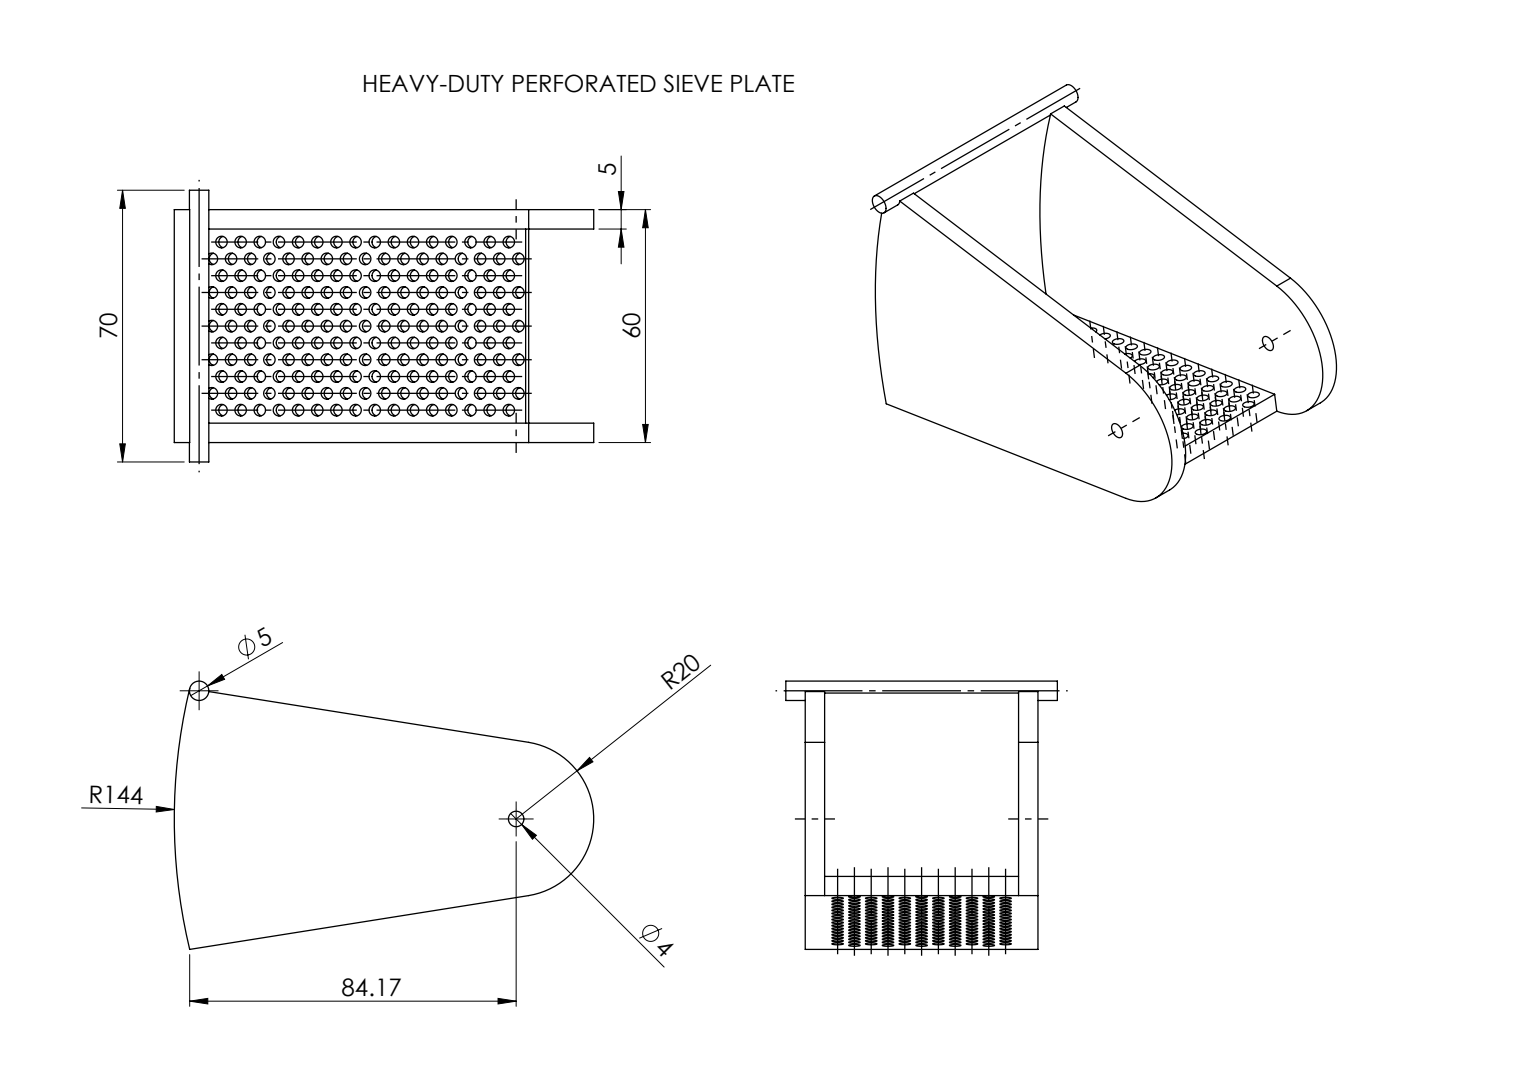
ISO-10303-21;
HEADER;
FILE_DESCRIPTION (('STEP AP214'),
    '1' );
FILE_NAME ('Heavy-Duty Perforated Sieve Plate.step',
    '2026-10-02T13:02:33',
    ( '' ),
    ( '' ),
    'SwSTEP 2.0',
    'SolidWorks 2026',
    '' );
FILE_SCHEMA (( 'AUTOMOTIVE_DESIGN' ));
ENDSEC;

DATA;
#1=DIRECTION ( 'NONE',  ( -0.9876526153536341335, -0.1566598588826327021, 0.000000000000000000 ) ) ;
#2=VERTEX_POINT ( 'NONE', #2570 ) ;
#3=LINE ( 'NONE', #7217, #14699 ) ;
#4=ADVANCED_FACE ( 'NONE', ( #13839 ), #888, .F. ) ;
#5=CARTESIAN_POINT ( 'NONE',  ( -30.20514499443620338, -82.74634522781904877, 4.330127018922213189 ) ) ;
#6=AXIS2_PLACEMENT_3D ( 'NONE', #420, #4760, #13466 ) ;
#7=DIRECTION ( 'NONE',  ( 0.000000000000000000, 0.000000000000000000, 1.000000000000000000 ) ) ;
#8=ORIENTED_EDGE ( 'NONE', *, *, #17949, .T. ) ;
#9=CIRCLE ( 'NONE', #3911, 1.500000000000000888 ) ;
#10=ORIENTED_EDGE ( 'NONE', *, *, #1419, .F. ) ;
#11=CYLINDRICAL_SURFACE ( 'NONE', #12678, 1.500000000000001554 ) ;
#14=VERTEX_POINT ( 'NONE', #10991 ) ;
#15=ORIENTED_EDGE ( 'NONE', *, *, #18047, .F. ) ;
#16=DIRECTION ( 'NONE',  ( -0.1566598588826321192, 0.9876526153536342445, 7.798540720466730171E-17 ) ) ;
#17=FACE_BOUND ( 'NONE', #10882, .T. ) ;
#18=AXIS2_PLACEMENT_3D ( 'NONE', #16860, #4970, #18101 ) ;
#19=EDGE_CURVE ( 'NONE', #12170, #1369, #18158, .T. ) ;
#20=DIRECTION ( 'NONE',  ( -0.9876526153536341335, -0.1566598588826327021, 0.000000000000000000 ) ) ;
#21=ORIENTED_EDGE ( 'NONE', *, *, #15181, .F. ) ;
#22=EDGE_CURVE ( 'NONE', #3591, #12466, #3580, .T. ) ;
#23=EDGE_CURVE ( 'NONE', #2732, #16279, #9785, .T. ) ;
#24=EDGE_CURVE ( 'NONE', #1802, #4978, #17849, .T. ) ;
#25=AXIS2_PLACEMENT_3D ( 'NONE', #11149, #18028, #14009 ) ;
#26=DIRECTION ( 'NONE',  ( -0.1566598588826321192, 0.9876526153536342445, 7.798540720466730171E-17 ) ) ;
#27=CARTESIAN_POINT ( 'NONE',  ( -56.41757431148525370, -29.19865005186066043, 17.32050807568881723 ) ) ;
#28=DIRECTION ( 'NONE',  ( -0.1566598588826321192, 0.9876526153536342445, 7.798540720466730171E-17 ) ) ;
#30=FACE_OUTER_BOUND ( 'NONE', #13183, .T. ) ;
#31=AXIS2_PLACEMENT_3D ( 'NONE', #12240, #913, #6318 ) ;
#32=DIRECTION ( 'NONE',  ( -0.1566598588826321192, 0.9876526153536342445, 7.798540720466730171E-17 ) ) ;
#33=ORIENTED_EDGE ( 'NONE', *, *, #662, .F. ) ;
#34=CIRCLE ( 'NONE', #6695, 1.500000000000000888 ) ;
#35=ORIENTED_EDGE ( 'NONE', *, *, #7081, .F. ) ;
#36=EDGE_LOOP ( 'NONE', ( #5022, #14370, #8560, #13804 ) ) ;
#37=ORIENTED_EDGE ( 'NONE', *, *, #12771, .T. ) ;
#38=ORIENTED_EDGE ( 'NONE', *, *, #14374, .T. ) ;
#41=DIRECTION ( 'NONE',  ( 0.000000000000000000, 0.000000000000000000, 1.000000000000000000 ) ) ;
#42=AXIS2_PLACEMENT_3D ( 'NONE', #5371, #11127, #3921 ) ;
#43=CARTESIAN_POINT ( 'NONE',  ( -67.24211807019732134, -88.62108993591773753, 1.443110928631665584E-14 ) ) ;
#45=AXIS2_PLACEMENT_3D ( 'NONE', #1422, #5499, #1514 ) ;
#46=CARTESIAN_POINT ( 'NONE',  ( -71.02801022084922522, -26.45362499944938506, 12.99038105676661736 ) ) ;
#48=CIRCLE ( 'NONE', #6755, 1.500000000000000000 ) ;
#50=DIRECTION ( 'NONE',  ( 0.000000000000000000, 0.000000000000000000, 1.000000000000000000 ) ) ;
#51=EDGE_CURVE ( 'NONE', #10382, #2699, #15096, .T. ) ;
#52=VECTOR ( 'NONE', #9149, 1000.000000000000000 ) ;
#53=DIRECTION ( 'NONE',  ( -0.9876526153536336894, -0.1566598588826349503, 0.000000000000000000 ) ) ;
#54=ORIENTED_EDGE ( 'NONE', *, *, #7944, .T. ) ;
#57=FACE_OUTER_BOUND ( 'NONE', #3238, .T. ) ;
#58=CARTESIAN_POINT ( 'NONE',  ( -47.32434745236211171, -22.69378838626622397, 1.926565525561698076E-14 ) ) ;
#60=CARTESIAN_POINT ( 'NONE',  ( -84.16561914167408531, -33.59999999999994458, -30.00000000000000000 ) ) ;
#61=CIRCLE ( 'NONE', #8830, 1.500000000000000444 ) ;
#62=VERTEX_POINT ( 'NONE', #27 ) ;
#63=LINE ( 'NONE', #14371, #9733 ) ;
#64=ORIENTED_EDGE ( 'NONE', *, *, #598, .T. ) ;
#66=VECTOR ( 'NONE', #7491, 1000.000000000000000 ) ;
#67=DIRECTION ( 'NONE',  ( -0.1566598588826321192, 0.9876526153536342445, 7.798540720466730171E-17 ) ) ;
#68=CARTESIAN_POINT ( 'NONE',  ( -27.28182215855319015, -24.57718421482303484, -4.330127018922181215 ) ) ;
#69=DIRECTION ( 'NONE',  ( -0.1566598588826321192, 0.9876526153536342445, 7.798540720466731404E-17 ) ) ;
#72=DIRECTION ( 'NONE',  ( -0.9876526153536336894, -0.1566598588826349503, 0.000000000000000000 ) ) ;
#73=DIRECTION ( 'NONE',  ( -0.1566598588826321192, 0.9876526153536342445, 7.798540720466731404E-17 ) ) ;
#74=DIRECTION ( 'NONE',  ( -0.1566598588826321192, 0.9876526153536342445, 7.798540720466730171E-17 ) ) ;
#75=CYLINDRICAL_SURFACE ( 'NONE', #18095, 1.500000000000001554 ) ;
#76=EDGE_LOOP ( 'NONE', ( #16554, #5977 ) ) ;
#77=CARTESIAN_POINT ( 'NONE',  ( -30.53425299135042081, -20.03057078526148516, 8.660254037844417496 ) ) ;
#78=ADVANCED_FACE ( 'NONE', ( #8643 ), #2771, .F. ) ;
#79=CARTESIAN_POINT ( 'NONE',  ( -22.79775037928398618, -81.57139628619931671, 17.32050807568881368 ) ) ;
#81=EDGE_CURVE ( 'NONE', #12067, #4830, #257, .T. ) ;
#82=DIRECTION ( 'NONE',  ( 0.000000000000000000, 0.000000000000000000, 1.000000000000000000 ) ) ;
#83=ORIENTED_EDGE ( 'NONE', *, *, #3528, .F. ) ;
#89=CYLINDRICAL_SURFACE ( 'NONE', #17046, 1.500000000000001554 ) ;
#90=DIRECTION ( 'NONE',  ( -0.1566598588826321192, 0.9876526153536342445, 7.798540720466730171E-17 ) ) ;
#91=CARTESIAN_POINT ( 'NONE',  ( -66.78792677269836986, -30.84357857012828674, 21.65063509461101887 ) ) ;
#92=CARTESIAN_POINT ( 'NONE',  ( -75.18297400320422241, -32.17518737063066681, 21.65063509461101887 ) ) ;
#93=VERTEX_POINT ( 'NONE', #10234 ) ;
#94=DIRECTION ( 'NONE',  ( -0.1566598588826321747, 0.9876526153536343555, 0.000000000000000000 ) ) ;
#95=DIRECTION ( 'NONE',  ( -0.1566598588826321747, 0.9876526153536343555, 0.000000000000000000 ) ) ;
#97=ORIENTED_EDGE ( 'NONE', *, *, #2052, .T. ) ;
#98=VERTEX_POINT ( 'NONE', #12699 ) ;
#100=AXIS2_PLACEMENT_3D ( 'NONE', #10768, #16585, #15534 ) ;
#101=EDGE_CURVE ( 'NONE', #13042, #12109, #10138, .T. ) ;
#103=ORIENTED_EDGE ( 'NONE', *, *, #6276, .F. ) ;
#104=DIRECTION ( 'NONE',  ( -0.9876526153536336894, -0.1566598588826349503, 0.000000000000000000 ) ) ;
#105=FACE_BOUND ( 'NONE', #10139, .T. ) ;
#106=ADVANCED_FACE ( 'NONE', ( #14516 ), #13086, .F. ) ;
#107=ORIENTED_EDGE ( 'NONE', *, *, #8467, .F. ) ;
#108=ORIENTED_EDGE ( 'NONE', *, *, #6919, .T. ) ;
#110=AXIS2_PLACEMENT_3D ( 'NONE', #4893, #11798, #13415 ) ;
#112=ORIENTED_EDGE ( 'NONE', *, *, #1667, .T. ) ;
#114=CARTESIAN_POINT ( 'NONE',  ( -84.16561914167411373, 33.60000000000000142, -30.00000000000000000 ) ) ;
#115=EDGE_LOOP ( 'NONE', ( #1862, #4295 ) ) ;
#117=LINE ( 'NONE', #3375, #307 ) ;
#118=EDGE_CURVE ( 'NONE', #9740, #1864, #12345, .T. ) ;
#119=FACE_OUTER_BOUND ( 'NONE', #18220, .T. ) ;
#120=FACE_BOUND ( 'NONE', #14429, .T. ) ;
#121=DIRECTION ( 'NONE',  ( -0.1566598588826321192, 0.9876526153536342445, 7.798540720466730171E-17 ) ) ;
#123=EDGE_CURVE ( 'NONE', #15608, #18110, #18554, .T. ) ;
#124=ORIENTED_EDGE ( 'NONE', *, *, #13553, .F. ) ;
#128=EDGE_CURVE ( 'NONE', #14364, #5884, #10830, .T. ) ;
#129=ORIENTED_EDGE ( 'NONE', *, *, #2912, .F. ) ;
#131=EDGE_CURVE ( 'NONE', #13266, #3195, #7839, .T. ) ;
#132=CYLINDRICAL_SURFACE ( 'NONE', #16628, 1.500000000000001554 ) ;
#133=EDGE_LOOP ( 'NONE', ( #5269, #5864 ) ) ;
#134=EDGE_CURVE ( 'NONE', #306, #3989, #4730, .T. ) ;
#135=DIRECTION ( 'NONE',  ( -0.9876526153536344665, -0.1566598588826304539, 0.000000000000000000 ) ) ;
#136=CARTESIAN_POINT ( 'NONE',  ( -54.89646037827696290, -86.66284169988483654, -12.99038105676658539 ) ) ;
#137=DIRECTION ( 'NONE',  ( -0.1566598588826321192, 0.9876526153536342445, 7.798540720466731404E-17 ) ) ;
#138=CARTESIAN_POINT ( 'NONE',  ( -48.02252708097939404, -27.86704125135830523, 8.660254037844417496 ) ) ;
#139=VERTEX_POINT ( 'NONE', #14880 ) ;
#140=ORIENTED_EDGE ( 'NONE', *, *, #2716, .F. ) ;
#143=CARTESIAN_POINT ( 'NONE',  ( -35.67686938905902849, -25.90879301532540779, -4.330127018922181215 ) ) ;
#144=CARTESIAN_POINT ( 'NONE',  ( -24.27922930231443743, -81.80638607452327449, 8.660254037844412167 ) ) ;
#145=EDGE_CURVE ( 'NONE', #1457, #13070, #13868, .T. ) ;
#146=ORIENTED_EDGE ( 'NONE', *, *, #12497, .F. ) ;
#147=DIRECTION ( 'NONE',  ( -0.1566598588826321747, 0.9876526153536343555, 0.000000000000000000 ) ) ;
#149=EDGE_CURVE ( 'NONE', #14051, #4382, #6373, .T. ) ;
#151=DIRECTION ( 'NONE',  ( -0.1566598588826321192, 0.9876526153536342445, 7.798540720466730171E-17 ) ) ;
#153=LINE ( 'NONE', #5658, #5168 ) ;
#154=CARTESIAN_POINT ( 'NONE',  ( -70.24471092643608472, -31.39188807621751209, 21.65063509461101887 ) ) ;
#155=SHAPE_REPRESENTATION_RELATIONSHIP ( 'NONE' , 'NONE' ,  #6739, #1868 ) ;
#157=CARTESIAN_POINT ( 'NONE',  ( -33.00338452973448966, -20.42222043246806251, 4.330127018922218518 ) ) ;
#158=DIRECTION ( 'NONE',  ( -0.1566598588826321192, 0.9876526153536342445, 7.798540720466730171E-17 ) ) ;
#159=DIRECTION ( 'NONE',  ( -0.1566598588826321192, 0.9876526153536342445, 7.798540720466730171E-17 ) ) ;
#160=CARTESIAN_POINT ( 'NONE',  ( -18.35331361019266794, -80.86642692122747178, 4.330127018922213189 ) ) ;
#161=ORIENTED_EDGE ( 'NONE', *, *, #2086, .F. ) ;
#163=CARTESIAN_POINT ( 'NONE',  ( -6.047290928450125946, -21.20899724884646531, -21.65063509461098334 ) ) ;
#164=ORIENTED_EDGE ( 'NONE', *, *, #5902, .T. ) ;
#166=CARTESIAN_POINT ( 'NONE',  ( -39.91695283720987675, -21.51883944464648479, -4.330127018922180326 ) ) ;
#167=EDGE_LOOP ( 'NONE', ( #17757, #5769 ) ) ;
#168=CARTESIAN_POINT ( 'NONE',  ( -16.91146969734005268, -22.93225569655540141, -8.660254037844380193 ) ) ;
#169=EDGE_CURVE ( 'NONE', #4575, #3501, #2377, .T. ) ;
#170=DIRECTION ( 'NONE',  ( -0.9876526153536336894, -0.1566598588826349503, 0.000000000000000000 ) ) ;
#172=DIRECTION ( 'NONE',  ( -0.1566598588826321192, 0.9876526153536342445, 7.798540720466730171E-17 ) ) ;
#173=CARTESIAN_POINT ( 'NONE',  ( -58.88670584986932255, -29.59029969906724133, 12.99038105676661736 ) ) ;
#174=EDGE_CURVE ( 'NONE', #9818, #7902, #192, .T. ) ;
#175=LINE ( 'NONE', #6157, #13878 ) ;
#176=AXIS2_PLACEMENT_3D ( 'NONE', #2016, #3423, #9416 ) ;
#177=ORIENTED_EDGE ( 'NONE', *, *, #17607, .F. ) ;
#178=CARTESIAN_POINT ( 'NONE',  ( -22.79775037928398618, -81.57139628619930249, -17.32050807568878525 ) ) ;
#179=CARTESIAN_POINT ( 'NONE',  ( -34.19539046602857724, -25.67380322700145356, 12.99038105676661736 ) ) ;
#182=CARTESIAN_POINT ( 'NONE',  ( -60.36818477289978091, -29.82528948739120267, -12.99038105676658006 ) ) ;
#183=CIRCLE ( 'NONE', #2605, 1.500000000000000888 ) ;
#184=ORIENTED_EDGE ( 'NONE', *, *, #555, .T. ) ;
#185=ORIENTED_EDGE ( 'NONE', *, *, #890, .F. ) ;
#186=CARTESIAN_POINT ( 'NONE',  ( -68.55887868246516348, -26.06197535224280770, 17.32050807568882078 ) ) ;
#187=CARTESIAN_POINT ( 'NONE',  ( -37.94164760650264867, -21.20551972688121012, -21.65063509461098334 ) ) ;
#188=EDGE_LOOP ( 'NONE', ( #13607, #15627 ) ) ;
#189=CARTESIAN_POINT ( 'NONE',  ( -49.01017969633304006, -28.02370111024093191, -12.99038105676658006 ) ) ;
#191=EDGE_CURVE ( 'NONE', #13070, #8810, #6083, .T. ) ;
#192=LINE ( 'NONE', #17673, #12969 ) ;
#193=EDGE_LOOP ( 'NONE', ( #12370, #7151, #5297, #6845 ) ) ;
#195=ORIENTED_EDGE ( 'NONE', *, *, #18603, .T. ) ;
#197=AXIS2_PLACEMENT_3D ( 'NONE', #13789, #13899, #10956 ) ;
#200=DIRECTION ( 'NONE',  ( -0.1566598588826321192, 0.9876526153536342445, 7.798540720466731404E-17 ) ) ;
#201=ADVANCED_FACE ( 'NONE', ( #1648 ), #132, .F. ) ;
#202=VERTEX_POINT ( 'NONE', #5909 ) ;
#203=ORIENTED_EDGE ( 'NONE', *, *, #2611, .T. ) ;
#204=ORIENTED_EDGE ( 'NONE', *, *, #16861, .F. ) ;
#205=ORIENTED_EDGE ( 'NONE', *, *, #601, .T. ) ;
#206=DIRECTION ( 'NONE',  ( -0.1566598588826321192, 0.9876526153536342445, 7.798540720466731404E-17 ) ) ;
#207=AXIS2_PLACEMENT_3D ( 'NONE', #17977, #18347, #1736 ) ;
#208=ORIENTED_EDGE ( 'NONE', *, *, #14608, .T. ) ;
#209=FACE_BOUND ( 'NONE', #76, .T. ) ;
#210=CARTESIAN_POINT ( 'NONE',  ( 10.28861223506262412, -76.32329101363113466, 8.660254037844406838 ) ) ;
#211=VERTEX_POINT ( 'NONE', #5994 ) ;
#213=EDGE_LOOP ( 'NONE', ( #813, #9222, #12211, #16308 ) ) ;
#214=CIRCLE ( 'NONE', #11085, 1.500000000000000888 ) ;
#216=CIRCLE ( 'NONE', #4738, 1.500000000000000444 ) ;
#217=DIRECTION ( 'NONE',  ( -0.9876526153536344665, -0.1566598588826304539, 0.000000000000000000 ) ) ;
#218=CIRCLE ( 'NONE', #4461, 1.499999999999999556 ) ;
#219=EDGE_CURVE ( 'NONE', #16637, #6756, #7426, .T. ) ;
#221=CARTESIAN_POINT ( 'NONE',  ( -18.39294862037050393, -23.16724548487935564, 1.869203119972154228E-14 ) ) ;
#222=CARTESIAN_POINT ( 'NONE',  ( -10.98555400521827607, -21.99229654325962002, 12.99038105676661381 ) ) ;
#223=DIRECTION ( 'NONE',  ( -0.000000000000000000, -0.000000000000000000, -1.000000000000000000 ) ) ;
#224=EDGE_CURVE ( 'NONE', #15083, #7553, #10560, .T. ) ;
#226=ORIENTED_EDGE ( 'NONE', *, *, #15016, .F. ) ;
#227=VERTEX_POINT ( 'NONE', #8930 ) ;
#228=CARTESIAN_POINT ( 'NONE',  ( -19.34096622554629263, -81.02308678011010556, 1.424741226644455312E-14 ) ) ;
#231=LINE ( 'NONE', #17611, #15362 ) ;
#232=ORIENTED_EDGE ( 'NONE', *, *, #13411, .F. ) ;
#234=ORIENTED_EDGE ( 'NONE', *, *, #16412, .F. ) ;
#235=CARTESIAN_POINT ( 'NONE',  ( -9.299721761247353058, -16.66238381928489787, -17.32050807568878170 ) ) ;
#236=FACE_BOUND ( 'NONE', #6125, .T. ) ;
#238=CARTESIAN_POINT ( 'NONE',  ( -64.77298653181324539, -88.22944028871116018, 21.65063509461101532 ) ) ;
#239=EDGE_CURVE ( 'NONE', #10470, #12526, #9677, .T. ) ;
#240=CIRCLE ( 'NONE', #6612, 1.500000000000000444 ) ;
#242=EDGE_CURVE ( 'NONE', #4960, #1643, #5109, .T. ) ;
#243=DIRECTION ( 'NONE',  ( -0.9876526153536336894, -0.1566598588826349503, 0.000000000000000000 ) ) ;
#244=CARTESIAN_POINT ( 'NONE',  ( -14.40270314877813895, -80.23978748569693664, -17.32050807568878525 ) ) ;
#247=EDGE_LOOP ( 'NONE', ( #10607, #2910 ) ) ;
#248=EDGE_LOOP ( 'NONE', ( #11901, #15407, #18357, #803 ) ) ;
#249=CARTESIAN_POINT ( 'NONE',  ( -41.39843176024032800, -21.75382923297043192, 4.330127018922218518 ) ) ;
#250=CIRCLE ( 'NONE', #2017, 1.500000000000000444 ) ;
#251=AXIS2_PLACEMENT_3D ( 'NONE', #14278, #17128, #4490 ) ;
#252=ORIENTED_EDGE ( 'NONE', *, *, #3818, .T. ) ;
#253=VECTOR ( 'NONE', #1467, 1000.000000000000000 ) ;
#254=EDGE_LOOP ( 'NONE', ( #5319, #8500, #14701, #2198 ) ) ;
#255=ORIENTED_EDGE ( 'NONE', *, *, #6970, .T. ) ;
#257=CIRCLE ( 'NONE', #7250, 1.499999999999999556 ) ;
#260=AXIS2_PLACEMENT_3D ( 'NONE', #1453, #14527, #297 ) ;
#261=CARTESIAN_POINT ( 'NONE',  ( -36.62488699423482785, -83.76463431055616127, -21.65063509461098690 ) ) ;
#262=CARTESIAN_POINT ( 'NONE',  ( -41.39843176024032800, -21.75382923297042836, -4.330127018922180326 ) ) ;
#264=DIRECTION ( 'NONE',  ( -0.9876526153536336894, -0.1566598588826349503, 0.000000000000000000 ) ) ;
#265=CARTESIAN_POINT ( 'NONE',  ( -26.78799585087635649, -24.49885428538171794, -8.660254037844380193 ) ) ;
#267=ORIENTED_EDGE ( 'NONE', *, *, #13623, .F. ) ;
#268=DIRECTION ( 'NONE',  ( -0.9876526153536336894, -0.1566598588826349503, 0.000000000000000000 ) ) ;
#269=EDGE_LOOP ( 'NONE', ( #9815, #12862, #15948, #5626 ) ) ;
#270=EDGE_CURVE ( 'NONE', #17286, #16790, #6357, .T. ) ;
#271=AXIS2_PLACEMENT_3D ( 'NONE', #15102, #6588, #11007 ) ;
#272=VERTEX_POINT ( 'NONE', #11653 ) ;
#274=CARTESIAN_POINT ( 'NONE',  ( -6.047290928450125946, -21.20899724884646531, 21.65063509461101177 ) ) ;
#275=VECTOR ( 'NONE', #8347, 1000.000000000000000 ) ;
#277=ORIENTED_EDGE ( 'NONE', *, *, #10855, .F. ) ;
#278=FACE_OUTER_BOUND ( 'NONE', #17914, .T. ) ;
#279=CIRCLE ( 'NONE', #11460, 1.500000000000000444 ) ;
#280=EDGE_CURVE ( 'NONE', #14450, #6414, #16167, .T. ) ;
#281=VECTOR ( 'NONE', #15110, 1000.000000000000000 ) ;
#282=CIRCLE ( 'NONE', #10852, 1.500000000000000000 ) ;
#283=DIRECTION ( 'NONE',  ( -0.9876526153536341335, -0.1566598588826327021, 0.000000000000000000 ) ) ;
#285=CARTESIAN_POINT ( 'NONE',  ( -13.25033222266188560, -17.28902325481542235, 4.330127018922214965 ) ) ;
#287=AXIS2_PLACEMENT_3D ( 'NONE', #9251, #13887, #9450 ) ;
#291=FACE_BOUND ( 'NONE', #9868, .T. ) ;
#292=AXIS2_PLACEMENT_3D ( 'NONE', #3529, #12534, #16843 ) ;
#295=DIRECTION ( 'NONE',  ( -0.9876526153536341335, -0.1566598588826327021, 0.000000000000000000 ) ) ;
#296=VECTOR ( 'NONE', #9069, 1000.000000000000000 ) ;
#297=DIRECTION ( 'NONE',  ( 0.000000000000000000, 0.000000000000000000, 1.000000000000000000 ) ) ;
#298=ORIENTED_EDGE ( 'NONE', *, *, #1505, .F. ) ;
#299=VERTEX_POINT ( 'NONE', #6020 ) ;
#300=ORIENTED_EDGE ( 'NONE', *, *, #13362, .F. ) ;
#301=AXIS2_PLACEMENT_3D ( 'NONE', #1034, #11223, #5560 ) ;
#302=ORIENTED_EDGE ( 'NONE', *, *, #6850, .F. ) ;
#303=DIRECTION ( 'NONE',  ( -0.9876526153536336894, -0.1566598588826349503, 0.000000000000000000 ) ) ;
#306=VERTEX_POINT ( 'NONE', #6126 ) ;
#307=VECTOR ( 'NONE', #16481, 1000.000000000000000 ) ;
#308=FACE_BOUND ( 'NONE', #13049, .T. ) ;
#309=DIRECTION ( 'NONE',  ( -0.9876526153536336894, -0.1566598588826349503, 0.000000000000000000 ) ) ;
#310=VECTOR ( 'NONE', #14810, 1000.000000000000000 ) ;
#311=VERTEX_POINT ( 'NONE', #14829 ) ;
#312=CARTESIAN_POINT ( 'NONE',  ( -23.33121169713865584, -23.95054477929251036, -8.660254037844380193 ) ) ;
#313=VECTOR ( 'NONE', #867, 1000.000000000000000 ) ;
#314=EDGE_LOOP ( 'NONE', ( #6630, #11469 ) ) ;
#315=EDGE_CURVE ( 'NONE', #5884, #5893, #1848, .T. ) ;
#316=EDGE_CURVE ( 'NONE', #12986, #12973, #2391, .T. ) ;
#317=EDGE_LOOP ( 'NONE', ( #16039, #7700, #562, #13733 ) ) ;
#318=AXIS2_PLACEMENT_3D ( 'NONE', #5866, #8616, #8694 ) ;
#319=DIRECTION ( 'NONE',  ( 0.000000000000000000, 0.000000000000000000, 1.000000000000000000 ) ) ;
#320=DIRECTION ( 'NONE',  ( -0.1566598588826321192, 0.9876526153536342445, 7.798540720466730171E-17 ) ) ;
#321=AXIS2_PLACEMENT_3D ( 'NONE', #1598, #12854, #13040 ) ;
#322=CARTESIAN_POINT ( 'NONE',  ( -13.45468554360235203, -22.38394619046619383, 1.869203119972154228E-14 ) ) ;
#323=DIRECTION ( 'NONE',  ( -0.1566598588826321192, 0.9876526153536342445, 7.798540720466731404E-17 ) ) ;
#324=CARTESIAN_POINT ( 'NONE',  ( -6.995308533625909320, -79.06483854407721878, 21.65063509461100821 ) ) ;
#325=LINE ( 'NONE', #9139, #5689 ) ;
#327=ORIENTED_EDGE ( 'NONE', *, *, #12450, .F. ) ;
#328=LINE ( 'NONE', #4668, #9322 ) ;
#329=AXIS2_PLACEMENT_3D ( 'NONE', #4692, #16469, #16269 ) ;
#330=DIRECTION ( 'NONE',  ( -0.1566598588826321192, 0.9876526153536342445, 7.798540720466730171E-17 ) ) ;
#331=DIRECTION ( 'NONE',  ( -0.1566598588826321192, 0.9876526153536342445, 7.798540720466730171E-17 ) ) ;
#332=CIRCLE ( 'NONE', #3341, 1.500000000000000888 ) ;
#333=ADVANCED_FACE ( 'NONE', ( #10729 ), #15383, .F. ) ;
#334=VERTEX_POINT ( 'NONE', #16930 ) ;
#335=CARTESIAN_POINT ( 'NONE',  ( -75.18297400320422241, -32.17518737063066681, 21.65063509461101887 ) ) ;
#336=CIRCLE ( 'NONE', #16374, 1.500000000000000888 ) ;
#337=AXIS2_PLACEMENT_3D ( 'NONE', #9442, #15216, #13774 ) ;
#338=FACE_BOUND ( 'NONE', #5848, .T. ) ;
#339=EDGE_CURVE ( 'NONE', #7418, #9571, #3618, .T. ) ;
#340=DIRECTION ( 'NONE',  ( 0.000000000000000000, 0.000000000000000000, 1.000000000000000000 ) ) ;
#341=CIRCLE ( 'NONE', #12123, 1.500000000000001332 ) ;
#342=DIRECTION ( 'NONE',  ( -0.1566598588826321192, 0.9876526153536342445, 7.798540720466731404E-17 ) ) ;
#343=DIRECTION ( 'NONE',  ( -0.1566598588826321192, 0.9876526153536342445, 7.798540720466730171E-17 ) ) ;
#344=VERTEX_POINT ( 'NONE', #5255 ) ;
#345=DIRECTION ( 'NONE',  ( -0.1566598588826321747, 0.9876526153536343555, 0.000000000000000000 ) ) ;
#346=CARTESIAN_POINT ( 'NONE',  ( -45.34904222165486942, -22.38046866850094929, -17.32050807568878170 ) ) ;
#349=FACE_OUTER_BOUND ( 'NONE', #8068, .T. ) ;
#350=LINE ( 'NONE', #15811, #2031 ) ;
#351=EDGE_LOOP ( 'NONE', ( #7291, #2729, #13644, #16148 ) ) ;
#352=CARTESIAN_POINT ( 'NONE',  ( -45.01993422474065198, -85.09624311105852712, 4.330127018922213189 ) ) ;
#353=EDGE_CURVE ( 'NONE', #8550, #12053, #18503, .T. ) ;
#356=VERTEX_POINT ( 'NONE', #16529 ) ;
#357=EDGE_CURVE ( 'NONE', #4379, #18393, #1509, .T. ) ;
#358=EDGE_CURVE ( 'NONE', #1477, #15259, #8155, .T. ) ;
#360=EDGE_LOOP ( 'NONE', ( #2874, #17765 ) ) ;
#362=EDGE_CURVE ( 'NONE', #1820, #10566, #9051, .T. ) ;
#363=AXIS2_PLACEMENT_3D ( 'NONE', #14211, #2358, #12673 ) ;
#365=DIRECTION ( 'NONE',  ( -0.1566598588826321192, 0.9876526153536342445, 7.798540720466730171E-17 ) ) ;
#366=ORIENTED_EDGE ( 'NONE', *, *, #8931, .T. ) ;
#367=CARTESIAN_POINT ( 'NONE',  ( -48.80582637539254875, -22.92877817459017464, 17.32050807568882078 ) ) ;
#368=CARTESIAN_POINT ( 'NONE',  ( -66.25446545484369665, -88.46443007703511796, -12.99038105676658539 ) ) ;
#369=DIRECTION ( 'NONE',  ( -0.9876526153536336894, -0.1566598588826349503, 0.000000000000000000 ) ) ;
#370=VERTEX_POINT ( 'NONE', #11385 ) ;
#371=AXIS2_PLACEMENT_3D ( 'NONE', #10848, #743, #7570 ) ;
#372=CARTESIAN_POINT ( 'NONE',  ( -46.50141314777110324, -85.33123289938248490, 4.330127018922213189 ) ) ;
#375=AXIS2_PLACEMENT_3D ( 'NONE', #5395, #11058, #12194 ) ;
#376=DIRECTION ( 'NONE',  ( -0.9876526153536341335, -0.1566598588826327021, 0.000000000000000000 ) ) ;
#377=EDGE_LOOP ( 'NONE', ( #5700, #15642 ) ) ;
#378=DIRECTION ( 'NONE',  ( -0.9876526153536341335, -0.1566598588826327021, 0.000000000000000000 ) ) ;
#382=DIRECTION ( 'NONE',  ( 0.000000000000000000, 0.000000000000000000, 1.000000000000000000 ) ) ;
#383=ORIENTED_EDGE ( 'NONE', *, *, #18100, .F. ) ;
#384=VERTEX_POINT ( 'NONE', #4086 ) ;
#385=EDGE_LOOP ( 'NONE', ( #16397, #10275 ) ) ;
#386=DIRECTION ( 'NONE',  ( -0.9876526153536341335, -0.1566598588826327021, 0.000000000000000000 ) ) ;
#389=ORIENTED_EDGE ( 'NONE', *, *, #13835, .T. ) ;
#390=CARTESIAN_POINT ( 'NONE',  ( -48.97054468615517919, -85.72288254658904805, 8.660254037844412167 ) ) ;
#391=ORIENTED_EDGE ( 'NONE', *, *, #358, .T. ) ;
#392=CYLINDRICAL_SURFACE ( 'NONE', #15221, 1.500000000000001554 ) ;
#393=ORIENTED_EDGE ( 'NONE', *, *, #4749, .F. ) ;
#394=EDGE_CURVE ( 'NONE', #17063, #537, #14514, .T. ) ;
#396=ORIENTED_EDGE ( 'NONE', *, *, #516, .F. ) ;
#397=ORIENTED_EDGE ( 'NONE', *, *, #14939, .F. ) ;
#398=AXIS2_PLACEMENT_3D ( 'NONE', #6831, #12574, #2548 ) ;
#399=DIRECTION ( 'NONE',  ( -0.9876526153536336894, -0.1566598588826350336, 0.000000000000000000 ) ) ;
#400=FACE_OUTER_BOUND ( 'NONE', #2830, .T. ) ;
#401=ORIENTED_EDGE ( 'NONE', *, *, #13050, .T. ) ;
#402=ORIENTED_EDGE ( 'NONE', *, *, #11892, .F. ) ;
#403=VERTEX_POINT ( 'NONE', #17028 ) ;
#404=ORIENTED_EDGE ( 'NONE', *, *, #8014, .T. ) ;
#405=VERTEX_POINT ( 'NONE', #2589 ) ;
#406=ORIENTED_EDGE ( 'NONE', *, *, #492, .F. ) ;
#407=CARTESIAN_POINT ( 'NONE',  ( -21.81009776393036503, -81.41473642731666871, -21.65063509461098690 ) ) ;
#408=ORIENTED_EDGE ( 'NONE', *, *, #6164, .F. ) ;
#409=ORIENTED_EDGE ( 'NONE', *, *, #15155, .F. ) ;
#410=FACE_BOUND ( 'NONE', #1885, .T. ) ;
#412=CARTESIAN_POINT ( 'NONE',  ( -44.03228160938703439, -84.93958325217590755, 8.660254037844412167 ) ) ;
#413=ORIENTED_EDGE ( 'NONE', *, *, #12861, .T. ) ;
#414=ADVANCED_FACE ( 'NONE', ( #17211 ), #2684, .T. ) ;
#415=ORIENTED_EDGE ( 'NONE', *, *, #13647, .F. ) ;
#416=FACE_BOUND ( 'NONE', #8311, .T. ) ;
#418=ADVANCED_FACE ( 'NONE', ( #10070 ), #1375, .F. ) ;
#419=CARTESIAN_POINT ( 'NONE',  ( -46.50141314777111745, -85.33123289938247069, -21.65063509461098690 ) ) ;
#420=CARTESIAN_POINT ( 'NONE',  ( -75.18297400320422241, -32.17518737063066681, 4.330127018922217630 ) ) ;
#422=DIRECTION ( 'NONE',  ( -0.1566598588826321192, 0.9876526153536342445, 7.798540720466731404E-17 ) ) ;
#423=DIRECTION ( 'NONE',  ( -0.9876526153536336894, -0.1566598588826349503, 0.000000000000000000 ) ) ;
#424=ORIENTED_EDGE ( 'NONE', *, *, #224, .F. ) ;
#425=EDGE_LOOP ( 'NONE', ( #6614, #11556 ) ) ;
#427=CARTESIAN_POINT ( 'NONE',  ( -51.97313754239394257, -28.49368068688882971, -21.65063509461098334 ) ) ;
#428=DIRECTION ( 'NONE',  ( -0.1566598588826321192, 0.9876526153536342445, 7.798540720466730171E-17 ) ) ;
#431=DIRECTION ( 'NONE',  ( -0.1566598588826321192, 0.9876526153536342445, 7.798540720466730171E-17 ) ) ;
#432=DIRECTION ( 'NONE',  ( -0.1566598588826321192, 0.9876526153536342445, 7.798540720466731404E-17 ) ) ;
#433=FACE_OUTER_BOUND ( 'NONE', #8720, .T. ) ;
#434=EDGE_CURVE ( 'NONE', #14223, #211, #7251, .T. ) ;
#435=CARTESIAN_POINT ( 'NONE',  ( -1.109027851681966492, -20.42569795443330349, 12.99038105676661026 ) ) ;
#436=FACE_OUTER_BOUND ( 'NONE', #14679, .T. ) ;
#437=CARTESIAN_POINT ( 'NONE',  ( -38.10636591726525069, -83.99962409888011905, 21.65063509461101532 ) ) ;
#439=ORIENTED_EDGE ( 'NONE', *, *, #9830, .F. ) ;
#441=DIRECTION ( 'NONE',  ( -0.1566598588826321192, 0.9876526153536342445, 7.798540720466730171E-17 ) ) ;
#442=VERTEX_POINT ( 'NONE', #9802 ) ;
#443=ORIENTED_EDGE ( 'NONE', *, *, #4057, .T. ) ;
#444=EDGE_CURVE ( 'NONE', #18320, #13724, #15774, .T. ) ;
#445=ORIENTED_EDGE ( 'NONE', *, *, #17707, .F. ) ;
#446=CIRCLE ( 'NONE', #10419, 1.500000000000000444 ) ;
#448=ORIENTED_EDGE ( 'NONE', *, *, #11230, .F. ) ;
#449=DIRECTION ( 'NONE',  ( -0.1566598588826321192, 0.9876526153536342445, 7.798540720466730171E-17 ) ) ;
#450=VERTEX_POINT ( 'NONE', #8374 ) ;
#451=DIRECTION ( 'NONE',  ( -0.1566598588826321747, 0.9876526153536343555, 0.000000000000000000 ) ) ;
#452=DIRECTION ( 'NONE',  ( -0.1566598588826321747, 0.9876526153536343555, 0.000000000000000000 ) ) ;
#453=DIRECTION ( 'NONE',  ( -0.9876526153536341335, -0.1566598588826327021, 0.000000000000000000 ) ) ;
#455=CARTESIAN_POINT ( 'NONE',  ( -37.61253960958843834, -83.92129416943879505, 1.443110928631665584E-14 ) ) ;
#456=ORIENTED_EDGE ( 'NONE', *, *, #5446, .T. ) ;
#458=FACE_BOUND ( 'NONE', #12232, .T. ) ;
#459=ADVANCED_FACE ( 'NONE', ( #14152 ), #2791, .F. ) ;
#460=DIRECTION ( 'NONE',  ( -0.1566598588826321192, 0.9876526153536342445, 7.798540720466730171E-17 ) ) ;
#461=ORIENTED_EDGE ( 'NONE', *, *, #12663, .T. ) ;
#462=DIRECTION ( 'NONE',  ( -0.1566598588826321192, 0.9876526153536342445, 7.798540720466730171E-17 ) ) ;
#463=EDGE_CURVE ( 'NONE', #931, #3364, #13273, .T. ) ;
#464=VECTOR ( 'NONE', #8302, 1000.000000000000000 ) ;
#465=FACE_OUTER_BOUND ( 'NONE', #17810, .T. ) ;
#466=ORIENTED_EDGE ( 'NONE', *, *, #9742, .F. ) ;
#467=EDGE_CURVE ( 'NONE', #9397, #7759, #14260, .T. ) ;
#469=EDGE_LOOP ( 'NONE', ( #9333, #3211, #5541, #13498 ) ) ;
#470=ORIENTED_EDGE ( 'NONE', *, *, #17168, .T. ) ;
#471=ORIENTED_EDGE ( 'NONE', *, *, #13823, .T. ) ;
#472=CARTESIAN_POINT ( 'NONE',  ( -38.10636591726526490, -83.99962409888010484, -12.99038105676658539 ) ) ;
#473=CYLINDRICAL_SURFACE ( 'NONE', #18582, 1.500000000000001554 ) ;
#474=ORIENTED_EDGE ( 'NONE', *, *, #16472, .T. ) ;
#475=CYLINDRICAL_SURFACE ( 'NONE', #1700, 1.500000000000000888 ) ;
#477=AXIS2_PLACEMENT_3D ( 'NONE', #13662, #13565, #10447 ) ;
#478=DIRECTION ( 'NONE',  ( 0.000000000000000000, 0.000000000000000000, 1.000000000000000000 ) ) ;
#483=FACE_BOUND ( 'NONE', #13486, .T. ) ;
#484=EDGE_CURVE ( 'NONE', #14364, #13704, #1564, .T. ) ;
#485=ORIENTED_EDGE ( 'NONE', *, *, #9618, .T. ) ;
#486=VECTOR ( 'NONE', #9487, 1000.000000000000000 ) ;
#487=DIRECTION ( 'NONE',  ( -0.9876526153536341335, -0.1566598588826327021, 0.000000000000000000 ) ) ;
#488=DIRECTION ( 'NONE',  ( -0.9876526153536341335, -0.1566598588826327021, 0.000000000000000000 ) ) ;
#489=EDGE_CURVE ( 'NONE', #18416, #1139, #6043, .T. ) ;
#491=VERTEX_POINT ( 'NONE', #2863 ) ;
#492=EDGE_CURVE ( 'NONE', #15556, #14764, #2100, .T. ) ;
#493=EDGE_LOOP ( 'NONE', ( #4032, #9284, #18031, #15546 ) ) ;
#494=ORIENTED_EDGE ( 'NONE', *, *, #2458, .T. ) ;
#495=VERTEX_POINT ( 'NONE', #13004 ) ;
#497=EDGE_LOOP ( 'NONE', ( #2948, #10572, #17851, #2071 ) ) ;
#498=FACE_BOUND ( 'NONE', #17308, .T. ) ;
#499=AXIS2_PLACEMENT_3D ( 'NONE', #13270, #3318, #9014 ) ;
#500=CYLINDRICAL_SURFACE ( 'NONE', #18608, 1.500000000000001554 ) ;
#501=ORIENTED_EDGE ( 'NONE', *, *, #11049, .F. ) ;
#502=VECTOR ( 'NONE', #15322, 1000.000000000000000 ) ;
#503=ORIENTED_EDGE ( 'NONE', *, *, #3380, .F. ) ;
#504=DIRECTION ( 'NONE',  ( -0.9876526153536341335, -0.1566598588826327021, 0.000000000000000000 ) ) ;
#505=ORIENTED_EDGE ( 'NONE', *, *, #6048, .T. ) ;
#506=LINE ( 'NONE', #700, #9084 ) ;
#507=CARTESIAN_POINT ( 'NONE',  ( -42.38608437559395270, -21.91048909185306925, 8.660254037844417496 ) ) ;
#509=DIRECTION ( 'NONE',  ( 0.000000000000000000, 0.000000000000000000, 1.000000000000000000 ) ) ;
#510=ORIENTED_EDGE ( 'NONE', *, *, #9686, .F. ) ;
#511=EDGE_LOOP ( 'NONE', ( #3706, #485 ) ) ;
#513=AXIS2_PLACEMENT_3D ( 'NONE', #14412, #1535, #9778 ) ;
#515=DIRECTION ( 'NONE',  ( -0.9876526153536336894, -0.1566598588826349503, 0.000000000000000000 ) ) ;
#516=EDGE_CURVE ( 'NONE', #370, #16376, #2953, .T. ) ;
#517=DIRECTION ( 'NONE',  ( 0.000000000000000000, 0.000000000000000000, 1.000000000000000000 ) ) ;
#519=EDGE_CURVE ( 'NONE', #14468, #5881, #4054, .T. ) ;
#520=VECTOR ( 'NONE', #6791, 1000.000000000000000 ) ;
#521=ORIENTED_EDGE ( 'NONE', *, *, #3170, .T. ) ;
#523=AXIS2_PLACEMENT_3D ( 'NONE', #1578, #2969, #8674 ) ;
#524=DIRECTION ( 'NONE',  ( -0.1566598588826321747, 0.9876526153536343555, 0.000000000000000000 ) ) ;
#525=ORIENTED_EDGE ( 'NONE', *, *, #14996, .F. ) ;
#526=EDGE_CURVE ( 'NONE', #6605, #14798, #15112, .T. ) ;
#527=CIRCLE ( 'NONE', #10191, 1.500000000000000888 ) ;
#529=DIRECTION ( 'NONE',  ( -0.1566598588826321192, 0.9876526153536342445, 7.798540720466731404E-17 ) ) ;
#531=EDGE_LOOP ( 'NONE', ( #10532, #13578 ) ) ;
#532=DIRECTION ( 'NONE',  ( -0.1566598588826321192, 0.9876526153536342445, 7.798540720466731404E-17 ) ) ;
#533=DIRECTION ( 'NONE',  ( -0.9876526153536341335, -0.1566598588826327021, 0.000000000000000000 ) ) ;
#535=VECTOR ( 'NONE', #11000, 1000.000000000000000 ) ;
#537=VERTEX_POINT ( 'NONE', #4535 ) ;
#538=DIRECTION ( 'NONE',  ( -0.1566598588826321192, 0.9876526153536342445, 7.798540720466731404E-17 ) ) ;
#539=ORIENTED_EDGE ( 'NONE', *, *, #13629, .T. ) ;
#540=AXIS2_PLACEMENT_3D ( 'NONE', #14197, #7021, #18420 ) ;
#541=ORIENTED_EDGE ( 'NONE', *, *, #18462, .T. ) ;
#542=ORIENTED_EDGE ( 'NONE', *, *, #10730, .T. ) ;
#543=EDGE_CURVE ( 'NONE', #4382, #4160, #12054, .T. ) ;
#544=DIRECTION ( 'NONE',  ( -0.9876526153536344665, -0.1566598588826304539, 0.000000000000000000 ) ) ;
#545=CARTESIAN_POINT ( 'NONE',  ( -57.20087360589841552, -24.26038697509253694, -8.660254037844380193 ) ) ;
#546=AXIS2_PLACEMENT_3D ( 'NONE', #4997, #10776, #10699 ) ;
#547=DIRECTION ( 'NONE',  ( -0.1566598588826321192, 0.9876526153536342445, 7.798540720466730171E-17 ) ) ;
#548=DIRECTION ( 'NONE',  ( -0.1566598588826321192, 0.9876526153536342445, 7.798540720466731404E-17 ) ) ;
#549=ORIENTED_EDGE ( 'NONE', *, *, #6994, .F. ) ;
#550=CARTESIAN_POINT ( 'NONE',  ( -26.74836084069850983, -82.19803572172985184, 21.65063509461101532 ) ) ;
#553=AXIS2_PLACEMENT_3D ( 'NONE', #8026, #3657, #13790 ) ;
#554=DIRECTION ( 'NONE',  ( -0.1566598588826321192, 0.9876526153536342445, 7.798540720466730171E-17 ) ) ;
#555=EDGE_CURVE ( 'NONE', #8251, #1903, #12013, .T. ) ;
#556=CARTESIAN_POINT ( 'NONE',  ( -16.87183468716221313, -80.63143713290354242, 12.99038105676661203 ) ) ;
#557=AXIS2_PLACEMENT_3D ( 'NONE', #12003, #12293, #13716 ) ;
#560=CARTESIAN_POINT ( 'NONE',  ( -43.86756329862440396, -22.14547888017701283, 8.660254037844417496 ) ) ;
#561=CARTESIAN_POINT ( 'NONE',  ( -42.55080268635658314, -84.70459346385194976, 1.443110928631665584E-14 ) ) ;
#562=ORIENTED_EDGE ( 'NONE', *, *, #1186, .T. ) ;
#565=ORIENTED_EDGE ( 'NONE', *, *, #12861, .F. ) ;
#566=EDGE_LOOP ( 'NONE', ( #4430, #255 ) ) ;
#567=DIRECTION ( 'NONE',  ( -0.1566598588826321747, 0.9876526153536343555, 0.000000000000000000 ) ) ;
#568=ADVANCED_FACE ( 'NONE', ( #7048 ), #12876, .F. ) ;
#570=CARTESIAN_POINT ( 'NONE',  ( -73.70149508017377116, -31.94019758230671258, -4.330127018922181215 ) ) ;
#571=VECTOR ( 'NONE', #10120, 1000.000000000000000 ) ;
#572=EDGE_CURVE ( 'NONE', #12438, #2916, #15328, .T. ) ;
#573=ORIENTED_EDGE ( 'NONE', *, *, #1192, .T. ) ;
#576=ORIENTED_EDGE ( 'NONE', *, *, #17660, .F. ) ;
#577=CARTESIAN_POINT ( 'NONE',  ( -50.49165861936347000, -28.25869089856487903, 21.65063509461101887 ) ) ;
#578=CYLINDRICAL_SURFACE ( 'NONE', #1583, 1.500000000000001554 ) ;
#579=ADVANCED_FACE ( 'NONE', ( #13708 ), #5677, .F. ) ;
#581=DIRECTION ( 'NONE',  ( -0.1566598588826321747, 0.9876526153536343555, 0.000000000000000000 ) ) ;
#583=CARTESIAN_POINT ( 'NONE',  ( -6.830590222863280658, -16.27073417207831696, 4.330127018922214965 ) ) ;
#585=CARTESIAN_POINT ( 'NONE',  ( -52.92115514756972061, -86.34952198211959740, -4.330127018922185655 ) ) ;
#586=ORIENTED_EDGE ( 'NONE', *, *, #12943, .T. ) ;
#587=FACE_OUTER_BOUND ( 'NONE', #13970, .T. ) ;
#588=CIRCLE ( 'NONE', #9042, 1.500000000000000888 ) ;
#589=AXIS2_PLACEMENT_3D ( 'NONE', #10009, #16176, #5934 ) ;
#590=CARTESIAN_POINT ( 'NONE',  ( -49.79347899074619477, -23.08543803347279422, -21.65063509461098334 ) ) ;
#591=CIRCLE ( 'NONE', #11158, 1.500000000000001332 ) ;
#592=VERTEX_POINT ( 'NONE', #4242 ) ;
#593=ORIENTED_EDGE ( 'NONE', *, *, #12961, .T. ) ;
#594=ORIENTED_EDGE ( 'NONE', *, *, #8585, .F. ) ;
#595=CARTESIAN_POINT ( 'NONE',  ( -42.38608437559395270, -21.91048909185306570, 1.926565525561698076E-14 ) ) ;
#596=EDGE_CURVE ( 'NONE', #7360, #1643, #10020, .T. ) ;
#597=FACE_BOUND ( 'NONE', #11849, .T. ) ;
#598=EDGE_CURVE ( 'NONE', #9513, #6519, #16338, .T. ) ;
#599=AXIS2_PLACEMENT_3D ( 'NONE', #9609, #16835, #3523 ) ;
#600=ADVANCED_FACE ( 'NONE', ( #10108 ), #4133, .F. ) ;
#601=EDGE_CURVE ( 'NONE', #8134, #12438, #12857, .T. ) ;
#602=CARTESIAN_POINT ( 'NONE',  ( -20.86208015875458344, -23.55889513208593655, 4.330127018922217630 ) ) ;
#604=ORIENTED_EDGE ( 'NONE', *, *, #11122, .T. ) ;
#605=VECTOR ( 'NONE', #12622, 1000.000000000000000 ) ;
#606=AXIS2_PLACEMENT_3D ( 'NONE', #12503, #16894, #9679 ) ;
#608=ORIENTED_EDGE ( 'NONE', *, *, #18557, .T. ) ;
#609=FACE_BOUND ( 'NONE', #5299, .T. ) ;
#612=ORIENTED_EDGE ( 'NONE', *, *, #8796, .F. ) ;
#613=DIRECTION ( 'NONE',  ( -0.9876526153536336894, -0.1566598588826349503, 0.000000000000000000 ) ) ;
#614=FACE_OUTER_BOUND ( 'NONE', #5842, .T. ) ;
#615=AXIS2_PLACEMENT_3D ( 'NONE', #12181, #13417, #453 ) ;
#616=DIRECTION ( 'NONE',  ( -0.1566598588826321192, 0.9876526153536342445, 7.798540720466730171E-17 ) ) ;
#617=DIRECTION ( 'NONE',  ( -0.9876526153536336894, -0.1566598588826349503, 0.000000000000000000 ) ) ;
#618=ORIENTED_EDGE ( 'NONE', *, *, #8953, .T. ) ;
#620=CARTESIAN_POINT ( 'NONE',  ( -0.5755665338273089349, -78.04654946134009208, -21.65063509461098690 ) ) ;
#621=AXIS2_PLACEMENT_3D ( 'NONE', #894, #5241, #613 ) ;
#622=CARTESIAN_POINT ( 'NONE',  ( 0.000000000000000000, 0.000000000000000000, 24.99999999999999289 ) ) ;
#623=CYLINDRICAL_SURFACE ( 'NONE', #6256, 1.500000000000001554 ) ;
#624=ORIENTED_EDGE ( 'NONE', *, *, #17746, .T. ) ;
#625=FACE_OUTER_BOUND ( 'NONE', #8989, .T. ) ;
#626=VERTEX_POINT ( 'NONE', #5942 ) ;
#627=VECTOR ( 'NONE', #13045, 1000.000000000000000 ) ;
#628=FACE_OUTER_BOUND ( 'NONE', #2003, .T. ) ;
#629=CIRCLE ( 'NONE', #16060, 1.500000000000000888 ) ;
#630=DIRECTION ( 'NONE',  ( -0.9876526153536341335, -0.1566598588826330907, 0.000000000000000000 ) ) ;
#631=EDGE_CURVE ( 'NONE', #4650, #2328, #2045, .T. ) ;
#632=EDGE_LOOP ( 'NONE', ( #12628, #11654, #16155, #8883 ) ) ;
#633=CIRCLE ( 'NONE', #2130, 1.500000000000000000 ) ;
#635=DIRECTION ( 'NONE',  ( 0.000000000000000000, 0.000000000000000000, 1.000000000000000000 ) ) ;
#637=CYLINDRICAL_SURFACE ( 'NONE', #5402, 1.500000000000001554 ) ;
#638=DIRECTION ( 'NONE',  ( 0.000000000000000000, 0.000000000000000000, 1.000000000000000000 ) ) ;
#639=EDGE_LOOP ( 'NONE', ( #12804, #15222 ) ) ;
#640=EDGE_LOOP ( 'NONE', ( #4206, #1912, #17476, #10777 ) ) ;
#641=DIRECTION ( 'NONE',  ( -0.1566598588826321192, 0.9876526153536342445, 7.798540720466730171E-17 ) ) ;
#642=EDGE_LOOP ( 'NONE', ( #576, #3191 ) ) ;
#643=AXIS2_PLACEMENT_3D ( 'NONE', #1751, #7726, #1586 ) ;
#644=CARTESIAN_POINT ( 'NONE',  ( -33.00338452973448966, -20.42222043246806606, 12.99038105676661736 ) ) ;
#645=ORIENTED_EDGE ( 'NONE', *, *, #717, .T. ) ;
#646=DIRECTION ( 'NONE',  ( -0.1566598588826321747, 0.9876526153536343555, 0.000000000000000000 ) ) ;
#647=CARTESIAN_POINT ( 'NONE',  ( 10.28861223506262412, -76.32329101363113466, -8.660254037844389075 ) ) ;
#649=CYLINDRICAL_SURFACE ( 'NONE', #9079, 1.500000000000001554 ) ;
#652=DIRECTION ( 'NONE',  ( -0.1566598588826321747, 0.9876526153536343555, 0.000000000000000000 ) ) ;
#653=EDGE_CURVE ( 'NONE', #16941, #893, #3016, .T. ) ;
#654=AXIS2_PLACEMENT_3D ( 'NONE', #15823, #11614, #7302 ) ;
#655=ADVANCED_FACE ( 'NONE', ( #2425 ), #15585, .F. ) ;
#656=DIRECTION ( 'NONE',  ( -0.1566598588826321747, 0.9876526153536343555, 0.000000000000000000 ) ) ;
#657=DIRECTION ( 'NONE',  ( -0.9876526153536336894, -0.1566598588826349503, 0.000000000000000000 ) ) ;
#658=FACE_BOUND ( 'NONE', #11920, .T. ) ;
#659=CARTESIAN_POINT ( 'NONE',  ( -84.16561914167408531, -33.59999999999994458, -30.00000000000000000 ) ) ;
#661=FACE_OUTER_BOUND ( 'NONE', #1913, .T. ) ;
#662=EDGE_CURVE ( 'NONE', #6476, #14356, #11311, .T. ) ;
#663=CARTESIAN_POINT ( 'NONE',  ( -33.20773785067495254, -25.51714336811882688, -17.32050807568878170 ) ) ;
#664=CARTESIAN_POINT ( 'NONE',  ( -49.79347899074619477, -23.08543803347279777, -12.99038105676658006 ) ) ;
#665=ORIENTED_EDGE ( 'NONE', *, *, #1714, .F. ) ;
#666=AXIS2_PLACEMENT_3D ( 'NONE', #9517, #14150, #12441 ) ;
#667=CARTESIAN_POINT ( 'NONE',  ( -64.77298653181324539, -88.22944028871116018, 4.330127018922213189 ) ) ;
#670=VECTOR ( 'NONE', #1243, 1000.000000000000000 ) ;
#672=ORIENTED_EDGE ( 'NONE', *, *, #2828, .F. ) ;
#673=CIRCLE ( 'NONE', #17636, 1.500000000000001332 ) ;
#674=DIRECTION ( 'NONE',  ( -0.9876526153536341335, -0.1566598588826327021, 0.000000000000000000 ) ) ;
#675=CARTESIAN_POINT ( 'NONE',  ( -70.24471092643608472, -31.39188807621751209, -4.330127018922181215 ) ) ;
#677=CARTESIAN_POINT ( 'NONE',  ( -21.84973277410820458, -23.71555499096855613, 8.660254037844417496 ) ) ;
#680=ORIENTED_EDGE ( 'NONE', *, *, #12590, .F. ) ;
#681=( LENGTH_UNIT ( ) NAMED_UNIT ( * ) SI_UNIT ( .MILLI., .METRE. ) );
#683=EDGE_CURVE ( 'NONE', #5280, #3602, #11594, .T. ) ;
#684=DIRECTION ( 'NONE',  ( -0.1566598588826321192, 0.9876526153536342445, 7.798540720466730171E-17 ) ) ;
#685=CARTESIAN_POINT ( 'NONE',  ( -84.16561914167408531, -33.59999999999994458, 30.00000000000000000 ) ) ;
#686=AXIS2_PLACEMENT_3D ( 'NONE', #16566, #452, #6525 ) ;
#687=ORIENTED_EDGE ( 'NONE', *, *, #7447, .F. ) ;
#688=EDGE_LOOP ( 'NONE', ( #15524, #11717, #9471, #1813 ) ) ;
#689=EDGE_LOOP ( 'NONE', ( #1640, #7060 ) ) ;
#690=EDGE_CURVE ( 'NONE', #16087, #855, #10278, .T. ) ;
#691=ORIENTED_EDGE ( 'NONE', *, *, #6782, .T. ) ;
#692=EDGE_LOOP ( 'NONE', ( #8385, #4021 ) ) ;
#693=DIRECTION ( 'NONE',  ( -1.000000000000000000, 0.000000000000000000, 0.000000000000000000 ) ) ;
#694=FACE_BOUND ( 'NONE', #15508, .T. ) ;
#695=CYLINDRICAL_SURFACE ( 'NONE', #15624, 1.500000000000001554 ) ;
#696=DIRECTION ( 'NONE',  ( 0.000000000000000000, 0.000000000000000000, 1.000000000000000000 ) ) ;
#697=VERTEX_POINT ( 'NONE', #8248 ) ;
#699=DIRECTION ( 'NONE',  ( -0.1566598588826321192, 0.9876526153536342445, 7.798540720466731404E-17 ) ) ;
#700=CARTESIAN_POINT ( 'NONE',  ( -28.22983976372896109, -82.43302551005379541, 12.99038105676661203 ) ) ;
#701=CARTESIAN_POINT ( 'NONE',  ( -79.30363509306917535, 32.43333333333333002, 25.00000000000002132 ) ) ;
#702=CYLINDRICAL_SURFACE ( 'NONE', #4184, 1.500000000000001554 ) ;
#704=EDGE_CURVE ( 'NONE', #8986, #862, #12070, .T. ) ;
#705=EDGE_LOOP ( 'NONE', ( #18497, #13074 ) ) ;
#706=ORIENTED_EDGE ( 'NONE', *, *, #10496, .T. ) ;
#707=DIRECTION ( 'NONE',  ( -0.1566598588826321192, 0.9876526153536342445, 7.798540720466731404E-17 ) ) ;
#708=EDGE_CURVE ( 'NONE', #13151, #10116, #6664, .T. ) ;
#709=DIRECTION ( 'NONE',  ( -0.1566598588826321192, 0.9876526153536342445, 7.798540720466730171E-17 ) ) ;
#710=ORIENTED_EDGE ( 'NONE', *, *, #11771, .F. ) ;
#711=CARTESIAN_POINT ( 'NONE',  ( -48.97054468615517919, -85.72288254658906226, 17.32050807568881368 ) ) ;
#712=EDGE_CURVE ( 'NONE', #4620, #15439, #5093, .T. ) ;
#713=CARTESIAN_POINT ( 'NONE',  ( -4.565812005419673802, -20.97400746052251108, 12.99038105676661026 ) ) ;
#714=ORIENTED_EDGE ( 'NONE', *, *, #10708, .T. ) ;
#717=EDGE_CURVE ( 'NONE', #8478, #7247, #7561, .T. ) ;
#719=VERTEX_POINT ( 'NONE', #12471 ) ;
#720=FACE_BOUND ( 'NONE', #3866, .T. ) ;
#721=CARTESIAN_POINT ( 'NONE',  ( -2.096680467035594297, -20.58235781331593017, -8.660254037844383745 ) ) ;
#722=CARTESIAN_POINT ( 'NONE',  ( -46.50141314777108903, -85.33123289938248490, 21.65063509461101532 ) ) ;
#723=CARTESIAN_POINT ( 'NONE',  ( -30.73860631229088725, -25.12549372091224598, 21.65063509461101887 ) ) ;
#724=CYLINDRICAL_SURFACE ( 'NONE', #1811, 1.500000000000001554 ) ;
#725=CARTESIAN_POINT ( 'NONE',  ( -8.516422466834198346, -21.60064689605303911, -17.32050807568878170 ) ) ;
#726=CARTESIAN_POINT ( 'NONE',  ( -77.65210554158829837, -32.56683701783724416, -8.660254037844380193 ) ) ;
#727=EDGE_CURVE ( 'NONE', #16068, #9239, #3604, .T. ) ;
#728=DIRECTION ( 'NONE',  ( -0.1566598588826321192, 0.9876526153536342445, 7.798540720466731404E-17 ) ) ;
#729=ADVANCED_FACE ( 'NONE', ( #13640 ), #2185, .F. ) ;
#730=VERTEX_POINT ( 'NONE', #6878 ) ;
#731=ORIENTED_EDGE ( 'NONE', *, *, #2510, .T. ) ;
#734=CYLINDRICAL_SURFACE ( 'NONE', #16067, 1.500000000000001554 ) ;
#735=ORIENTED_EDGE ( 'NONE', *, *, #17861, .T. ) ;
#737=ORIENTED_EDGE ( 'NONE', *, *, #9685, .F. ) ;
#738=EDGE_CURVE ( 'NONE', #5480, #5362, #12722, .T. ) ;
#740=DIRECTION ( 'NONE',  ( -0.9876526153536341335, -0.1566598588826327021, 0.000000000000000000 ) ) ;
#741=CARTESIAN_POINT ( 'NONE',  ( -72.71384246482016067, -31.78353772342409300, 8.660254037844417496 ) ) ;
#743=DIRECTION ( 'NONE',  ( -0.1566598588826321192, 0.9876526153536342445, 7.798540720466731404E-17 ) ) ;
#745=DIRECTION ( 'NONE',  ( -0.1566598588826321192, 0.9876526153536342445, 7.798540720466730171E-17 ) ) ;
#747=CARTESIAN_POINT ( 'NONE',  ( -56.91140061916207316, -29.27697998130197732, 21.65063509461101887 ) ) ;
#749=DIRECTION ( 'NONE',  ( 0.000000000000000000, 0.000000000000000000, 1.000000000000000000 ) ) ;
#750=ORIENTED_EDGE ( 'NONE', *, *, #11331, .T. ) ;
#752=VECTOR ( 'NONE', #5936, 1000.000000000000000 ) ;
#754=ADVANCED_FACE ( 'NONE', ( #2793 ), #7079, .F. ) ;
#755=VERTEX_POINT ( 'NONE', #15859 ) ;
#756=ORIENTED_EDGE ( 'NONE', *, *, #631, .F. ) ;
#758=CARTESIAN_POINT ( 'NONE',  ( 6.831828081324923474, -76.87160051972034580, 8.660254037844406838 ) ) ;
#759=ORIENTED_EDGE ( 'NONE', *, *, #8356, .F. ) ;
#760=DIRECTION ( 'NONE',  ( -0.9876526153536336894, -0.1566598588826349503, 0.000000000000000000 ) ) ;
#761=ADVANCED_FACE ( 'NONE', ( #14689 ), #17671, .F. ) ;
#762=DIRECTION ( 'NONE',  ( -0.9876526153536341335, -0.1566598588826327021, 0.000000000000000000 ) ) ;
#763=ORIENTED_EDGE ( 'NONE', *, *, #17578, .T. ) ;
#764=FACE_OUTER_BOUND ( 'NONE', #7194, .T. ) ;
#767=CIRCLE ( 'NONE', #14675, 1.499999999999999556 ) ;
#770=ORIENTED_EDGE ( 'NONE', *, *, #8506, .F. ) ;
#771=DIRECTION ( 'NONE',  ( 0.000000000000000000, 0.000000000000000000, 1.000000000000000000 ) ) ;
#772=CARTESIAN_POINT ( 'NONE',  ( -43.86756329862441817, -22.14547888017700217, -17.32050807568878170 ) ) ;
#773=DIRECTION ( 'NONE',  ( -0.9876526153536341335, -0.1566598588826327021, 0.000000000000000000 ) ) ;
#774=CARTESIAN_POINT ( 'NONE',  ( -40.08167114797250719, -84.31294381664535820, -4.330127018922185655 ) ) ;
#776=EDGE_LOOP ( 'NONE', ( #9787, #14436, #16293, #12999 ) ) ;
#777=VERTEX_POINT ( 'NONE', #10233 ) ;
#778=EDGE_LOOP ( 'NONE', ( #10197, #3952, #17970, #7335 ) ) ;
#779=EDGE_LOOP ( 'NONE', ( #18617, #8741 ) ) ;
#781=AXIS2_PLACEMENT_3D ( 'NONE', #9710, #793, #3786 ) ;
#782=FACE_BOUND ( 'NONE', #531, .T. ) ;
#785=CIRCLE ( 'NONE', #5003, 1.499999999999999556 ) ;
#786=CARTESIAN_POINT ( 'NONE',  ( -32.50955822205765600, -20.34389050302674562, -8.660254037844380193 ) ) ;
#788=FACE_BOUND ( 'NONE', #3592, .T. ) ;
#790=AXIS2_PLACEMENT_3D ( 'NONE', #5797, #17364, #11534 ) ;
#792=CARTESIAN_POINT ( 'NONE',  ( -29.05277406831996245, -19.79558099693754158, 17.32050807568882078 ) ) ;
#793=DIRECTION ( 'NONE',  ( -0.1566598588826321747, 0.9876526153536343555, 0.000000000000000000 ) ) ;
#794=VERTEX_POINT ( 'NONE', #15247 ) ;
#795=VERTEX_POINT ( 'NONE', #14107 ) ;
#796=CARTESIAN_POINT ( 'NONE',  ( -40.57549745564934085, -84.39127374608669641, 1.424741226644455312E-14 ) ) ;
#798=DIRECTION ( 'NONE',  ( -0.1566598588826321192, 0.9876526153536342445, 7.798540720466730171E-17 ) ) ;
#799=EDGE_LOOP ( 'NONE', ( #13422, #7345, #16257, #5142 ) ) ;
#801=DIRECTION ( 'NONE',  ( -0.9876526153536336894, -0.1566598588826350336, 0.000000000000000000 ) ) ;
#803=ORIENTED_EDGE ( 'NONE', *, *, #16114, .T. ) ;
#805=ORIENTED_EDGE ( 'NONE', *, *, #9038, .T. ) ;
#806=AXIS2_PLACEMENT_3D ( 'NONE', #11891, #3185, #17730 ) ;
#807=EDGE_CURVE ( 'NONE', #4830, #12067, #9970, .T. ) ;
#808=CARTESIAN_POINT ( 'NONE',  ( -9.299721761247353058, -16.66238381928489787, 8.660254037844413944 ) ) ;
#809=ADVANCED_FACE ( 'NONE', ( #14209 ), #3858, .F. ) ;
#810=CARTESIAN_POINT ( 'NONE',  ( -48.02252708097940825, -27.86704125135830523, 1.869203119972154228E-14 ) ) ;
#813=ORIENTED_EDGE ( 'NONE', *, *, #339, .F. ) ;
#814=CIRCLE ( 'NONE', #2022, 1.499999999999999556 ) ;
#815=CARTESIAN_POINT ( 'NONE',  ( -22.34355908178503114, -23.79388492040988012, -21.65063509461098334 ) ) ;
#817=CARTESIAN_POINT ( 'NONE',  ( -47.98289207080156160, -85.56622268770642847, 12.99038105676661203 ) ) ;
#818=FACE_OUTER_BOUND ( 'NONE', #1173, .T. ) ;
#819=ORIENTED_EDGE ( 'NONE', *, *, #8066, .F. ) ;
#821=FACE_OUTER_BOUND ( 'NONE', #16486, .T. ) ;
#823=EDGE_LOOP ( 'NONE', ( #1463, #16116, #18789, #5628 ) ) ;
#825=CARTESIAN_POINT ( 'NONE',  ( -40.57549745564932664, -84.39127374608669641, 8.660254037844412167 ) ) ;
#828=ORIENTED_EDGE ( 'NONE', *, *, #3619, .F. ) ;
#829=CIRCLE ( 'NONE', #17492, 1.500000000000000000 ) ;
#831=CYLINDRICAL_SURFACE ( 'NONE', #12076, 1.500000000000000666 ) ;
#832=CARTESIAN_POINT ( 'NONE',  ( -51.27495791377664602, -23.32042782179673779, -21.65063509461097979 ) ) ;
#833=EDGE_CURVE ( 'NONE', #4754, #3060, #17278, .T. ) ;
#834=ADVANCED_FACE ( 'NONE', ( #14585 ), #14490, .F. ) ;
#835=DIRECTION ( 'NONE',  ( -0.1566598588826321192, 0.9876526153536342445, 7.798540720466730171E-17 ) ) ;
#838=ORIENTED_EDGE ( 'NONE', *, *, #18207, .F. ) ;
#839=DIRECTION ( 'NONE',  ( -0.1566598588826321192, 0.9876526153536342445, 7.798540720466730171E-17 ) ) ;
#840=AXIS2_PLACEMENT_3D ( 'NONE', #8135, #16786, #5089 ) ;
#841=DIRECTION ( 'NONE',  ( -0.9876526153536341335, -0.1566598588826327021, 0.000000000000000000 ) ) ;
#842=FACE_OUTER_BOUND ( 'NONE', #11073, .T. ) ;
#843=VECTOR ( 'NONE', #10454, 1000.000000000000000 ) ;
#847=CARTESIAN_POINT ( 'NONE',  ( -42.87991068327079347, -21.98881902129437194, -12.99038105676658006 ) ) ;
#848=DIRECTION ( 'NONE',  ( -0.1566598588826321192, 0.9876526153536342445, 7.798540720466731404E-17 ) ) ;
#849=EDGE_LOOP ( 'NONE', ( #13453, #13783, #15744, #11573 ) ) ;
#850=ORIENTED_EDGE ( 'NONE', *, *, #10300, .T. ) ;
#851=CARTESIAN_POINT ( 'NONE',  ( -5.349111299832828514, -16.03574438375436984, 21.65063509461101177 ) ) ;
#852=DIRECTION ( 'NONE',  ( -0.9876526153536336894, -0.1566598588826349503, 0.000000000000000000 ) ) ;
#853=ORIENTED_EDGE ( 'NONE', *, *, #1767, .F. ) ;
#854=AXIS2_PLACEMENT_3D ( 'NONE', #7811, #428, #17704 ) ;
#855=VERTEX_POINT ( 'NONE', #13058 ) ;
#856=DIRECTION ( 'NONE',  ( -0.1566598588826321192, 0.9876526153536342445, 7.798540720466730171E-17 ) ) ;
#857=EDGE_LOOP ( 'NONE', ( #17739, #13981 ) ) ;
#858=CARTESIAN_POINT ( 'NONE',  ( -5.349111299832828514, -16.03574438375436984, -12.99038105676658006 ) ) ;
#859=VERTEX_POINT ( 'NONE', #91 ) ;
#862=VERTEX_POINT ( 'NONE', #10482 ) ;
#863=DIRECTION ( 'NONE',  ( 0.000000000000000000, 0.000000000000000000, 1.000000000000000000 ) ) ;
#864=DIRECTION ( 'NONE',  ( 0.000000000000000000, 0.000000000000000000, 1.000000000000000000 ) ) ;
#865=VECTOR ( 'NONE', #5049, 1000.000000000000000 ) ;
#867=DIRECTION ( 'NONE',  ( -0.1566598588826321192, 0.9876526153536342445, 7.798540720466730171E-17 ) ) ;
#868=FACE_OUTER_BOUND ( 'NONE', #902, .T. ) ;
#869=ORIENTED_EDGE ( 'NONE', *, *, #10612, .T. ) ;
#871=EDGE_LOOP ( 'NONE', ( #12940, #17306, #8437, #16097 ) ) ;
#872=EDGE_CURVE ( 'NONE', #12166, #14919, #9068, .T. ) ;
#873=ADVANCED_FACE ( 'NONE', ( #3102 ), #11109, .F. ) ;
#874=DIRECTION ( 'NONE',  ( -0.9876526153536336894, -0.1566598588826349503, 0.000000000000000000 ) ) ;
#875=CARTESIAN_POINT ( 'NONE',  ( -48.80582637539256297, -22.92877817459016399, -8.660254037844380193 ) ) ;
#877=DIRECTION ( 'NONE',  ( -0.9876526153536336894, -0.1566598588826349503, 0.000000000000000000 ) ) ;
#878=EDGE_CURVE ( 'NONE', #16586, #8364, #5126, .T. ) ;
#879=ORIENTED_EDGE ( 'NONE', *, *, #394, .F. ) ;
#880=EDGE_LOOP ( 'NONE', ( #16122, #16267, #14072, #18069 ) ) ;
#881=ORIENTED_EDGE ( 'NONE', *, *, #6302, .T. ) ;
#882=DIRECTION ( 'NONE',  ( -0.1566598588826321192, 0.9876526153536342445, 7.798540720466730171E-17 ) ) ;
#884=FACE_BOUND ( 'NONE', #6398, .T. ) ;
#885=DIRECTION ( 'NONE',  ( -0.1566598588826321747, 0.9876526153536343555, 0.000000000000000000 ) ) ;
#886=VERTEX_POINT ( 'NONE', #3551 ) ;
#887=VECTOR ( 'NONE', #3303, 1000.000000000000000 ) ;
#888=CYLINDRICAL_SURFACE ( 'NONE', #8455, 1.500000000000001554 ) ;
#889=AXIS2_PLACEMENT_3D ( 'NONE', #3859, #9849, #13920 ) ;
#890=EDGE_CURVE ( 'NONE', #98, #3520, #18190, .T. ) ;
#891=CARTESIAN_POINT ( 'NONE',  ( -34.19539046602857724, -25.67380322700145356, -12.99038105676658006 ) ) ;
#892=CIRCLE ( 'NONE', #17254, 1.500000000000000888 ) ;
#893=VERTEX_POINT ( 'NONE', #18016 ) ;
#894=CARTESIAN_POINT ( 'NONE',  ( -56.37793930130741415, -86.89783148820879433, -12.99038105676658539 ) ) ;
#895=LINE ( 'NONE', #15645, #17841 ) ;
#896=CARTESIAN_POINT ( 'NONE',  ( -65.30644784966793281, -30.60858878180435738, -21.65063509461098334 ) ) ;
#898=VERTEX_POINT ( 'NONE', #6885 ) ;
#900=ADVANCED_FACE ( 'NONE', ( #4200 ), #11393, .F. ) ;
#902=EDGE_LOOP ( 'NONE', ( #12357, #18724, #16202, #3889 ) ) ;
#903=VECTOR ( 'NONE', #7351, 1000.000000000000000 ) ;
#904=ORIENTED_EDGE ( 'NONE', *, *, #17050, .F. ) ;
#905=CARTESIAN_POINT ( 'NONE',  ( -55.42992169613163611, -29.04199019297804085, -4.330127018922181215 ) ) ;
#906=AXIS2_PLACEMENT_3D ( 'NONE', #274, #1790, #11900 ) ;
#907=ORIENTED_EDGE ( 'NONE', *, *, #8935, .T. ) ;
#908=CARTESIAN_POINT ( 'NONE',  ( -2.590506774712417748, -20.66068774275724707, 21.65063509461101177 ) ) ;
#909=EDGE_CURVE ( 'NONE', #15855, #10665, #14442, .T. ) ;
#910=ORIENTED_EDGE ( 'NONE', *, *, #2829, .F. ) ;
#911=CIRCLE ( 'NONE', #16330, 1.500000000000001332 ) ;
#913=DIRECTION ( 'NONE',  ( -0.1566598588826321747, 0.9876526153536343555, 0.000000000000000000 ) ) ;
#914=DIRECTION ( 'NONE',  ( -0.1566598588826321192, 0.9876526153536342445, 7.798540720466730171E-17 ) ) ;
#916=AXIS2_PLACEMENT_3D ( 'NONE', #13711, #15331, #3949 ) ;
#917=DIRECTION ( 'NONE',  ( -0.1566598588826321192, 0.9876526153536342445, 7.798540720466730171E-17 ) ) ;
#919=FACE_OUTER_BOUND ( 'NONE', #18493, .T. ) ;
#920=DIRECTION ( 'NONE',  ( 0.000000000000000000, 0.000000000000000000, 1.000000000000000000 ) ) ;
#921=LINE ( 'NONE', #18672, #18060 ) ;
#923=ORIENTED_EDGE ( 'NONE', *, *, #11613, .T. ) ;
#924=ORIENTED_EDGE ( 'NONE', *, *, #12167, .F. ) ;
#925=DIRECTION ( 'NONE',  ( -0.1566598588826321747, 0.9876526153536343555, 0.000000000000000000 ) ) ;
#926=DIRECTION ( 'NONE',  ( -0.1566598588826321747, 0.9876526153536343555, 0.000000000000000000 ) ) ;
#928=CIRCLE ( 'NONE', #9702, 1.500000000000001332 ) ;
#929=ORIENTED_EDGE ( 'NONE', *, *, #10244, .F. ) ;
#930=ORIENTED_EDGE ( 'NONE', *, *, #11892, .T. ) ;
#931=VERTEX_POINT ( 'NONE', #7355 ) ;
#932=DIRECTION ( 'NONE',  ( -0.9876526153536341335, -0.1566598588826327021, 0.000000000000000000 ) ) ;
#933=ADVANCED_FACE ( 'NONE', ( #17778, #2013, #3142, #13463, #416, #7623, #6298, #17491, #8934, #4756, #7798, #4478, #609, #16055, #12129, #17969, #3700, #6484, #2200, #16910, #12222, #5020, #10800, #16616, #788, #9500, #15268, #2284, #14238, #6958, #1361, #14418, #11557, #11368, #12807, #18648, #5617, #2772, #7235, #7141, #17384, #12889, #7600, #13257, #483, #17466, #4454, #291, #9106, #11832, #17758, #16030, #3041, #1634, #5980, #4556, #10778, #6376, #6552, #13535, #3488, #9386, #10976, #1991, #7874, #3681, #11067, #7776, #3767, #2267, #11535, #15453, #18631, #8543, #1343, #11164, #1430, #5599, #10035, #18535, #4051, #9853, #4258, #7125, #8897, #13146, #6160, #4709, #1521, #1691, #10486, #458, #4530, #6248, #17365, #17447, #16005, #3015, #658, #18019, #9356, #2161, #12273, #18112, #16392, #10854, #3656, #8025, #11978, #17824, #10367, #14557, #5930, #338, #17509, #236, #17794, #16169, #1750, #7641, #4773, #16358, #9151, #5159, #18186, #720, #15012, #16838, #3800, #9611, #2219, #12238, #2030, #5045, #10817, #15385, #2403, #8943, #1389, #17226, #1574, #4586, #13196, #12916, #6011, #16158, #13294, #15787, #13017, #1282, #2854, #120, #14424, #13171, #1452, #7066, #5623, #5824, #11564, #17390, #4375, #15935, #14526, #1551, #11118, #17127, #4103, #10936, #16943, #5557, #3914, #4011, #5459, #2518, #18299, #11219, #6997, #18390, #2317, #8305, #15301, #8388 ), #13873, .F. ) ;
#934=AXIS2_PLACEMENT_3D ( 'NONE', #18591, #925, #11307 ) ;
#936=CARTESIAN_POINT ( 'NONE',  ( 5.350349158294472218, -77.10659030804430358, 8.660254037844406838 ) ) ;
#937=CIRCLE ( 'NONE', #15133, 1.500000000000001332 ) ;
#938=DIRECTION ( 'NONE',  ( -0.9876526153536336894, -0.1566598588826349503, 0.000000000000000000 ) ) ;
#939=LINE ( 'NONE', #10844, #13609 ) ;
#940=CARTESIAN_POINT ( 'NONE',  ( -41.39843176024032800, -21.75382923297042836, -4.330127018922180326 ) ) ;
#941=AXIS2_PLACEMENT_3D ( 'NONE', #8136, #17532, #7463 ) ;
#942=CARTESIAN_POINT ( 'NONE',  ( -24.27922930231443743, -81.80638607452326028, -17.32050807568878525 ) ) ;
#943=FILL_AREA_STYLE ('',( #2157 ) ) ;
#944=CYLINDRICAL_SURFACE ( 'NONE', #1796, 1.500000000000001554 ) ;
#945=EDGE_CURVE ( 'NONE', #17224, #18075, #18675, .T. ) ;
#946=CARTESIAN_POINT ( 'NONE',  ( -44.85521591397802155, -22.30213873905964661, 4.330127018922218518 ) ) ;
#947=AXIS2_PLACEMENT_3D ( 'NONE', #13306, #1941, #340 ) ;
#948=DIRECTION ( 'NONE',  ( 0.000000000000000000, 0.000000000000000000, 1.000000000000000000 ) ) ;
#950=DIRECTION ( 'NONE',  ( -0.1566598588826321192, 0.9876526153536342445, 7.798540720466730171E-17 ) ) ;
#951=CIRCLE ( 'NONE', #3049, 1.500000000000000888 ) ;
#952=EDGE_CURVE ( 'NONE', #7902, #17807, #2411, .T. ) ;
#953=ORIENTED_EDGE ( 'NONE', *, *, #7118, .F. ) ;
#954=ORIENTED_EDGE ( 'NONE', *, *, #1714, .T. ) ;
#956=DIRECTION ( 'NONE',  ( -0.1566598588826321747, 0.9876526153536343555, 0.000000000000000000 ) ) ;
#957=EDGE_CURVE ( 'NONE', #12710, #4380, #15759, .T. ) ;
#958=FACE_OUTER_BOUND ( 'NONE', #9602, .T. ) ;
#959=VERTEX_POINT ( 'NONE', #1210 ) ;
#960=EDGE_CURVE ( 'NONE', #15970, #4650, #1538, .T. ) ;
#961=AXIS2_PLACEMENT_3D ( 'NONE', #18768, #147, #1663 ) ;
#962=EDGE_LOOP ( 'NONE', ( #982, #2651 ) ) ;
#964=ORIENTED_EDGE ( 'NONE', *, *, #1067, .F. ) ;
#965=CIRCLE ( 'NONE', #654, 1.500000000000000888 ) ;
#966=CARTESIAN_POINT ( 'NONE',  ( -47.03487446562579777, -27.71038139247566789, -21.65063509461098334 ) ) ;
#968=VERTEX_POINT ( 'NONE', #6707 ) ;
#969=DIRECTION ( 'NONE',  ( -0.1566598588826321192, 0.9876526153536342445, 7.798540720466730171E-17 ) ) ;
#971=CARTESIAN_POINT ( 'NONE',  ( -9.464440072009985272, -79.45648819128378193, 8.660254037844412167 ) ) ;
#972=CARTESIAN_POINT ( 'NONE',  ( -68.72359699322777260, -88.85607972424168111, -17.32050807568878525 ) ) ;
#973=CARTESIAN_POINT ( 'NONE',  ( -7.982961148979534016, -79.22149840295983836, 1.443110928631665584E-14 ) ) ;
#974=AXIS2_PLACEMENT_3D ( 'NONE', #15485, #9425, #17025 ) ;
#975=( NAMED_UNIT ( * ) SI_UNIT ( $, .STERADIAN. ) SOLID_ANGLE_UNIT ( ) );
#976=DIRECTION ( 'NONE',  ( -0.1566598588826321747, 0.9876526153536343555, 0.000000000000000000 ) ) ;
#979=AXIS2_PLACEMENT_3D ( 'NONE', #8665, #13009, #11657 ) ;
#980=EDGE_CURVE ( 'NONE', #15050, #12253, #16678, .T. ) ;
#981=DIRECTION ( 'NONE',  ( -0.1566598588826321192, 0.9876526153536342445, 7.798540720466731404E-17 ) ) ;
#982=ORIENTED_EDGE ( 'NONE', *, *, #17143, .F. ) ;
#983=VERTEX_POINT ( 'NONE', #1306 ) ;
#984=ORIENTED_EDGE ( 'NONE', *, *, #17637, .F. ) ;
#988=EDGE_LOOP ( 'NONE', ( #7419, #3433, #3820, #3749 ) ) ;
#989=FACE_BOUND ( 'NONE', #4224, .T. ) ;
#990=EDGE_CURVE ( 'NONE', #13999, #9162, #7089, .T. ) ;
#991=LINE ( 'NONE', #6761, #9455 ) ;
#992=ORIENTED_EDGE ( 'NONE', *, *, #3502, .T. ) ;
#993=CIRCLE ( 'NONE', #7939, 1.500000000000000444 ) ;
#994=DIRECTION ( 'NONE',  ( -0.1566598588826321747, 0.9876526153536343555, 0.000000000000000000 ) ) ;
#995=CARTESIAN_POINT ( 'NONE',  ( -78.43540483600145308, -27.62857394106912068, 8.660254037844417496 ) ) ;
#996=AXIS2_PLACEMENT_3D ( 'NONE', #6812, #18219, #10951 ) ;
#999=VERTEX_POINT ( 'NONE', #11022 ) ;
#1001=CARTESIAN_POINT ( 'NONE',  ( -33.16810284049710589, -83.21632480446696434, 12.99038105676661203 ) ) ;
#1002=DIRECTION ( 'NONE',  ( -0.9876526153536341335, -0.1566598588826327021, 0.000000000000000000 ) ) ;
#1003=EDGE_LOOP ( 'NONE', ( #17375, #14071 ) ) ;
#1004=CARTESIAN_POINT ( 'NONE',  ( -6.995308533625909320, -79.06483854407721878, -4.330127018922185655 ) ) ;
#1005=CARTESIAN_POINT ( 'NONE',  ( -53.74408945216072198, -23.71207746900332225, -8.660254037844380193 ) ) ;
#1006=AXIS2_PLACEMENT_3D ( 'NONE', #3862, #6839, #17082 ) ;
#1007=ORIENTED_EDGE ( 'NONE', *, *, #957, .F. ) ;
#1009=CARTESIAN_POINT ( 'NONE',  ( -41.56315007100295844, -84.54793360496931598, 4.330127018922213189 ) ) ;
#1011=LINE ( 'NONE', #12528, #2152 ) ;
#1013=EDGE_LOOP ( 'NONE', ( #16793, #1076 ) ) ;
#1014=CIRCLE ( 'NONE', #11559, 1.500000000000000444 ) ;
#1017=DIRECTION ( 'NONE',  ( -0.1566598588826321192, 0.9876526153536342445, 7.798540720466730171E-17 ) ) ;
#1018=EDGE_CURVE ( 'NONE', #16065, #3908, #5469, .T. ) ;
#1019=CARTESIAN_POINT ( 'NONE',  ( 0.4120860815263194254, -77.88988960245745830, 1.077796531449093893E-14 ) ) ;
#1022=ORIENTED_EDGE ( 'NONE', *, *, #8831, .T. ) ;
#1023=FACE_OUTER_BOUND ( 'NONE', #12507, .T. ) ;
#1024=DIRECTION ( 'NONE',  ( 0.000000000000000000, 0.000000000000000000, 1.000000000000000000 ) ) ;
#1027=EDGE_LOOP ( 'NONE', ( #5119, #9867, #15090, #4924 ) ) ;
#1028=VERTEX_POINT ( 'NONE', #18426 ) ;
#1029=VECTOR ( 'NONE', #16300, 1000.000000000000000 ) ;
#1030=CARTESIAN_POINT ( 'NONE',  ( -84.16561914167408531, -33.59999999999994458, 30.00000000000000000 ) ) ;
#1031=LINE ( 'NONE', #12349, #14856 ) ;
#1032=ORIENTED_EDGE ( 'NONE', *, *, #5749, .T. ) ;
#1033=ORIENTED_EDGE ( 'NONE', *, *, #17505, .T. ) ;
#1034=CARTESIAN_POINT ( 'NONE',  ( -66.25446545484369665, -88.46443007703511796, 4.330127018922213189 ) ) ;
#1035=LINE ( 'NONE', #12355, #2442 ) ;
#1038=ORIENTED_EDGE ( 'NONE', *, *, #11314, .T. ) ;
#1039=LINE ( 'NONE', #5277, #7907 ) ;
#1040=CYLINDRICAL_SURFACE ( 'NONE', #3177, 1.500000000000001554 ) ;
#1041=CARTESIAN_POINT ( 'NONE',  ( -7.034943543803747090, -21.36565710772908488, 1.540628126764003082E-14 ) ) ;
#1042=DIRECTION ( 'NONE',  ( -0.9876526153536341335, -0.1566598588826327021, 0.000000000000000000 ) ) ;
#1044=DIRECTION ( 'NONE',  ( -0.9876526153536341335, -0.1566598588826327021, 0.000000000000000000 ) ) ;
#1045=EDGE_CURVE ( 'NONE', #7610, #7134, #15447, .T. ) ;
#1046=CARTESIAN_POINT ( 'NONE',  ( -61.35583738825340561, -29.98194934627382224, 8.660254037844417496 ) ) ;
#1047=CARTESIAN_POINT ( 'NONE',  ( -76.17062661855784711, -32.33184722951329348, -8.660254037844380193 ) ) ;
#1049=ORIENTED_EDGE ( 'NONE', *, *, #16408, .F. ) ;
#1050=CARTESIAN_POINT ( 'NONE',  ( -5.059638313096497697, -21.05233738996382797, 17.32050807568881012 ) ) ;
#1051=ADVANCED_FACE ( 'NONE', ( #958 ), #2344, .F. ) ;
#1052=DIRECTION ( 'NONE',  ( -0.9876526153536341335, -0.1566598588826327021, 0.000000000000000000 ) ) ;
#1054=DIRECTION ( 'NONE',  ( 0.000000000000000000, 0.000000000000000000, 1.000000000000000000 ) ) ;
#1055=CARTESIAN_POINT ( 'NONE',  ( -70.24471092643608472, -31.39188807621751209, -12.99038105676658006 ) ) ;
#1056=FACE_OUTER_BOUND ( 'NONE', #254, .T. ) ;
#1057=ORIENTED_EDGE ( 'NONE', *, *, #8341, .F. ) ;
#1059=DIRECTION ( 'NONE',  ( -0.9876526153536336894, -0.1566598588826349503, 0.000000000000000000 ) ) ;
#1060=ORIENTED_EDGE ( 'NONE', *, *, #5810, .T. ) ;
#1062=DIRECTION ( 'NONE',  ( -0.1566598588826321747, 0.9876526153536343555, 0.000000000000000000 ) ) ;
#1063=VERTEX_POINT ( 'NONE', #4134 ) ;
#1065=DIRECTION ( 'NONE',  ( -0.1566598588826321192, 0.9876526153536342445, 7.798540720466730171E-17 ) ) ;
#1066=CARTESIAN_POINT ( 'NONE',  ( -37.61253960958842413, -83.92129416943879505, 17.32050807568881368 ) ) ;
#1067=EDGE_CURVE ( 'NONE', #2946, #18001, #15606, .T. ) ;
#1068=EDGE_CURVE ( 'NONE', #5828, #8019, #7573, .T. ) ;
#1069=DIRECTION ( 'NONE',  ( 0.000000000000000000, 0.000000000000000000, 1.000000000000000000 ) ) ;
#1072=FACE_OUTER_BOUND ( 'NONE', #248, .T. ) ;
#1073=ORIENTED_EDGE ( 'NONE', *, *, #10640, .T. ) ;
#1074=DIRECTION ( 'NONE',  ( 0.000000000000000000, 0.000000000000000000, 1.000000000000000000 ) ) ;
#1075=ORIENTED_EDGE ( 'NONE', *, *, #5040, .F. ) ;
#1076=ORIENTED_EDGE ( 'NONE', *, *, #2727, .T. ) ;
#1077=ORIENTED_EDGE ( 'NONE', *, *, #15950, .T. ) ;
#1078=CARTESIAN_POINT ( 'NONE',  ( -36.62488699423481364, -83.76463431055616127, -4.330127018922185655 ) ) ;
#1079=FACE_BOUND ( 'NONE', #10545, .T. ) ;
#1080=EDGE_CURVE ( 'NONE', #14612, #18673, #6076, .T. ) ;
#1081=DIRECTION ( 'NONE',  ( -0.9876526153536341335, -0.1566598588826327021, 0.000000000000000000 ) ) ;
#1082=VECTOR ( 'NONE', #17061, 1000.000000000000000 ) ;
#1083=EDGE_CURVE ( 'NONE', #12177, #4657, #17900, .T. ) ;
#1085=EDGE_LOOP ( 'NONE', ( #9067, #11367 ) ) ;
#1086=ADVANCED_FACE ( 'NONE', ( #11427 ), #1507, .F. ) ;
#1087=DIRECTION ( 'NONE',  ( -0.1566598588826321747, 0.9876526153536343555, 0.000000000000000000 ) ) ;
#1088=CARTESIAN_POINT ( 'NONE',  ( -72.01566283620284992, -26.61028485833201884, 8.660254037844417496 ) ) ;
#1089=DIRECTION ( 'NONE',  ( -0.1566598588826321192, 0.9876526153536342445, 7.798540720466731404E-17 ) ) ;
#1090=ORIENTED_EDGE ( 'NONE', *, *, #6326, .F. ) ;
#1091=CARTESIAN_POINT ( 'NONE',  ( -51.47931123471711601, -28.41535075744751282, -8.660254037844380193 ) ) ;
#1093=CARTESIAN_POINT ( 'NONE',  ( -71.02801022084922522, -26.45362499944937085, -21.65063509461097979 ) ) ;
#1095=VERTEX_POINT ( 'NONE', #11610 ) ;
#1096=DIRECTION ( 'NONE',  ( -0.1566598588826321192, 0.9876526153536342445, 7.798540720466730171E-17 ) ) ;
#1097=EDGE_LOOP ( 'NONE', ( #10806, #13544, #9035, #12463 ) ) ;
#1098=LINE ( 'NONE', #18475, #1570 ) ;
#1100=ORIENTED_EDGE ( 'NONE', *, *, #16560, .T. ) ;
#1101=CIRCLE ( 'NONE', #10147, 1.500000000000000888 ) ;
#1102=DIRECTION ( 'NONE',  ( -0.9876526153536341335, -0.1566598588826327021, 0.000000000000000000 ) ) ;
#1105=CARTESIAN_POINT ( 'NONE',  ( -54.44226908077799720, -28.88533033409540351, 17.32050807568881723 ) ) ;
#1106=CARTESIAN_POINT ( 'NONE',  ( -45.01993422474066620, -85.09624311105852712, -4.330127018922185655 ) ) ;
#1107=ORIENTED_EDGE ( 'NONE', *, *, #6048, .F. ) ;
#1108=EDGE_CURVE ( 'NONE', #2286, #13042, #7003, .T. ) ;
#1109=DIRECTION ( 'NONE',  ( -0.1566598588826321192, 0.9876526153536342445, 7.798540720466730171E-17 ) ) ;
#1110=DIRECTION ( 'NONE',  ( 0.000000000000000000, 0.000000000000000000, 1.000000000000000000 ) ) ;
#1111=EDGE_LOOP ( 'NONE', ( #10380, #9692, #2653, #16288 ) ) ;
#1112=ADVANCED_FACE ( 'NONE', ( #15817 ), #17434, .F. ) ;
#1113=VERTEX_POINT ( 'NONE', #14393 ) ;
#1114=DIRECTION ( 'NONE',  ( -0.9876526153536342445, -0.1566598588826321470, 0.000000000000000000 ) ) ;
#1115=CARTESIAN_POINT ( 'NONE',  ( -59.83472345504510770, -87.44614099429799126, -12.99038105676658539 ) ) ;
#1116=VECTOR ( 'NONE', #4946, 1000.000000000000000 ) ;
#1117=ORIENTED_EDGE ( 'NONE', *, *, #3693, .T. ) ;
#1119=EDGE_CURVE ( 'NONE', #5250, #17961, #1414, .T. ) ;
#1120=ORIENTED_EDGE ( 'NONE', *, *, #2436, .T. ) ;
#1123=CARTESIAN_POINT ( 'NONE',  ( -57.85941822433786541, -87.13282127653273790, -12.99038105676658539 ) ) ;
#1125=ORIENTED_EDGE ( 'NONE', *, *, #15181, .T. ) ;
#1126=CARTESIAN_POINT ( 'NONE',  ( -11.76885329963143079, -17.05403346649147878, 4.330127018922214965 ) ) ;
#1127=AXIS2_PLACEMENT_3D ( 'NONE', #16323, #3218, #17682 ) ;
#1129=FACE_OUTER_BOUND ( 'NONE', #12163, .T. ) ;
#1131=CARTESIAN_POINT ( 'NONE',  ( 5.350349158294472218, -77.10659030804430358, -8.660254037844389075 ) ) ;
#1133=DIRECTION ( 'NONE',  ( -0.1566598588826321192, 0.9876526153536342445, 7.798540720466731404E-17 ) ) ;
#1134=CARTESIAN_POINT ( 'NONE',  ( -43.08426400421124924, -27.08374195694514341, 8.660254037844417496 ) ) ;
#1135=EDGE_LOOP ( 'NONE', ( #3407, #12333, #11137, #11919 ) ) ;
#1136=ORIENTED_EDGE ( 'NONE', *, *, #4437, .T. ) ;
#1138=DIRECTION ( 'NONE',  ( -0.1566598588826321192, 0.9876526153536342445, 7.798540720466730171E-17 ) ) ;
#1139=VERTEX_POINT ( 'NONE', #2826 ) ;
#1140=CIRCLE ( 'NONE', #2930, 1.500000000000000888 ) ;
#1141=CIRCLE ( 'NONE', #7183, 1.500000000000001332 ) ;
#1142=ADVANCED_FACE ( 'NONE', ( #1602 ), #8884, .F. ) ;
#1145=CIRCLE ( 'NONE', #17485, 1.499999999999999556 ) ;
#1146=CARTESIAN_POINT ( 'NONE',  ( -33.20773785067495965, -25.51714336811882688, 8.660254037844417496 ) ) ;
#1147=EDGE_CURVE ( 'NONE', #13568, #2699, #5943, .T. ) ;
#1148=CIRCLE ( 'NONE', #7487, 1.500000000000001332 ) ;
#1149=ORIENTED_EDGE ( 'NONE', *, *, #1553, .F. ) ;
#1152=DIRECTION ( 'NONE',  ( -0.000000000000000000, -0.000000000000000000, -1.000000000000000000 ) ) ;
#1154=ORIENTED_EDGE ( 'NONE', *, *, #12128, .F. ) ;
#1155=FACE_OUTER_BOUND ( 'NONE', #3199, .T. ) ;
#1156=CYLINDRICAL_SURFACE ( 'NONE', #8119, 1.500000000000000666 ) ;
#1157=CIRCLE ( 'NONE', #15972, 1.500000000000000444 ) ;
#1158=DIRECTION ( 'NONE',  ( -0.1566598588826321192, 0.9876526153536342445, 7.798540720466730171E-17 ) ) ;
#1159=DIRECTION ( 'NONE',  ( -0.1566598588826321747, 0.9876526153536343555, 0.000000000000000000 ) ) ;
#1163=ORIENTED_EDGE ( 'NONE', *, *, #18121, .F. ) ;
#1164=ORIENTED_EDGE ( 'NONE', *, *, #13310, .T. ) ;
#1166=EDGE_CURVE ( 'NONE', #17343, #6687, #1819, .T. ) ;
#1167=EDGE_LOOP ( 'NONE', ( #16777, #1534 ) ) ;
#1168=VERTEX_POINT ( 'NONE', #166 ) ;
#1169=DIRECTION ( 'NONE',  ( -0.1566598588826321192, 0.9876526153536342445, 7.798540720466731404E-17 ) ) ;
#1170=CIRCLE ( 'NONE', #9295, 2.000000000000000000 ) ;
#1171=FACE_BOUND ( 'NONE', #8973, .T. ) ;
#1172=EDGE_CURVE ( 'NONE', #8567, #13224, #4546, .T. ) ;
#1173=EDGE_LOOP ( 'NONE', ( #13695, #16928, #14846, #15179 ) ) ;
#1174=EDGE_LOOP ( 'NONE', ( #16625, #8138, #6275, #5012 ) ) ;
#1175=AXIS2_PLACEMENT_3D ( 'NONE', #12005, #6274, #12108 ) ;
#1176=ORIENTED_EDGE ( 'NONE', *, *, #5946, .T. ) ;
#1177=ORIENTED_EDGE ( 'NONE', *, *, #3923, .F. ) ;
#1178=AXIS2_PLACEMENT_3D ( 'NONE', #8807, #4352, #14496 ) ;
#1179=CYLINDRICAL_SURFACE ( 'NONE', #6081, 1.500000000000001554 ) ;
#1180=DIRECTION ( 'NONE',  ( -0.9876526153536341335, -0.1566598588826327021, 0.000000000000000000 ) ) ;
#1182=CIRCLE ( 'NONE', #3557, 1.500000000000000888 ) ;
#1183=CIRCLE ( 'NONE', #6002, 1.499999999999999556 ) ;
#1185=ORIENTED_EDGE ( 'NONE', *, *, #2912, .T. ) ;
#1186=EDGE_CURVE ( 'NONE', #4810, #886, #3031, .T. ) ;
#1187=ORIENTED_EDGE ( 'NONE', *, *, #13997, .T. ) ;
#1188=VERTEX_POINT ( 'NONE', #12474 ) ;
#1189=ORIENTED_EDGE ( 'NONE', *, *, #11793, .T. ) ;
#1190=CARTESIAN_POINT ( 'NONE',  ( -4.361458684479201153, -15.87908452487173427, -17.32050807568878170 ) ) ;
#1191=EDGE_CURVE ( 'NONE', #14798, #6605, #10294, .T. ) ;
#1192=EDGE_CURVE ( 'NONE', #17282, #16734, #10892, .T. ) ;
#1193=ORIENTED_EDGE ( 'NONE', *, *, #1553, .T. ) ;
#1196=DIRECTION ( 'NONE',  ( -0.9876526153536336894, -0.1566598588826350336, 0.000000000000000000 ) ) ;
#1198=LINE ( 'NONE', #7160, #12742 ) ;
#1199=VECTOR ( 'NONE', #745, 1000.000000000000000 ) ;
#1200=AXIS2_PLACEMENT_3D ( 'NONE', #3723, #2696, #12829 ) ;
#1201=DIRECTION ( 'NONE',  ( -0.9876526153536336894, -0.1566598588826350336, 0.000000000000000000 ) ) ;
#1202=DIRECTION ( 'NONE',  ( -0.1566598588826321192, 0.9876526153536342445, 7.798540720466730171E-17 ) ) ;
#1204=FACE_OUTER_BOUND ( 'NONE', #1787, .T. ) ;
#1205=DIRECTION ( 'NONE',  ( 0.000000000000000000, 0.000000000000000000, 1.000000000000000000 ) ) ;
#1206=VECTOR ( 'NONE', #10253, 1000.000000000000000 ) ;
#1207=CYLINDRICAL_SURFACE ( 'NONE', #7138, 1.500000000000000666 ) ;
#1208=ORIENTED_EDGE ( 'NONE', *, *, #2727, .F. ) ;
#1209=VERTEX_POINT ( 'NONE', #3546 ) ;
#1210=CARTESIAN_POINT ( 'NONE',  ( -16.91146969734005268, -22.93225569655540141, -17.32050807568878170 ) ) ;
#1211=CYLINDRICAL_SURFACE ( 'NONE', #2072, 20.00000000000001066 ) ;
#1212=DIRECTION ( 'NONE',  ( -0.1566598588826321192, 0.9876526153536342445, 7.798540720466730171E-17 ) ) ;
#1213=AXIS2_PLACEMENT_3D ( 'NONE', #10785, #16709, #13826 ) ;
#1214=EDGE_CURVE ( 'NONE', #13600, #3308, #2125, .T. ) ;
#1216=AXIS2_PLACEMENT_3D ( 'NONE', #2129, #13678, #3527 ) ;
#1217=ORIENTED_EDGE ( 'NONE', *, *, #18525, .F. ) ;
#1219=DIRECTION ( 'NONE',  ( -0.9876526153536341335, -0.1566598588826327021, 0.000000000000000000 ) ) ;
#1221=AXIS2_PLACEMENT_3D ( 'NONE', #5833, #7158, #8480 ) ;
#1223=EDGE_CURVE ( 'NONE', #12973, #12986, #9398, .T. ) ;
#1224=DIRECTION ( 'NONE',  ( -0.9876526153536341335, -0.1566598588826327021, 0.000000000000000000 ) ) ;
#1225=VECTOR ( 'NONE', #12033, 1000.000000000000000 ) ;
#1226=CARTESIAN_POINT ( 'NONE',  ( -10.98555400521827607, -21.99229654325962002, 4.330127018922214077 ) ) ;
#1228=DIRECTION ( 'NONE',  ( -0.9876526153536336894, -0.1566598588826349503, 0.000000000000000000 ) ) ;
#1229=CIRCLE ( 'NONE', #15424, 1.500000000000000888 ) ;
#1230=CARTESIAN_POINT ( 'NONE',  ( -83.14047854185180597, 6.938893903907228378E-15, 25.00000000000002132 ) ) ;
#1231=LINE ( 'NONE', #7109, #13735 ) ;
#1232=DIRECTION ( 'NONE',  ( -0.1566598588826321747, 0.9876526153536343555, 0.000000000000000000 ) ) ;
#1233=VERTEX_POINT ( 'NONE', #9452 ) ;
#1234=DIRECTION ( 'NONE',  ( 0.9876526153536341335, -0.1566598588826326743, 0.000000000000000000 ) ) ;
#1236=DIRECTION ( 'NONE',  ( -0.1566598588826321192, 0.9876526153536342445, 7.798540720466730171E-17 ) ) ;
#1239=CARTESIAN_POINT ( 'NONE',  ( -43.08426400421126345, -27.08374195694514341, -8.660254037844380193 ) ) ;
#1240=CIRCLE ( 'NONE', #3302, 1.500000000000001332 ) ;
#1242=CIRCLE ( 'NONE', #3928, 1.500000000000000000 ) ;
#1243=DIRECTION ( 'NONE',  ( -0.1566598588826321192, 0.9876526153536342445, 7.798540720466730171E-17 ) ) ;
#1244=EDGE_CURVE ( 'NONE', #403, #16695, #13918, .T. ) ;
#1246=EDGE_CURVE ( 'NONE', #4660, #13845, #12174, .T. ) ;
#1248=DIRECTION ( 'NONE',  ( -0.9876526153536341335, -0.1566598588826327021, 0.000000000000000000 ) ) ;
#1249=DIRECTION ( 'NONE',  ( -0.1566598588826321192, 0.9876526153536342445, 7.798540720466730171E-17 ) ) ;
#1250=AXIS2_PLACEMENT_3D ( 'NONE', #12266, #18216, #3736 ) ;
#1251=ADVANCED_FACE ( 'NONE', ( #2439 ), #8122, .F. ) ;
#1252=DIRECTION ( 'NONE',  ( -0.9876526153536336894, -0.1566598588826350336, 0.000000000000000000 ) ) ;
#1253=DIRECTION ( 'NONE',  ( -0.9876526153536336894, -0.1566598588826350336, 0.000000000000000000 ) ) ;
#1254=AXIS2_PLACEMENT_3D ( 'NONE', #14338, #15644, #15845 ) ;
#1257=AXIS2_PLACEMENT_3D ( 'NONE', #12290, #9196, #14966 ) ;
#1259=AXIS2_PLACEMENT_3D ( 'NONE', #4319, #2972, #15878 ) ;
#1260=EDGE_LOOP ( 'NONE', ( #9417, #10495, #17087, #8009 ) ) ;
#1261=EDGE_LOOP ( 'NONE', ( #16723, #9900, #18731, #3471, #10997, #3485 ) ) ;
#1263=VERTEX_POINT ( 'NONE', #9253 ) ;
#1264=VERTEX_POINT ( 'NONE', #7940 ) ;
#1265=VERTEX_POINT ( 'NONE', #18401 ) ;
#1266=CIRCLE ( 'NONE', #12101, 2.000000000000000000 ) ;
#1267=VERTEX_POINT ( 'NONE', #12552 ) ;
#1268=FACE_OUTER_BOUND ( 'NONE', #14639, .T. ) ;
#1269=CIRCLE ( 'NONE', #13322, 1.500000000000000444 ) ;
#1270=CARTESIAN_POINT ( 'NONE',  ( -24.27922930231443743, -81.80638607452326028, -8.660254037844385522 ) ) ;
#1271=CARTESIAN_POINT ( 'NONE',  ( -23.12685837619818940, -18.85562184364173888, -12.99038105676658006 ) ) ;
#1273=ADVANCED_FACE ( 'NONE', ( #6720 ), #18309, .F. ) ;
#1277=CIRCLE ( 'NONE', #11817, 1.500000000000000888 ) ;
#1278=CARTESIAN_POINT ( 'NONE',  ( -1.069392841504132052, -78.12487939078141608, 1.077796531449093893E-14 ) ) ;
#1279=CARTESIAN_POINT ( 'NONE',  ( -5.349111299832828514, -16.03574438375436984, -4.330127018922183879 ) ) ;
#1281=ADVANCED_FACE ( 'NONE', ( #16473 ), #649, .F. ) ;
#1282=FACE_BOUND ( 'NONE', #11132, .T. ) ;
#1283=FACE_OUTER_BOUND ( 'NONE', #17126, .T. ) ;
#1284=AXIS2_PLACEMENT_3D ( 'NONE', #8706, #1338, #15827 ) ;
#1285=ORIENTED_EDGE ( 'NONE', *, *, #16091, .T. ) ;
#1288=EDGE_LOOP ( 'NONE', ( #2095, #8493, #3511, #9093 ) ) ;
#1289=CARTESIAN_POINT ( 'NONE',  ( 2.058283315319403783, -14.86079544213463066, -17.32050807568878170 ) ) ;
#1290=VECTOR ( 'NONE', #2283, 1000.000000000000000 ) ;
#1291=DIRECTION ( 'NONE',  ( -0.1566598588826321192, 0.9876526153536342445, 7.798540720466730171E-17 ) ) ;
#1292=EDGE_LOOP ( 'NONE', ( #10578, #3990 ) ) ;
#1293=AXIS2_PLACEMENT_3D ( 'NONE', #3370, #9175, #14945 ) ;
#1294=DIRECTION ( 'NONE',  ( 1.000000000000000000, 0.000000000000000000, 0.000000000000000000 ) ) ;
#1296=AXIS2_PLACEMENT_3D ( 'NONE', #1979, #17943, #8906 ) ;
#1297=EDGE_CURVE ( 'NONE', #6069, #14627, #17290, .T. ) ;
#1298=EDGE_CURVE ( 'NONE', #5533, #356, #10749, .T. ) ;
#1300=DIRECTION ( 'NONE',  ( 0.000000000000000000, 0.000000000000000000, 1.000000000000000000 ) ) ;
#1301=CARTESIAN_POINT ( 'NONE',  ( -0.9046745307415022808, -15.33077501878252136, 17.32050807568881012 ) ) ;
#1302=ADVANCED_FACE ( 'NONE', ( #6615 ), #5188, .F. ) ;
#1304=ORIENTED_EDGE ( 'NONE', *, *, #16796, .T. ) ;
#1305=EDGE_LOOP ( 'NONE', ( #4565, #16384, #1189, #9828 ) ) ;
#1306=CARTESIAN_POINT ( 'NONE',  ( -69.25705831108246002, -31.23522821733487476, 1.869203119972154228E-14 ) ) ;
#1308=FACE_OUTER_BOUND ( 'NONE', #11877, .T. ) ;
#1310=ORIENTED_EDGE ( 'NONE', *, *, #3150, .F. ) ;
#1313=CARTESIAN_POINT ( 'NONE',  ( -61.35583738825340561, -29.98194934627382224, 1.887572821959364500E-14 ) ) ;
#1314=VERTEX_POINT ( 'NONE', #6522 ) ;
#1315=CARTESIAN_POINT ( 'NONE',  ( -40.61513246582718040, -26.69209230973856251, 4.330127018922217630 ) ) ;
#1316=DIRECTION ( 'NONE',  ( -0.000000000000000000, -0.000000000000000000, -1.000000000000000000 ) ) ;
#1318=ORIENTED_EDGE ( 'NONE', *, *, #11898, .T. ) ;
#1319=EDGE_CURVE ( 'NONE', #2695, #14517, #15220, .T. ) ;
#1320=CIRCLE ( 'NONE', #17676, 1.500000000000000888 ) ;
#1321=DIRECTION ( 'NONE',  ( -0.9876526153536336894, -0.1566598588826349503, 0.000000000000000000 ) ) ;
#1322=CARTESIAN_POINT ( 'NONE',  ( -20.82244514857674389, -81.25807656843406335, 17.32050807568881368 ) ) ;
#1323=LINE ( 'NONE', #14293, #16494 ) ;
#1324=DIRECTION ( 'NONE',  ( -0.1566598588826321192, 0.9876526153536342445, 7.798540720466730171E-17 ) ) ;
#1326=VERTEX_POINT ( 'NONE', #17336 ) ;
#1327=ADVANCED_FACE ( 'NONE', ( #12844 ), #15591, .F. ) ;
#1328=CARTESIAN_POINT ( 'NONE',  ( -33.16810284049710589, -83.21632480446696434, 4.330127018922213189 ) ) ;
#1329=ORIENTED_EDGE ( 'NONE', *, *, #690, .T. ) ;
#1330=EDGE_CURVE ( 'NONE', #4398, #10018, #12723, .T. ) ;
#1332=DIRECTION ( 'NONE',  ( -0.9876526153536336894, -0.1566598588826349503, 0.000000000000000000 ) ) ;
#1333=ORIENTED_EDGE ( 'NONE', *, *, #13285, .T. ) ;
#1335=DIRECTION ( 'NONE',  ( -0.9876526153536341335, -0.1566598588826327021, 0.000000000000000000 ) ) ;
#1336=DIRECTION ( 'NONE',  ( -0.1566598588826321192, 0.9876526153536342445, 7.798540720466731404E-17 ) ) ;
#1338=DIRECTION ( 'NONE',  ( -0.1566598588826321747, 0.9876526153536343555, 0.000000000000000000 ) ) ;
#1343=FACE_BOUND ( 'NONE', #4982, .T. ) ;
#1345=CARTESIAN_POINT ( 'NONE',  ( -45.55339554259533230, -27.47539160415171722, -12.99038105676658006 ) ) ;
#1346=VECTOR ( 'NONE', #12553, 1000.000000000000000 ) ;
#1348=EDGE_LOOP ( 'NONE', ( #7266, #4707, #14572, #15451 ) ) ;
#1349=EDGE_CURVE ( 'NONE', #4102, #15920, #6693, .T. ) ;
#1350=EDGE_CURVE ( 'NONE', #16790, #17286, #5177, .T. ) ;
#1351=FACE_OUTER_BOUND ( 'NONE', #7199, .T. ) ;
#1352=ORIENTED_EDGE ( 'NONE', *, *, #4629, .T. ) ;
#1353=ORIENTED_EDGE ( 'NONE', *, *, #315, .F. ) ;
#1357=DIRECTION ( 'NONE',  ( -0.1566598588826321747, 0.9876526153536343555, 0.000000000000000000 ) ) ;
#1361=FACE_BOUND ( 'NONE', #17500, .T. ) ;
#1362=CARTESIAN_POINT ( 'NONE',  ( -20.32861884089991023, -81.17974663899271093, -21.65063509461098690 ) ) ;
#1365=FACE_OUTER_BOUND ( 'NONE', #18646, .T. ) ;
#1367=DIRECTION ( 'NONE',  ( -0.9876526153536341335, -0.1566598588826327021, 0.000000000000000000 ) ) ;
#1368=EDGE_LOOP ( 'NONE', ( #7951, #8946, #1833, #12084 ) ) ;
#1369=VERTEX_POINT ( 'NONE', #1398 ) ;
#1370=ORIENTED_EDGE ( 'NONE', *, *, #15991, .T. ) ;
#1372=EDGE_CURVE ( 'NONE', #2469, #4280, #4254, .T. ) ;
#1373=AXIS2_PLACEMENT_3D ( 'NONE', #9286, #3128, #11730 ) ;
#1374=FACE_BOUND ( 'NONE', #314, .T. ) ;
#1375=CYLINDRICAL_SURFACE ( 'NONE', #1221, 1.500000000000001554 ) ;
#1376=ORIENTED_EDGE ( 'NONE', *, *, #4127, .T. ) ;
#1377=EDGE_CURVE ( 'NONE', #14160, #10171, #17137, .T. ) ;
#1378=DIRECTION ( 'NONE',  ( -0.1566598588826321192, 0.9876526153536342445, 7.798540720466730171E-17 ) ) ;
#1379=ADVANCED_FACE ( 'NONE', ( #9748 ), #4322, .F. ) ;
#1380=FACE_OUTER_BOUND ( 'NONE', #4464, .T. ) ;
#1382=EDGE_LOOP ( 'NONE', ( #4177, #17416 ) ) ;
#1384=CARTESIAN_POINT ( 'NONE',  ( -79.23462711737164454, 33.01666666666666572, 35.00000000000000000 ) ) ;
#1386=FACE_OUTER_BOUND ( 'NONE', #16373, .T. ) ;
#1387=ORIENTED_EDGE ( 'NONE', *, *, #3448, .T. ) ;
#1388=ORIENTED_EDGE ( 'NONE', *, *, #7142, .T. ) ;
#1389=FACE_BOUND ( 'NONE', #17368, .T. ) ;
#1390=DIRECTION ( 'NONE',  ( -0.1566598588826321192, 0.9876526153536342445, 7.798540720466730171E-17 ) ) ;
#1391=CARTESIAN_POINT ( 'NONE',  ( -67.07739975943471222, -25.82698556391885347, -8.660254037844380193 ) ) ;
#1392=ORIENTED_EDGE ( 'NONE', *, *, #17578, .F. ) ;
#1394=EDGE_CURVE ( 'NONE', #2218, #14954, #1266, .T. ) ;
#1395=CIRCLE ( 'NONE', #176, 1.500000000000000888 ) ;
#1396=DIRECTION ( 'NONE',  ( -0.1566598588826321747, 0.9876526153536343555, 0.000000000000000000 ) ) ;
#1398=CARTESIAN_POINT ( 'NONE',  ( -69.54653129781877396, -26.21863521112543793, 4.330127018922218518 ) ) ;
#1399=DIRECTION ( 'NONE',  ( 0.000000000000000000, 0.000000000000000000, 1.000000000000000000 ) ) ;
#1400=DIRECTION ( 'NONE',  ( 0.9876526153536342445, 0.1566598588826321470, 0.000000000000000000 ) ) ;
#1401=CIRCLE ( 'NONE', #5634, 1.500000000000000000 ) ;
#1402=DIRECTION ( 'NONE',  ( -0.9876526153536341335, -0.1566598588826327021, 0.000000000000000000 ) ) ;
#1403=ORIENTED_EDGE ( 'NONE', *, *, #6674, .F. ) ;
#1404=DIRECTION ( 'NONE',  ( -0.9876526153536336894, -0.1566598588826349503, 0.000000000000000000 ) ) ;
#1406=DIRECTION ( 'NONE',  ( -0.1566598588826321192, 0.9876526153536342445, 7.798540720466730171E-17 ) ) ;
#1407=ORIENTED_EDGE ( 'NONE', *, *, #18253, .F. ) ;
#1408=CARTESIAN_POINT ( 'NONE',  ( -60.36818477289978091, -29.82528948739120267, -21.65063509461098334 ) ) ;
#1411=EDGE_CURVE ( 'NONE', #13426, #11861, #9725, .T. ) ;
#1412=ORIENTED_EDGE ( 'NONE', *, *, #10407, .F. ) ;
#1413=DIRECTION ( 'NONE',  ( -0.9876526153536341335, -0.1566598588826327576, 0.000000000000000000 ) ) ;
#1414=LINE ( 'NONE', #12945, #627 ) ;
#1415=VERTEX_POINT ( 'NONE', #14181 ) ;
#1416=EDGE_LOOP ( 'NONE', ( #18088, #13081 ) ) ;
#1418=ADVANCED_FACE ( 'NONE', ( #14734 ), #10459, .F. ) ;
#1419=EDGE_CURVE ( 'NONE', #7156, #16655, #7895, .T. ) ;
#1420=CIRCLE ( 'NONE', #11676, 1.500000000000000888 ) ;
#1421=LINE ( 'NONE', #7117, #670 ) ;
#1422=CARTESIAN_POINT ( 'NONE',  ( -33.99103714508810725, -20.57888029135069274, 1.908195823574487804E-14 ) ) ;
#1423=CARTESIAN_POINT ( 'NONE',  ( -16.91146969734005268, -22.93225569655540141, 17.32050807568881012 ) ) ;
#1424=VECTOR ( 'NONE', #5665, 1000.000000000000000 ) ;
#1425=DIRECTION ( 'NONE',  ( -0.9876526153536341335, -0.1566598588826327021, 0.000000000000000000 ) ) ;
#1426=DIRECTION ( 'NONE',  ( -0.1566598588826321192, 0.9876526153536342445, 7.798540720466730171E-17 ) ) ;
#1427=CARTESIAN_POINT ( 'NONE',  ( -61.31620237807555895, -87.68113078262194904, 4.330127018922213189 ) ) ;
#1429=CARTESIAN_POINT ( 'NONE',  ( -20.65772683781411345, -18.46397219643516152, -8.660254037844380193 ) ) ;
#1430=FACE_BOUND ( 'NONE', #6889, .T. ) ;
#1431=LINE ( 'NONE', #4433, #16913 ) ;
#1432=VECTOR ( 'NONE', #11631, 1000.000000000000000 ) ;
#1433=CARTESIAN_POINT ( 'NONE',  ( -68.55887868246516348, -26.06197535224280415, 8.660254037844417496 ) ) ;
#1434=ORIENTED_EDGE ( 'NONE', *, *, #11049, .T. ) ;
#1435=CARTESIAN_POINT ( 'NONE',  ( -2.590506774712417748, -20.66068774275724707, 4.330127018922212301 ) ) ;
#1436=VERTEX_POINT ( 'NONE', #16251 ) ;
#1437=CIRCLE ( 'NONE', #6282, 1.500000000000001332 ) ;
#1438=EDGE_LOOP ( 'NONE', ( #17360, #14146 ) ) ;
#1439=DIRECTION ( 'NONE',  ( -0.9876526153536336894, -0.1566598588826349503, 0.000000000000000000 ) ) ;
#1440=AXIS2_PLACEMENT_3D ( 'NONE', #10747, #3544, #16857 ) ;
#1441=FACE_BOUND ( 'NONE', #12061, .T. ) ;
#1442=CIRCLE ( 'NONE', #14123, 1.499999999999999556 ) ;
#1443=CARTESIAN_POINT ( 'NONE',  ( -25.80034323552273534, -24.34219442649909126, 21.65063509461101887 ) ) ;
#1444=EDGE_CURVE ( 'NONE', #11927, #13075, #13931, .T. ) ;
#1446=EDGE_CURVE ( 'NONE', #13518, #9479, #18546, .T. ) ;
#1447=AXIS2_PLACEMENT_3D ( 'NONE', #18670, #137, #1205 ) ;
#1448=CIRCLE ( 'NONE', #18120, 1.500000000000001332 ) ;
#1449=CARTESIAN_POINT ( 'NONE',  ( -52.75643683680706886, -23.55541761012069912, 12.99038105676661736 ) ) ;
#1450=DIRECTION ( 'NONE',  ( -0.1566598588826321747, 0.9876526153536343555, 0.000000000000000000 ) ) ;
#1451=DIRECTION ( 'NONE',  ( -0.1566598588826321192, 0.9876526153536342445, 7.798540720466730171E-17 ) ) ;
#1452=FACE_BOUND ( 'NONE', #7236, .T. ) ;
#1453=CARTESIAN_POINT ( 'NONE',  ( -63.62061560569701157, -25.27867605782964233, 1.908195823574487804E-14 ) ) ;
#1454=ORIENTED_EDGE ( 'NONE', *, *, #1350, .T. ) ;
#1456=VERTEX_POINT ( 'NONE', #11600 ) ;
#1457=VERTEX_POINT ( 'NONE', #3078 ) ;
#1458=DIRECTION ( 'NONE',  ( -0.9876526153536341335, -0.1566598588826327021, 0.000000000000000000 ) ) ;
#1459=VERTEX_POINT ( 'NONE', #17619 ) ;
#1460=DIRECTION ( 'NONE',  ( -0.1566598588826321192, 0.9876526153536342445, 7.798540720466730171E-17 ) ) ;
#1461=AXIS2_PLACEMENT_3D ( 'NONE', #12294, #7961, #14881 ) ;
#1462=DIRECTION ( 'NONE',  ( 2.887450008416415878E-16, 0.000000000000000000, 1.000000000000000000 ) ) ;
#1463=ORIENTED_EDGE ( 'NONE', *, *, #11826, .F. ) ;
#1464=LINE ( 'NONE', #11580, #10011 ) ;
#1465=EDGE_CURVE ( 'NONE', #5203, #17378, #14844, .T. ) ;
#1466=AXIS2_PLACEMENT_3D ( 'NONE', #18717, #11166, #16991 ) ;
#1467=DIRECTION ( 'NONE',  ( -0.9876526153536341335, 0.1566598588826326743, 2.851797552515345870E-16 ) ) ;
#1468=LINE ( 'NONE', #11581, #8547 ) ;
#1470=CIRCLE ( 'NONE', #14176, 1.500000000000001332 ) ;
#1471=EDGE_CURVE ( 'NONE', #4101, #8059, #13631, .T. ) ;
#1472=DIRECTION ( 'NONE',  ( -0.9876526153536336894, -0.1566598588826349503, 0.000000000000000000 ) ) ;
#1477=VERTEX_POINT ( 'NONE', #10557 ) ;
#1478=CARTESIAN_POINT ( 'NONE',  ( -36.62488699423479943, -83.76463431055617548, 21.65063509461101532 ) ) ;
#1479=CARTESIAN_POINT ( 'NONE',  ( -17.85948730251583783, -80.78809699178616199, 17.32050807568881368 ) ) ;
#1480=EDGE_CURVE ( 'NONE', #5250, #15378, #9096, .T. ) ;
#1481=DIRECTION ( 'NONE',  ( 0.9876526153536342445, 0.1566598588826321470, 0.000000000000000000 ) ) ;
#1482=ORIENTED_EDGE ( 'NONE', *, *, #2611, .F. ) ;
#1484=DIRECTION ( 'NONE',  ( -0.1566598588826321192, 0.9876526153536342445, 7.798540720466730171E-17 ) ) ;
#1486=EDGE_LOOP ( 'NONE', ( #6896, #992 ) ) ;
#1488=CIRCLE ( 'NONE', #8142, 1.500000000000000888 ) ;
#1489=VECTOR ( 'NONE', #5333, 1000.000000000000000 ) ;
#1490=DIRECTION ( 'NONE',  ( 0.000000000000000000, 0.000000000000000000, 1.000000000000000000 ) ) ;
#1491=CARTESIAN_POINT ( 'NONE',  ( -58.68235252892885256, -24.49537676341648762, 8.660254037844417496 ) ) ;
#1492=DIRECTION ( 'NONE',  ( -1.000000000000000000, 0.000000000000000000, 0.000000000000000000 ) ) ;
#1495=FACE_OUTER_BOUND ( 'NONE', #799, .T. ) ;
#1496=CIRCLE ( 'NONE', #3568, 1.500000000000000888 ) ;
#1497=DIRECTION ( 'NONE',  ( -0.1566598588826321192, 0.9876526153536342445, 7.798540720466730171E-17 ) ) ;
#1498=LINE ( 'NONE', #13038, #17120 ) ;
#1499=CIRCLE ( 'NONE', #16019, 1.500000000000000888 ) ;
#1500=ORIENTED_EDGE ( 'NONE', *, *, #14501, .F. ) ;
#1501=DIRECTION ( 'NONE',  ( -0.9876526153536341335, -0.1566598588826327021, 0.000000000000000000 ) ) ;
#1502=AXIS2_PLACEMENT_3D ( 'NONE', #17737, #4711, #268 ) ;
#1503=LINE ( 'NONE', #79, #9060 ) ;
#1504=EDGE_LOOP ( 'NONE', ( #15054, #14543, #13451, #4712 ) ) ;
#1505=EDGE_CURVE ( 'NONE', #12166, #3971, #8871, .T. ) ;
#1506=VERTEX_POINT ( 'NONE', #6219 ) ;
#1507=CYLINDRICAL_SURFACE ( 'NONE', #318, 1.500000000000001554 ) ;
#1508=ORIENTED_EDGE ( 'NONE', *, *, #17437, .T. ) ;
#1509=CIRCLE ( 'NONE', #599, 1.500000000000000888 ) ;
#1510=AXIS2_PLACEMENT_3D ( 'NONE', #7878, #10979, #7968 ) ;
#1511=DIRECTION ( 'NONE',  ( -0.000000000000000000, -0.000000000000000000, -1.000000000000000000 ) ) ;
#1512=ORIENTED_EDGE ( 'NONE', *, *, #14379, .F. ) ;
#1514=DIRECTION ( 'NONE',  ( 0.000000000000000000, 0.000000000000000000, 1.000000000000000000 ) ) ;
#1516=AXIS2_PLACEMENT_3D ( 'NONE', #17367, #14497, #8629 ) ;
#1517=CARTESIAN_POINT ( 'NONE',  ( -52.96079015774756016, -28.65034054577145994, 1.869203119972154228E-14 ) ) ;
#1518=LINE ( 'NONE', #10207, #13241 ) ;
#1520=DIRECTION ( 'NONE',  ( -0.1566598588826321192, 0.9876526153536342445, 7.798540720466731404E-17 ) ) ;
#1521=FACE_BOUND ( 'NONE', #3260, .T. ) ;
#1522=EDGE_CURVE ( 'NONE', #334, #10470, #16170, .T. ) ;
#1524=EDGE_CURVE ( 'NONE', #15683, #6731, #16690, .T. ) ;
#1528=AXIS2_PLACEMENT_3D ( 'NONE', #12056, #1946, #15210 ) ;
#1529=ORIENTED_EDGE ( 'NONE', *, *, #4633, .T. ) ;
#1530=DIRECTION ( 'NONE',  ( -0.9876526153536336894, -0.1566598588826349503, 0.000000000000000000 ) ) ;
#1531=AXIS2_PLACEMENT_3D ( 'NONE', #6549, #3301, #3484 ) ;
#1532=VERTEX_POINT ( 'NONE', #9047 ) ;
#1534=ORIENTED_EDGE ( 'NONE', *, *, #13160, .T. ) ;
#1535=DIRECTION ( 'NONE',  ( -0.1566598588826321747, 0.9876526153536343555, 0.000000000000000000 ) ) ;
#1536=FACE_BOUND ( 'NONE', #12481, .T. ) ;
#1537=ORIENTED_EDGE ( 'NONE', *, *, #16319, .T. ) ;
#1538=CIRCLE ( 'NONE', #934, 1.500000000000000444 ) ;
#1540=AXIS2_PLACEMENT_3D ( 'NONE', #16573, #9359, #6250 ) ;
#1541=VERTEX_POINT ( 'NONE', #14831 ) ;
#1544=VECTOR ( 'NONE', #5102, 1000.000000000000000 ) ;
#1545=VERTEX_POINT ( 'NONE', #11948 ) ;
#1547=DIRECTION ( 'NONE',  ( -0.9876526153536341335, -0.1566598588826327576, 0.000000000000000000 ) ) ;
#1548=CARTESIAN_POINT ( 'NONE',  ( -74.19532138785061193, -32.01852751174804013, 8.660254037844417496 ) ) ;
#1550=CARTESIAN_POINT ( 'NONE',  ( -18.39294862037050393, -23.16724548487935564, -17.32050807568878170 ) ) ;
#1551=FACE_BOUND ( 'NONE', #18483, .T. ) ;
#1552=CYLINDRICAL_SURFACE ( 'NONE', #8140, 1.500000000000001554 ) ;
#1553=EDGE_CURVE ( 'NONE', #16881, #10372, #336, .T. ) ;
#1554=AXIS2_PLACEMENT_3D ( 'NONE', #8106, #14169, #3636 ) ;
#1555=ADVANCED_FACE ( 'NONE', ( #628 ), #9428, .F. ) ;
#1557=ADVANCED_FACE ( 'NONE', ( #12335 ), #2303, .F. ) ;
#1558=EDGE_CURVE ( 'NONE', #11543, #3425, #11501, .T. ) ;
#1559=ORIENTED_EDGE ( 'NONE', *, *, #357, .F. ) ;
#1560=ORIENTED_EDGE ( 'NONE', *, *, #18525, .T. ) ;
#1561=LINE ( 'NONE', #2786, #13648 ) ;
#1562=ORIENTED_EDGE ( 'NONE', *, *, #7966, .T. ) ;
#1563=CARTESIAN_POINT ( 'NONE',  ( -64.60826822105063627, -25.43533591671227612, -4.330127018922180326 ) ) ;
#1564=LINE ( 'NONE', #7076, #5742 ) ;
#1565=VERTEX_POINT ( 'NONE', #8196 ) ;
#1567=AXIS2_PLACEMENT_3D ( 'NONE', #14048, #1096, #6868 ) ;
#1568=DIRECTION ( 'NONE',  ( -0.1566598588826321747, 0.9876526153536343555, 0.000000000000000000 ) ) ;
#1569=DIRECTION ( 'NONE',  ( -0.1566598588826321192, 0.9876526153536342445, 7.798540720466730171E-17 ) ) ;
#1570=VECTOR ( 'NONE', #2588, 1000.000000000000000 ) ;
#1572=ORIENTED_EDGE ( 'NONE', *, *, #15226, .T. ) ;
#1573=ORIENTED_EDGE ( 'NONE', *, *, #9814, .F. ) ;
#1574=FACE_BOUND ( 'NONE', #11405, .T. ) ;
#1575=CARTESIAN_POINT ( 'NONE',  ( -29.21749237908258223, -82.58968536893640078, 7.308518362537324739E-15 ) ) ;
#1576=EDGE_CURVE ( 'NONE', #16216, #9221, #5161, .T. ) ;
#1577=AXIS2_PLACEMENT_3D ( 'NONE', #8249, #16791, #3950 ) ;
#1578=CARTESIAN_POINT ( 'NONE',  ( -11.76885329963143434, -17.05403346649147522, -21.65063509461097979 ) ) ;
#1579=AXIS2_PLACEMENT_3D ( 'NONE', #972, #5309, #15450 ) ;
#1580=EDGE_CURVE ( 'NONE', #10670, #15897, #9999, .T. ) ;
#1581=EDGE_LOOP ( 'NONE', ( #11529, #12659 ) ) ;
#1582=DIRECTION ( 'NONE',  ( -0.1566598588826321192, 0.9876526153536342445, 7.798540720466731404E-17 ) ) ;
#1583=AXIS2_PLACEMENT_3D ( 'NONE', #6546, #10874, #3480 ) ;
#1584=ADVANCED_FACE ( 'NONE', ( #17988 ), #10924, .F. ) ;
#1585=CIRCLE ( 'NONE', #12135, 1.500000000000000888 ) ;
#1586=DIRECTION ( 'NONE',  ( 1.000000000000000000, 0.000000000000000000, -3.469446951953612217E-16 ) ) ;
#1588=FACE_OUTER_BOUND ( 'NONE', #9304, .T. ) ;
#1590=AXIS2_PLACEMENT_3D ( 'NONE', #10536, #7896, #8645 ) ;
#1591=DIRECTION ( 'NONE',  ( -0.1566598588826321192, 0.9876526153536342445, 7.798540720466730171E-17 ) ) ;
#1592=CARTESIAN_POINT ( 'NONE',  ( -13.41505053342451426, -80.08312762681433128, 4.330127018922213189 ) ) ;
#1593=LINE ( 'NONE', #15980, #752 ) ;
#1594=DIRECTION ( 'NONE',  ( -0.9876526153536341335, -0.1566598588826327021, 0.000000000000000000 ) ) ;
#1595=VERTEX_POINT ( 'NONE', #12448 ) ;
#1596=ORIENTED_EDGE ( 'NONE', *, *, #1394, .F. ) ;
#1597=AXIS2_PLACEMENT_3D ( 'NONE', #17139, #9454, #8021 ) ;
#1598=CARTESIAN_POINT ( 'NONE',  ( -11.76885329963143434, -17.05403346649147878, -12.99038105676658006 ) ) ;
#1599=ORIENTED_EDGE ( 'NONE', *, *, #3502, .F. ) ;
#1601=VERTEX_POINT ( 'NONE', #6591 ) ;
#1602=FACE_OUTER_BOUND ( 'NONE', #1914, .T. ) ;
#1603=ORIENTED_EDGE ( 'NONE', *, *, #17001, .T. ) ;
#1604=ADVANCED_FACE ( 'NONE', ( #15387 ), #16745, .F. ) ;
#1605=DIRECTION ( 'NONE',  ( -0.1566598588826321192, 0.9876526153536342445, 7.798540720466731404E-17 ) ) ;
#1606=DIRECTION ( 'NONE',  ( -0.9876526153536336894, -0.1566598588826349503, 0.000000000000000000 ) ) ;
#1607=AXIS2_PLACEMENT_3D ( 'NONE', #15466, #12513, #1081 ) ;
#1608=DIRECTION ( 'NONE',  ( -0.1566598588826321192, 0.9876526153536342445, 7.798540720466731404E-17 ) ) ;
#1609=EDGE_LOOP ( 'NONE', ( #17915, #16603, #18471, #7883 ) ) ;
#1610=CARTESIAN_POINT ( 'NONE',  ( -24.31886431249228053, -24.10720463817513703, -12.99038105676658006 ) ) ;
#1611=CARTESIAN_POINT ( 'NONE',  ( 0.000000000000000000, 0.000000000000000000, -24.99999999999999289 ) ) ;
#1612=EDGE_CURVE ( 'NONE', #5465, #1095, #15462, .T. ) ;
#1613=DIRECTION ( 'NONE',  ( -0.1566598588826321747, 0.9876526153536343555, 0.000000000000000000 ) ) ;
#1617=VERTEX_POINT ( 'NONE', #11009 ) ;
#1618=ORIENTED_EDGE ( 'NONE', *, *, #3328, .F. ) ;
#1620=CIRCLE ( 'NONE', #10963, 1.500000000000000888 ) ;
#1621=VERTEX_POINT ( 'NONE', #18288 ) ;
#1625=LINE ( 'NONE', #4721, #2484 ) ;
#1626=ORIENTED_EDGE ( 'NONE', *, *, #6874, .F. ) ;
#1630=ADVANCED_FACE ( 'NONE', ( #18187 ), #2032, .F. ) ;
#1631=CIRCLE ( 'NONE', #13707, 1.500000000000001332 ) ;
#1633=VERTEX_POINT ( 'NONE', #2220 ) ;
#1634=FACE_BOUND ( 'NONE', #13474, .T. ) ;
#1635=ORIENTED_EDGE ( 'NONE', *, *, #118, .T. ) ;
#1636=CYLINDRICAL_SURFACE ( 'NONE', #3035, 1.500000000000001554 ) ;
#1637=CARTESIAN_POINT ( 'NONE',  ( -48.80582637539256297, -22.92877817459016399, -8.660254037844380193 ) ) ;
#1638=CARTESIAN_POINT ( 'NONE',  ( 5.350349158294472218, -77.10659030804430358, 8.660254037844406838 ) ) ;
#1639=DIRECTION ( 'NONE',  ( -0.9876526153536336894, -0.1566598588826349503, 0.000000000000000000 ) ) ;
#1640=ORIENTED_EDGE ( 'NONE', *, *, #1083, .F. ) ;
#1641=VERTEX_POINT ( 'NONE', #721 ) ;
#1643=VERTEX_POINT ( 'NONE', #6500 ) ;
#1644=DIRECTION ( 'NONE',  ( -0.9876526153536336894, -0.1566598588826349503, 0.000000000000000000 ) ) ;
#1645=ORIENTED_EDGE ( 'NONE', *, *, #17724, .F. ) ;
#1647=EDGE_CURVE ( 'NONE', #6106, #13454, #10921, .T. ) ;
#1648=FACE_OUTER_BOUND ( 'NONE', #12631, .T. ) ;
#1649=EDGE_CURVE ( 'NONE', #9534, #3195, #13965, .T. ) ;
#1650=ORIENTED_EDGE ( 'NONE', *, *, #15098, .T. ) ;
#1651=ORIENTED_EDGE ( 'NONE', *, *, #16533, .T. ) ;
#1652=ORIENTED_EDGE ( 'NONE', *, *, #6802, .F. ) ;
#1653=ADVANCED_FACE ( 'NONE', ( #3898 ), #2794, .F. ) ;
#1654=CARTESIAN_POINT ( 'NONE',  ( -60.16383145195931803, -24.73036655174043119, 1.908195823574487804E-14 ) ) ;
#1655=CARTESIAN_POINT ( 'NONE',  ( 3.231158466157540765, -19.73726462726228092, -24.99999999999998934 ) ) ;
#1657=EDGE_LOOP ( 'NONE', ( #9720, #10349, #3053, #17418 ) ) ;
#1658=ORIENTED_EDGE ( 'NONE', *, *, #1214, .F. ) ;
#1659=LINE ( 'NONE', #4766, #11138 ) ;
#1660=CIRCLE ( 'NONE', #12218, 1.500000000000000444 ) ;
#1661=CYLINDRICAL_SURFACE ( 'NONE', #8097, 1.500000000000001554 ) ;
#1662=VERTEX_POINT ( 'NONE', #2592 ) ;
#1663=DIRECTION ( 'NONE',  ( -0.9876526153536341335, -0.1566598588826327021, 0.000000000000000000 ) ) ;
#1664=DIRECTION ( 'NONE',  ( -0.1566598588826321192, 0.9876526153536342445, 7.798540720466730171E-17 ) ) ;
#1665=AXIS2_PLACEMENT_3D ( 'NONE', #9437, #728, #6510 ) ;
#1666=CARTESIAN_POINT ( 'NONE',  ( -33.20773785067495965, -25.51714336811882688, 17.32050807568881723 ) ) ;
#1667=EDGE_CURVE ( 'NONE', #7348, #1565, #5734, .T. ) ;
#1668=EDGE_LOOP ( 'NONE', ( #267, #12837, #12530, #9189 ) ) ;
#1669=ADVANCED_FACE ( 'NONE', ( #5443, #18376 ), #11388, .F. ) ;
#1670=CARTESIAN_POINT ( 'NONE',  ( -39.62747985047356281, -26.53543245085592517, -8.660254037844380193 ) ) ;
#1671=DIRECTION ( 'NONE',  ( -0.9876526153536336894, -0.1566598588826349503, 0.000000000000000000 ) ) ;
#1672=CYLINDRICAL_SURFACE ( 'NONE', #5958, 1.500000000000000888 ) ;
#1673=VERTEX_POINT ( 'NONE', #17213 ) ;
#1675=EDGE_CURVE ( 'NONE', #10299, #968, #15489, .T. ) ;
#1676=CARTESIAN_POINT ( 'NONE',  ( -88.82622559915370175, -29.27674910825304977, 25.00000000000001776 ) ) ;
#1678=ORIENTED_EDGE ( 'NONE', *, *, #11185, .T. ) ;
#1682=VERTEX_POINT ( 'NONE', #9803 ) ;
#1686=CARTESIAN_POINT ( 'NONE',  ( -56.37793930130741415, -86.89783148820879433, -4.330127018922185655 ) ) ;
#1688=DIRECTION ( 'NONE',  ( 0.000000000000000000, 0.000000000000000000, 1.000000000000000000 ) ) ;
#1689=CIRCLE ( 'NONE', #12259, 1.500000000000000444 ) ;
#1690=FACE_OUTER_BOUND ( 'NONE', #15751, .T. ) ;
#1691=FACE_BOUND ( 'NONE', #4055, .T. ) ;
#1692=CARTESIAN_POINT ( 'NONE',  ( -57.89905323451571206, -29.43363984018462176, -17.32050807568878170 ) ) ;
#1693=FACE_OUTER_BOUND ( 'NONE', #13800, .T. ) ;
#1694=EDGE_CURVE ( 'NONE', #7684, #18620, #1198, .T. ) ;
#1695=CARTESIAN_POINT ( 'NONE',  ( -46.33669483700847280, -22.53712852738359373, 12.99038105676661736 ) ) ;
#1696=LINE ( 'NONE', #14860, #7256 ) ;
#1697=ORIENTED_EDGE ( 'NONE', *, *, #12586, .T. ) ;
#1698=ORIENTED_EDGE ( 'NONE', *, *, #5305, .F. ) ;
#1699=CARTESIAN_POINT ( 'NONE',  ( -61.31620237807555895, -87.68113078262196325, 21.65063509461101532 ) ) ;
#1700=AXIS2_PLACEMENT_3D ( 'NONE', #9194, #15557, #11282 ) ;
#1702=EDGE_CURVE ( 'NONE', #18222, #2420, #15775, .T. ) ;
#1703=VERTEX_POINT ( 'NONE', #12904 ) ;
#1704=DIRECTION ( 'NONE',  ( -0.1566598588826321747, 0.9876526153536343555, 0.000000000000000000 ) ) ;
#1705=ORIENTED_EDGE ( 'NONE', *, *, #3696, .F. ) ;
#1708=CYLINDRICAL_SURFACE ( 'NONE', #2816, 1.500000000000001554 ) ;
#1710=DIRECTION ( 'NONE',  ( -0.1566598588826321192, 0.9876526153536342445, 7.798540720466731404E-17 ) ) ;
#1711=ORIENTED_EDGE ( 'NONE', *, *, #6359, .T. ) ;
#1712=LINE ( 'NONE', #16310, #5525 ) ;
#1713=ORIENTED_EDGE ( 'NONE', *, *, #7104, .T. ) ;
#1714=EDGE_CURVE ( 'NONE', #7134, #8567, #1464, .T. ) ;
#1715=DIRECTION ( 'NONE',  ( -0.1566598588826321747, 0.9876526153536343555, 0.000000000000000000 ) ) ;
#1716=CARTESIAN_POINT ( 'NONE',  ( -66.08974714408108753, -25.67032570503621969, -4.330127018922180326 ) ) ;
#1717=ORIENTED_EDGE ( 'NONE', *, *, #11760, .T. ) ;
#1721=CYLINDRICAL_SURFACE ( 'NONE', #18708, 1.500000000000001554 ) ;
#1722=VECTOR ( 'NONE', #14742, 1000.000000000000000 ) ;
#1723=AXIS2_PLACEMENT_3D ( 'NONE', #1795, #567, #17457 ) ;
#1724=FACE_BOUND ( 'NONE', #13194, .T. ) ;
#1725=DIRECTION ( 'NONE',  ( 0.000000000000000000, 0.000000000000000000, 1.000000000000000000 ) ) ;
#1728=ORIENTED_EDGE ( 'NONE', *, *, #16724, .T. ) ;
#1729=DIRECTION ( 'NONE',  ( -0.1566598588826321747, 0.9876526153536343555, 0.000000000000000000 ) ) ;
#1730=CIRCLE ( 'NONE', #12309, 1.500000000000000000 ) ;
#1731=DIRECTION ( 'NONE',  ( -0.1566598588826321192, 0.9876526153536342445, 7.798540720466731404E-17 ) ) ;
#1735=EDGE_CURVE ( 'NONE', #13724, #6259, #17627, .T. ) ;
#1736=DIRECTION ( 'NONE',  ( 0.000000000000000000, 0.000000000000000000, 1.000000000000000000 ) ) ;
#1737=ORIENTED_EDGE ( 'NONE', *, *, #17505, .F. ) ;
#1738=ORIENTED_EDGE ( 'NONE', *, *, #10215, .F. ) ;
#1739=DIRECTION ( 'NONE',  ( -0.1566598588826321192, 0.9876526153536342445, 7.798540720466730171E-17 ) ) ;
#1740=EDGE_CURVE ( 'NONE', #6097, #10127, #1277, .T. ) ;
#1741=LINE ( 'NONE', #13570, #3025 ) ;
#1743=ORIENTED_EDGE ( 'NONE', *, *, #15544, .F. ) ;
#1744=LINE ( 'NONE', #5844, #5974 ) ;
#1745=AXIS2_PLACEMENT_3D ( 'NONE', #12041, #16351, #3340 ) ;
#1746=CARTESIAN_POINT ( 'NONE',  ( -58.68235252892886678, -24.49537676341648051, -8.660254037844380193 ) ) ;
#1748=ORIENTED_EDGE ( 'NONE', *, *, #1904, .T. ) ;
#1749=CARTESIAN_POINT ( 'NONE',  ( 3.868870235264020963, -77.34158009636824715, -17.32050807568878525 ) ) ;
#1750=FACE_BOUND ( 'NONE', #7647, .T. ) ;
#1751=CARTESIAN_POINT ( 'NONE',  ( 0.000000000000000000, 0.000000000000000000, 24.99999999999999289 ) ) ;
#1752=AXIS2_PLACEMENT_3D ( 'NONE', #11601, #69, #14559 ) ;
#1753=DIRECTION ( 'NONE',  ( -0.1566598588826321192, 0.9876526153536342445, 7.798540720466731404E-17 ) ) ;
#1754=CIRCLE ( 'NONE', #546, 1.500000000000000888 ) ;
#1755=EDGE_LOOP ( 'NONE', ( #2947, #4083 ) ) ;
#1756=LINE ( 'NONE', #17246, #3586 ) ;
#1757=DIRECTION ( 'NONE',  ( -0.1566598588826321192, 0.9876526153536342445, 7.798540720466731404E-17 ) ) ;
#1758=DIRECTION ( 'NONE',  ( 0.000000000000000000, 0.000000000000000000, 1.000000000000000000 ) ) ;
#1759=EDGE_CURVE ( 'NONE', #10340, #4741, #6710, .T. ) ;
#1760=CYLINDRICAL_SURFACE ( 'NONE', #16250, 1.500000000000000888 ) ;
#1763=ORIENTED_EDGE ( 'NONE', *, *, #14939, .T. ) ;
#1764=AXIS2_PLACEMENT_3D ( 'NONE', #13358, #17755, #4728 ) ;
#1766=ORIENTED_EDGE ( 'NONE', *, *, #6857, .F. ) ;
#1767=EDGE_CURVE ( 'NONE', #11126, #13246, #17317, .T. ) ;
#1768=AXIS2_PLACEMENT_3D ( 'NONE', #17362, #4347, #18627 ) ;
#1769=EDGE_LOOP ( 'NONE', ( #14744, #11820 ) ) ;
#1773=CARTESIAN_POINT ( 'NONE',  ( -81.73462711737164454, 33.01666666666666572, -30.00000000000000000 ) ) ;
#1774=DIRECTION ( 'NONE',  ( -0.1566598588826321192, 0.9876526153536342445, 7.798540720466730171E-17 ) ) ;
#1775=CIRCLE ( 'NONE', #12351, 1.499999999999999556 ) ;
#1776=ORIENTED_EDGE ( 'NONE', *, *, #5784, .F. ) ;
#1777=DIRECTION ( 'NONE',  ( -0.1566598588826321192, 0.9876526153536342445, 7.798540720466730171E-17 ) ) ;
#1778=DIRECTION ( 'NONE',  ( -0.1566598588826321192, 0.9876526153536342445, 7.798540720466730171E-17 ) ) ;
#1779=EDGE_LOOP ( 'NONE', ( #5664, #8692, #1990, #11428 ) ) ;
#1781=DIRECTION ( 'NONE',  ( 0.000000000000000000, 0.000000000000000000, 1.000000000000000000 ) ) ;
#1782=CIRCLE ( 'NONE', #9962, 1.500000000000000444 ) ;
#1784=CARTESIAN_POINT ( 'NONE',  ( -30.04042668367358360, -19.95224085582016471, -12.99038105676658006 ) ) ;
#1785=VERTEX_POINT ( 'NONE', #5591 ) ;
#1786=CARTESIAN_POINT ( 'NONE',  ( -4.565812005419673802, -20.97400746052251108, -4.330127018922184767 ) ) ;
#1787=EDGE_LOOP ( 'NONE', ( #7734, #9700, #6659, #13001 ) ) ;
#1788=VECTOR ( 'NONE', #8869, 1000.000000000000000 ) ;
#1789=EDGE_LOOP ( 'NONE', ( #18449, #5393, #112, #10399 ) ) ;
#1790=DIRECTION ( 'NONE',  ( -0.1566598588826321747, 0.9876526153536343555, 0.000000000000000000 ) ) ;
#1791=AXIS2_PLACEMENT_3D ( 'NONE', #17285, #2759, #5605 ) ;
#1794=ORIENTED_EDGE ( 'NONE', *, *, #18353, .F. ) ;
#1795=CARTESIAN_POINT ( 'NONE',  ( -30.73860631229088369, -25.12549372091224598, 4.330127018922217630 ) ) ;
#1796=AXIS2_PLACEMENT_3D ( 'NONE', #14290, #6726, #1321 ) ;
#1798=AXIS2_PLACEMENT_3D ( 'NONE', #3437, #9328, #11950 ) ;
#1799=AXIS2_PLACEMENT_3D ( 'NONE', #5863, #17431, #4418 ) ;
#1800=VECTOR ( 'NONE', #10558, 1000.000000000000000 ) ;
#1802=VERTEX_POINT ( 'NONE', #10203 ) ;
#1803=ADVANCED_FACE ( 'NONE', ( #11255 ), #10027, .F. ) ;
#1804=DIRECTION ( 'NONE',  ( -0.1566598588826321192, 0.9876526153536342445, 7.798540720466730171E-17 ) ) ;
#1805=AXIS2_PLACEMENT_3D ( 'NONE', #11229, #7005, #3925 ) ;
#1806=CARTESIAN_POINT ( 'NONE',  ( -67.77557938805200877, -31.00023842901093118, 8.660254037844417496 ) ) ;
#1807=AXIS2_PLACEMENT_3D ( 'NONE', #2496, #8280, #6401 ) ;
#1808=CARTESIAN_POINT ( 'NONE',  ( -33.16810284049710589, -83.21632480446695013, -4.330127018922185655 ) ) ;
#1809=DIRECTION ( 'NONE',  ( -0.1566598588826321192, 0.9876526153536342445, 7.798540720466731404E-17 ) ) ;
#1810=ORIENTED_EDGE ( 'NONE', *, *, #14128, .F. ) ;
#1811=AXIS2_PLACEMENT_3D ( 'NONE', #12247, #17905, #18082 ) ;
#1813=ORIENTED_EDGE ( 'NONE', *, *, #12144, .T. ) ;
#1814=LINE ( 'NONE', #7603, #7719 ) ;
#1815=AXIS2_PLACEMENT_3D ( 'NONE', #10512, #26, #15927 ) ;
#1816=DIRECTION ( 'NONE',  ( -0.1566598588826321192, 0.9876526153536342445, 7.798540720466730171E-17 ) ) ;
#1817=EDGE_LOOP ( 'NONE', ( #2784, #14936 ) ) ;
#1819=CIRCLE ( 'NONE', #12400, 1.500000000000000888 ) ;
#1820=VERTEX_POINT ( 'NONE', #17267 ) ;
#1821=DIRECTION ( 'NONE',  ( 0.000000000000000000, 0.000000000000000000, 1.000000000000000000 ) ) ;
#1822=AXIS2_PLACEMENT_3D ( 'NONE', #6529, #8834, #10757 ) ;
#1823=FACE_BOUND ( 'NONE', #3030, .T. ) ;
#1824=AXIS2_PLACEMENT_3D ( 'NONE', #6485, #16513, #17879 ) ;
#1825=VERTEX_POINT ( 'NONE', #11527 ) ;
#1826=EDGE_CURVE ( 'NONE', #11513, #15461, #965, .T. ) ;
#1829=VERTEX_POINT ( 'NONE', #2904 ) ;
#1830=EDGE_CURVE ( 'NONE', #6534, #3287, #14280, .T. ) ;
#1831=AXIS2_PLACEMENT_3D ( 'NONE', #13760, #10655, #16642 ) ;
#1832=DIRECTION ( 'NONE',  ( -0.1566598588826321192, 0.9876526153536342445, 7.798540720466731404E-17 ) ) ;
#1833=ORIENTED_EDGE ( 'NONE', *, *, #7332, .T. ) ;
#1834=DIRECTION ( 'NONE',  ( 0.000000000000000000, 0.000000000000000000, 1.000000000000000000 ) ) ;
#1835=AXIS2_PLACEMENT_3D ( 'NONE', #9916, #7459, #4331 ) ;
#1837=DIRECTION ( 'NONE',  ( -0.9876526153536336894, -0.1566598588826349503, 0.000000000000000000 ) ) ;
#1838=DIRECTION ( 'NONE',  ( -0.1566598588826321192, 0.9876526153536342445, 7.798540720466730171E-17 ) ) ;
#1839=VERTEX_POINT ( 'NONE', #14204 ) ;
#1840=ORIENTED_EDGE ( 'NONE', *, *, #10688, .T. ) ;
#1841=CARTESIAN_POINT ( 'NONE',  ( -13.45468554360235203, -22.38394619046619383, 1.869203119972154228E-14 ) ) ;
#1842=AXIS2_PLACEMENT_3D ( 'NONE', #13120, #18687, #8872 ) ;
#1843=LINE ( 'NONE', #7633, #14151 ) ;
#1844=VECTOR ( 'NONE', #14175, 1000.000000000000000 ) ;
#1845=ORIENTED_EDGE ( 'NONE', *, *, #13785, .F. ) ;
#1847=AXIS2_PLACEMENT_3D ( 'NONE', #9884, #1378, #5635 ) ;
#1848=LINE ( 'NONE', #7639, #2697 ) ;
#1849=VECTOR ( 'NONE', #16760, 1000.000000000000000 ) ;
#1850=EDGE_CURVE ( 'NONE', #5249, #13731, #8819, .T. ) ;
#1851=CARTESIAN_POINT ( 'NONE',  ( -48.97054468615519340, -85.72288254658904805, -17.32050807568878525 ) ) ;
#1853=CARTESIAN_POINT ( 'NONE',  ( -51.47931123471710890, -28.41535075744750571, 1.887572821959364500E-14 ) ) ;
#1854=ADVANCED_FACE ( 'NONE', ( #7211 ), #14942, .F. ) ;
#1856=DIRECTION ( 'NONE',  ( 0.000000000000000000, 0.000000000000000000, 1.000000000000000000 ) ) ;
#1858=AXIS2_PLACEMENT_3D ( 'NONE', #2831, #12863, #17157 ) ;
#1859=AXIS2_PLACEMENT_3D ( 'NONE', #13139, #3097, #17645 ) ;
#1861=ORIENTED_EDGE ( 'NONE', *, *, #10638, .T. ) ;
#1862=ORIENTED_EDGE ( 'NONE', *, *, #4493, .T. ) ;
#1864=VERTEX_POINT ( 'NONE', #16382 ) ;
#1865=CIRCLE ( 'NONE', #17945, 1.500000000000001332 ) ;
#1866=ORIENTED_EDGE ( 'NONE', *, *, #2081, .T. ) ;
#1867=AXIS2_PLACEMENT_3D ( 'NONE', #13080, #18549, #14231 ) ;
#1868=ADVANCED_BREP_SHAPE_REPRESENTATION ( '', ( #2591, #18772 ), #7243 ) ;
#1869=CARTESIAN_POINT ( 'NONE',  ( -43.04462899403339549, -84.78292339329327376, 12.99038105676661203 ) ) ;
#1870=AXIS2_PLACEMENT_3D ( 'NONE', #8436, #15346, #2468 ) ;
#1871=EDGE_CURVE ( 'NONE', #2581, #18009, #5498, .T. ) ;
#1872=LINE ( 'NONE', #13414, #7030 ) ;
#1874=DIRECTION ( 'NONE',  ( -0.1566598588826321192, 0.9876526153536342445, 7.798540720466730171E-17 ) ) ;
#1878=AXIS2_PLACEMENT_3D ( 'NONE', #12178, #13333, #10751 ) ;
#1879=CARTESIAN_POINT ( 'NONE',  ( -0.9046745307415022808, -15.33077501878252136, -8.660254037844383745 ) ) ;
#1880=EDGE_LOOP ( 'NONE', ( #10584, #12657 ) ) ;
#1881=LINE ( 'NONE', #3373, #15321 ) ;
#1885=EDGE_LOOP ( 'NONE', ( #13407, #2564 ) ) ;
#1886=AXIS2_PLACEMENT_3D ( 'NONE', #4481, #1832, #319 ) ;
#1887=DIRECTION ( 'NONE',  ( -0.9876526153536336894, -0.1566598588826349503, 0.000000000000000000 ) ) ;
#1888=ORIENTED_EDGE ( 'NONE', *, *, #5404, .F. ) ;
#1889=ORIENTED_EDGE ( 'NONE', *, *, #5855, .T. ) ;
#1890=ORIENTED_EDGE ( 'NONE', *, *, #17831, .T. ) ;
#1891=CARTESIAN_POINT ( 'NONE',  ( -62.13913668266654611, -25.04368626950570587, 17.32050807568881723 ) ) ;
#1892=AXIS2_PLACEMENT_3D ( 'NONE', #2101, #16612, #9020 ) ;
#1893=AXIS2_PLACEMENT_3D ( 'NONE', #1190, #7154, #2949 ) ;
#1895=ORIENTED_EDGE ( 'NONE', *, *, #5420, .F. ) ;
#1896=DIRECTION ( 'NONE',  ( -0.1566598588826321192, 0.9876526153536342445, 7.798540720466730171E-17 ) ) ;
#1897=DIRECTION ( 'NONE',  ( -0.9876526153536336894, -0.1566598588826349503, 0.000000000000000000 ) ) ;
#1898=CARTESIAN_POINT ( 'NONE',  ( -39.13365354279672914, -26.45710252141460828, 4.330127018922217630 ) ) ;
#1901=CYLINDRICAL_SURFACE ( 'NONE', #12698, 1.500000000000001554 ) ;
#1902=CARTESIAN_POINT ( 'NONE',  ( -53.74408945216072198, -23.71207746900331870, -17.32050807568878170 ) ) ;
#1903=VERTEX_POINT ( 'NONE', #8794 ) ;
#1904=EDGE_CURVE ( 'NONE', #13791, #16138, #6237, .T. ) ;
#1905=EDGE_CURVE ( 'NONE', #1188, #9148, #9739, .T. ) ;
#1907=CIRCLE ( 'NONE', #5556, 1.499999999999999556 ) ;
#1908=CYLINDRICAL_SURFACE ( 'NONE', #9225, 1.500000000000001554 ) ;
#1909=DIRECTION ( 'NONE',  ( -0.1566598588826321747, 0.9876526153536343555, 0.000000000000000000 ) ) ;
#1910=ADVANCED_FACE ( 'NONE', ( #6051 ), #16187, .F. ) ;
#1911=ORIENTED_EDGE ( 'NONE', *, *, #24, .F. ) ;
#1912=ORIENTED_EDGE ( 'NONE', *, *, #2458, .F. ) ;
#1913=EDGE_LOOP ( 'NONE', ( #17983, #10408, #13405, #10472 ) ) ;
#1914=EDGE_LOOP ( 'NONE', ( #17770, #12813, #13909, #3661 ) ) ;
#1915=EDGE_LOOP ( 'NONE', ( #4337, #8057 ) ) ;
#1918=FACE_BOUND ( 'NONE', #15833, .T. ) ;
#1919=ORIENTED_EDGE ( 'NONE', *, *, #6145, .T. ) ;
#1920=AXIS2_PLACEMENT_3D ( 'NONE', #6240, #11702, #15031 ) ;
#1921=ORIENTED_EDGE ( 'NONE', *, *, #9782, .T. ) ;
#1922=ORIENTED_EDGE ( 'NONE', *, *, #526, .T. ) ;
#1924=CYLINDRICAL_SURFACE ( 'NONE', #7581, 1.500000000000001554 ) ;
#1926=CARTESIAN_POINT ( 'NONE',  ( -16.70711637639958269, -17.83733276090463704, -12.99038105676658006 ) ) ;
#1928=CARTESIAN_POINT ( 'NONE',  ( -38.14600092744309734, -26.30044266253198160, -8.660254037844380193 ) ) ;
#1929=ORIENTED_EDGE ( 'NONE', *, *, #17709, .T. ) ;
#1931=AXIS2_PLACEMENT_3D ( 'NONE', #12368, #2330, #1224 ) ;
#1932=CARTESIAN_POINT ( 'NONE',  ( 3.231158466157545206, -19.73726462726228092, 30.00000000000000000 ) ) ;
#1935=FACE_OUTER_BOUND ( 'NONE', #11244, .T. ) ;
#1937=ORIENTED_EDGE ( 'NONE', *, *, #18207, .T. ) ;
#1938=VERTEX_POINT ( 'NONE', #13231 ) ;
#1940=EDGE_CURVE ( 'NONE', #10290, #15025, #1872, .T. ) ;
#1941=DIRECTION ( 'NONE',  ( -0.1566598588826321192, 0.9876526153536342445, 7.798540720466731404E-17 ) ) ;
#1945=ORIENTED_EDGE ( 'NONE', *, *, #13940, .T. ) ;
#1946=DIRECTION ( 'NONE',  ( -0.1566598588826321747, 0.9876526153536343555, 0.000000000000000000 ) ) ;
#1948=DIRECTION ( 'NONE',  ( -0.1566598588826321747, 0.9876526153536343555, 0.000000000000000000 ) ) ;
#1949=ORIENTED_EDGE ( 'NONE', *, *, #11524, .F. ) ;
#1951=ORIENTED_EDGE ( 'NONE', *, *, #16965, .T. ) ;
#1952=ORIENTED_EDGE ( 'NONE', *, *, #8811, .F. ) ;
#1953=DIRECTION ( 'NONE',  ( -0.9876526153536336894, -0.1566598588826350336, 0.000000000000000000 ) ) ;
#1954=ADVANCED_FACE ( 'NONE', ( #11701 ), #4892, .F. ) ;
#1955=ORIENTED_EDGE ( 'NONE', *, *, #1830, .T. ) ;
#1956=EDGE_CURVE ( 'NONE', #15309, #12162, #10303, .T. ) ;
#1957=ORIENTED_EDGE ( 'NONE', *, *, #1394, .T. ) ;
#1958=EDGE_CURVE ( 'NONE', #7789, #2452, #7620, .T. ) ;
#1959=CARTESIAN_POINT ( 'NONE',  ( -34.97868976044173195, -20.73554015023333008, 4.330127018922218518 ) ) ;
#1960=DIRECTION ( 'NONE',  ( -0.1566598588826321192, 0.9876526153536342445, 7.798540720466730171E-17 ) ) ;
#1963=CARTESIAN_POINT ( 'NONE',  ( -36.62488699423481364, -83.76463431055616127, -4.330127018922185655 ) ) ;
#1966=CARTESIAN_POINT ( 'NONE',  ( -41.60278508118079799, -26.84875216862118918, 1.887572821959364500E-14 ) ) ;
#1967=ORIENTED_EDGE ( 'NONE', *, *, #14405, .T. ) ;
#1968=DIRECTION ( 'NONE',  ( -0.1566598588826321747, 0.9876526153536343555, 0.000000000000000000 ) ) ;
#1969=CIRCLE ( 'NONE', #5310, 1.500000000000000888 ) ;
#1970=EDGE_CURVE ( 'NONE', #12438, #15242, #8533, .T. ) ;
#1971=CARTESIAN_POINT ( 'NONE',  ( -38.14600092744310444, -26.30044266253198160, 8.660254037844417496 ) ) ;
#1973=ADVANCED_FACE ( 'NONE', ( #10477 ), #4521, .F. ) ;
#1974=DIRECTION ( 'NONE',  ( -0.9876526153536341335, -0.1566598588826327021, 0.000000000000000000 ) ) ;
#1977=EDGE_LOOP ( 'NONE', ( #11451, #14276, #11198, #4345 ) ) ;
#1979=CARTESIAN_POINT ( 'NONE',  ( -10.98555400521827607, -21.99229654325962002, 12.99038105676661381 ) ) ;
#1981=CARTESIAN_POINT ( 'NONE',  ( -41.60278508118080509, -26.84875216862118918, -17.32050807568878170 ) ) ;
#1982=CIRCLE ( 'NONE', #9551, 1.499999999999999556 ) ;
#1983=ORIENTED_EDGE ( 'NONE', *, *, #2995, .F. ) ;
#1984=CARTESIAN_POINT ( 'NONE',  ( -0.5755665338273054932, -78.04654946134009208, 4.330127018922209636 ) ) ;
#1985=CARTESIAN_POINT ( 'NONE',  ( 0.000000000000000000, 0.000000000000000000, 30.00000000000000000 ) ) ;
#1986=LINE ( 'NONE', #7772, #2958 ) ;
#1987=CARTESIAN_POINT ( 'NONE',  ( -31.52190560670403841, -20.18723064414411184, -4.330127018922180326 ) ) ;
#1988=DIRECTION ( 'NONE',  ( -1.000000000000000000, 0.000000000000000000, 0.000000000000000000 ) ) ;
#1989=CARTESIAN_POINT ( 'NONE',  ( -31.52190560670403841, -20.18723064414412249, 21.65063509461102242 ) ) ;
#1990=ORIENTED_EDGE ( 'NONE', *, *, #3378, .T. ) ;
#1991=FACE_BOUND ( 'NONE', #11735, .T. ) ;
#1992=DIRECTION ( 'NONE',  ( -0.1566598588826321192, 0.9876526153536342445, 7.798540720466731404E-17 ) ) ;
#1993=VERTEX_POINT ( 'NONE', #6984 ) ;
#1997=AXIS2_PLACEMENT_3D ( 'NONE', #18168, #1159, #13817 ) ;
#1998=ORIENTED_EDGE ( 'NONE', *, *, #9376, .F. ) ;
#1999=ORIENTED_EDGE ( 'NONE', *, *, #10412, .F. ) ;
#2000=ORIENTED_EDGE ( 'NONE', *, *, #11230, .T. ) ;
#2001=CARTESIAN_POINT ( 'NONE',  ( -9.504075082187823043, -21.75730675493566579, 4.330127018922214077 ) ) ;
#2002=ORIENTED_EDGE ( 'NONE', *, *, #6879, .F. ) ;
#2003=EDGE_LOOP ( 'NONE', ( #14656, #16427, #4356, #15741 ) ) ;
#2004=FACE_BOUND ( 'NONE', #13705, .T. ) ;
#2007=CIRCLE ( 'NONE', #6566, 1.499999999999999556 ) ;
#2008=CARTESIAN_POINT ( 'NONE',  ( -16.87183468716221313, -80.63143713290352821, -4.330127018922185655 ) ) ;
#2009=ORIENTED_EDGE ( 'NONE', *, *, #15330, .T. ) ;
#2010=AXIS2_PLACEMENT_3D ( 'NONE', #6527, #5288, #18111 ) ;
#2013=FACE_BOUND ( 'NONE', #15725, .T. ) ;
#2015=DIRECTION ( 'NONE',  ( -0.1566598588826321192, 0.9876526153536342445, 7.798540720466731404E-17 ) ) ;
#2016=CARTESIAN_POINT ( 'NONE',  ( -62.83731631128386397, -30.21693913459777647, 8.660254037844417496 ) ) ;
#2017=AXIS2_PLACEMENT_3D ( 'NONE', #13064, #17448, #8977 ) ;
#2018=DIRECTION ( 'NONE',  ( -0.1566598588826321192, 0.9876526153536342445, 7.798540720466730171E-17 ) ) ;
#2019=ORIENTED_EDGE ( 'NONE', *, *, #12167, .T. ) ;
#2021=DIRECTION ( 'NONE',  ( -0.9876526153536336894, -0.1566598588826349503, 0.000000000000000000 ) ) ;
#2022=AXIS2_PLACEMENT_3D ( 'NONE', #7051, #8552, #2658 ) ;
#2023=DIRECTION ( 'NONE',  ( 0.000000000000000000, 0.000000000000000000, 1.000000000000000000 ) ) ;
#2024=ORIENTED_EDGE ( 'NONE', *, *, #7887, .T. ) ;
#2025=VECTOR ( 'NONE', #9331, 1000.000000000000000 ) ;
#2026=ORIENTED_EDGE ( 'NONE', *, *, #1905, .T. ) ;
#2028=AXIS2_PLACEMENT_3D ( 'NONE', #3381, #4808, #10494 ) ;
#2029=ORIENTED_EDGE ( 'NONE', *, *, #18331, .F. ) ;
#2030=FACE_BOUND ( 'NONE', #11289, .T. ) ;
#2031=VECTOR ( 'NONE', #8879, 1000.000000000000000 ) ;
#2032=CYLINDRICAL_SURFACE ( 'NONE', #16388, 1.500000000000001554 ) ;
#2033=EDGE_CURVE ( 'NONE', #12526, #10470, #3073, .T. ) ;
#2034=CARTESIAN_POINT ( 'NONE',  ( -58.84707083969148300, -87.28948113541535747, -17.32050807568878525 ) ) ;
#2036=CARTESIAN_POINT ( 'NONE',  ( -64.31879523431432233, -30.45192892292171294, -8.660254037844380193 ) ) ;
#2037=EDGE_CURVE ( 'NONE', #11894, #9998, #61, .T. ) ;
#2039=DIRECTION ( 'NONE',  ( -0.1566598588826321747, 0.9876526153536343555, 0.000000000000000000 ) ) ;
#2040=ORIENTED_EDGE ( 'NONE', *, *, #6876, .T. ) ;
#2041=CARTESIAN_POINT ( 'NONE',  ( -77.65210554158829837, -32.56683701783724416, 1.869203119972154228E-14 ) ) ;
#2042=EDGE_LOOP ( 'NONE', ( #8774, #10055 ) ) ;
#2043=CIRCLE ( 'NONE', #16268, 1.500000000000001332 ) ;
#2044=EDGE_LOOP ( 'NONE', ( #1599, #13275, #10107, #15945 ) ) ;
#2045=LINE ( 'NONE', #4963, #7869 ) ;
#2047=FACE_OUTER_BOUND ( 'NONE', #12379, .T. ) ;
#2048=DIRECTION ( 'NONE',  ( -0.1566598588826321192, 0.9876526153536342445, 7.798540720466730171E-17 ) ) ;
#2049=VECTOR ( 'NONE', #15616, 1000.000000000000000 ) ;
#2050=EDGE_LOOP ( 'NONE', ( #13470, #17687 ) ) ;
#2051=DIRECTION ( 'NONE',  ( -0.1566598588826321192, 0.9876526153536342445, 7.798540720466730171E-17 ) ) ;
#2052=EDGE_CURVE ( 'NONE', #16948, #9536, #17331, .T. ) ;
#2053=DIRECTION ( 'NONE',  ( -0.1566598588826321192, 0.9876526153536342445, 7.798540720466731404E-17 ) ) ;
#2055=DIRECTION ( 'NONE',  ( -0.1566598588826321192, 0.9876526153536342445, 7.798540720466730171E-17 ) ) ;
#2059=EDGE_CURVE ( 'NONE', #9632, #8678, #11526, .T. ) ;
#2060=CIRCLE ( 'NONE', #15075, 1.500000000000000888 ) ;
#2061=DIRECTION ( 'NONE',  ( -0.9876526153536336894, -0.1566598588826349503, 0.000000000000000000 ) ) ;
#2062=CIRCLE ( 'NONE', #2401, 1.500000000000001332 ) ;
#2063=VERTEX_POINT ( 'NONE', #17489 ) ;
#2064=DIRECTION ( 'NONE',  ( 0.000000000000000000, 0.000000000000000000, 1.000000000000000000 ) ) ;
#2066=ORIENTED_EDGE ( 'NONE', *, *, #16543, .T. ) ;
#2067=STYLED_ITEM ( 'NONE', ( #3832 ), #1868 ) ;
#2069=ORIENTED_EDGE ( 'NONE', *, *, #1068, .F. ) ;
#2070=ORIENTED_EDGE ( 'NONE', *, *, #4867, .F. ) ;
#2071=ORIENTED_EDGE ( 'NONE', *, *, #14640, .T. ) ;
#2072=AXIS2_PLACEMENT_3D ( 'NONE', #7267, #5646, #8672 ) ;
#2074=VECTOR ( 'NONE', #10680, 1000.000000000000000 ) ;
#2075=CARTESIAN_POINT ( 'NONE',  ( -14.40270314877813895, -80.23978748569695085, 17.32050807568881368 ) ) ;
#2076=CIRCLE ( 'NONE', #9935, 1.499999999999999556 ) ;
#2078=CARTESIAN_POINT ( 'NONE',  ( -31.68662391746666884, -82.98133501614299234, -12.99038105676658539 ) ) ;
#2080=EDGE_CURVE ( 'NONE', #777, #11543, #1468, .T. ) ;
#2081=EDGE_CURVE ( 'NONE', #4058, #3679, #7258, .T. ) ;
#2085=EDGE_LOOP ( 'NONE', ( #16322, #13061, #14561, #14604 ) ) ;
#2086=EDGE_CURVE ( 'NONE', #7797, #4310, #14869, .T. ) ;
#2087=DIRECTION ( 'NONE',  ( -0.1566598588826321192, 0.9876526153536342445, 7.798540720466731404E-17 ) ) ;
#2088=EDGE_CURVE ( 'NONE', #6604, #3989, #7634, .T. ) ;
#2089=CARTESIAN_POINT ( 'NONE',  ( -35.67686938905902849, -25.90879301532540779, -4.330127018922181215 ) ) ;
#2090=EDGE_CURVE ( 'NONE', #10127, #17419, #10160, .T. ) ;
#2091=AXIS2_PLACEMENT_3D ( 'NONE', #1131, #4026, #8406 ) ;
#2092=LINE ( 'NONE', #685, #10562 ) ;
#2093=AXIS2_PLACEMENT_3D ( 'NONE', #11506, #17515, #3080 ) ;
#2094=ORIENTED_EDGE ( 'NONE', *, *, #18316, .F. ) ;
#2095=ORIENTED_EDGE ( 'NONE', *, *, #717, .F. ) ;
#2096=VERTEX_POINT ( 'NONE', #10353 ) ;
#2098=CARTESIAN_POINT ( 'NONE',  ( 55.85952145814821534, 6.938893903907228378E-15, 92.77853496600735639 ) ) ;
#2099=FACE_BOUND ( 'NONE', #4289, .T. ) ;
#2100=CIRCLE ( 'NONE', #6650, 139.0000000000000000 ) ;
#2101=CARTESIAN_POINT ( 'NONE',  ( -2.057045456857760524, -78.28153924966404986, -4.330127018922185655 ) ) ;
#2102=EDGE_CURVE ( 'NONE', #11883, #10248, #9436, .T. ) ;
#2103=ADVANCED_FACE ( 'NONE', ( #18666 ), #5637, .F. ) ;
#2104=CIRCLE ( 'NONE', #7820, 1.500000000000000444 ) ;
#2106=DIRECTION ( 'NONE',  ( -0.1566598588826321192, 0.9876526153536342445, 7.798540720466731404E-17 ) ) ;
#2107=ORIENTED_EDGE ( 'NONE', *, *, #2994, .F. ) ;
#2109=CARTESIAN_POINT ( 'NONE',  ( -66.78792677269838407, -30.84357857012830095, 4.330127018922217630 ) ) ;
#2111=EDGE_CURVE ( 'NONE', #4310, #7797, #10637, .T. ) ;
#2112=AXIS2_PLACEMENT_3D ( 'NONE', #18330, #12284, #18124 ) ;
#2115=VERTEX_POINT ( 'NONE', #6107 ) ;
#2116=ORIENTED_EDGE ( 'NONE', *, *, #2404, .T. ) ;
#2117=DIRECTION ( 'NONE',  ( -0.1566598588826321192, 0.9876526153536342445, 7.798540720466731404E-17 ) ) ;
#2118=CIRCLE ( 'NONE', #10280, 1.499999999999999556 ) ;
#2119=CARTESIAN_POINT ( 'NONE',  ( -29.21749237908258223, -82.58968536893640078, 7.308518362537324739E-15 ) ) ;
#2120=EDGE_LOOP ( 'NONE', ( #14336, #10632, #9227, #2656 ) ) ;
#2125=CIRCLE ( 'NONE', #2745, 1.500000000000000444 ) ;
#2128=CARTESIAN_POINT ( 'NONE',  ( 0.000000000000000000, 0.000000000000000000, 30.00000000000000000 ) ) ;
#2129=CARTESIAN_POINT ( 'NONE',  ( -6.047290928450125946, -21.20899724884646531, 4.330127018922214077 ) ) ;
#2130=AXIS2_PLACEMENT_3D ( 'NONE', #8647, #5896, #4371 ) ;
#2131=DIRECTION ( 'NONE',  ( 0.000000000000000000, 0.000000000000000000, 1.000000000000000000 ) ) ;
#2134=EDGE_CURVE ( 'NONE', #5271, #6856, #10440, .T. ) ;
#2136=CIRCLE ( 'NONE', #42, 1.499999999999999556 ) ;
#2137=DIRECTION ( 'NONE',  ( -0.9876526153536344665, -0.1566598588826304539, 0.000000000000000000 ) ) ;
#2139=VERTEX_POINT ( 'NONE', #18057 ) ;
#2140=DIRECTION ( 'NONE',  ( -0.9876526153536344665, -0.1566598588826304539, 0.000000000000000000 ) ) ;
#2141=ORIENTED_EDGE ( 'NONE', *, *, #13823, .F. ) ;
#2142=EDGE_LOOP ( 'NONE', ( #16142, #208, #5298, #15919 ) ) ;
#2143=ORIENTED_EDGE ( 'NONE', *, *, #8442, .F. ) ;
#2145=EDGE_CURVE ( 'NONE', #1209, #3494, #5512, .T. ) ;
#2148=ORIENTED_EDGE ( 'NONE', *, *, #4321, .T. ) ;
#2149=EDGE_LOOP ( 'NONE', ( #13958, #11494, #17524, #16764 ) ) ;
#2150=FACE_OUTER_BOUND ( 'NONE', #2085, .T. ) ;
#2151=CARTESIAN_POINT ( 'NONE',  ( -23.29157668696081629, -81.64972621564064070, -4.330127018922185655 ) ) ;
#2152=VECTOR ( 'NONE', #18373, 1000.000000000000000 ) ;
#2155=DIRECTION ( 'NONE',  ( -0.1566598588826321192, 0.9876526153536342445, 7.798540720466730171E-17 ) ) ;
#2157=FILL_AREA_STYLE_COLOUR ( '', #6322 ) ;
#2159=CARTESIAN_POINT ( 'NONE',  ( -83.14047854185180597, 6.938893903907228378E-15, 92.77853496600735639 ) ) ;
#2160=FACE_OUTER_BOUND ( 'NONE', #13539, .T. ) ;
#2161=FACE_BOUND ( 'NONE', #7843, .T. ) ;
#2163=CIRCLE ( 'NONE', #7624, 1.500000000000000888 ) ;
#2164=DIRECTION ( 'NONE',  ( -0.1566598588826321192, 0.9876526153536342445, 7.798540720466730171E-17 ) ) ;
#2165=DIRECTION ( 'NONE',  ( -0.9876526153536336894, -0.1566598588826350336, 0.000000000000000000 ) ) ;
#2166=ORIENTED_EDGE ( 'NONE', *, *, #1186, .F. ) ;
#2168=EDGE_CURVE ( 'NONE', #9109, #8230, #8227, .T. ) ;
#2169=EDGE_LOOP ( 'NONE', ( #12654, #9944, #4667, #8189 ) ) ;
#2170=AXIS2_PLACEMENT_3D ( 'NONE', #6483, #12220, #9409 ) ;
#2173=ORIENTED_EDGE ( 'NONE', *, *, #6910, .F. ) ;
#2175=CARTESIAN_POINT ( 'NONE',  ( -30.04042668367358360, -19.95224085582017537, 12.99038105676661736 ) ) ;
#2177=DIRECTION ( 'NONE',  ( -0.1566598588826321747, 0.9876526153536343555, 0.000000000000000000 ) ) ;
#2178=DIRECTION ( 'NONE',  ( 0.000000000000000000, 0.000000000000000000, 1.000000000000000000 ) ) ;
#2179=CARTESIAN_POINT ( 'NONE',  ( -22.34355908178503469, -23.79388492040988012, -4.330127018922181215 ) ) ;
#2180=CARTESIAN_POINT ( 'NONE',  ( -1.892327146095121204, -15.48743487766515337, 12.99038105676661026 ) ) ;
#2181=EDGE_LOOP ( 'NONE', ( #18565, #13788, #12286, #17679 ) ) ;
#2182=AXIS2_PLACEMENT_3D ( 'NONE', #13926, #14976, #5224 ) ;
#2183=LINE ( 'NONE', #7963, #14898 ) ;
#2184=DIRECTION ( 'NONE',  ( -0.1566598588826321747, 0.9876526153536343555, 0.000000000000000000 ) ) ;
#2185=CYLINDRICAL_SURFACE ( 'NONE', #8168, 1.500000000000000666 ) ;
#2186=CARTESIAN_POINT ( 'NONE',  ( -64.77298653181324539, -88.22944028871116018, -12.99038105676658539 ) ) ;
#2187=AXIS2_PLACEMENT_3D ( 'NONE', #368, #14852, #10583 ) ;
#2189=VERTEX_POINT ( 'NONE', #2199 ) ;
#2190=ORIENTED_EDGE ( 'NONE', *, *, #3347, .T. ) ;
#2191=CARTESIAN_POINT ( 'NONE',  ( -69.54653129781877396, -26.21863521112544149, 12.99038105676661736 ) ) ;
#2192=EDGE_CURVE ( 'NONE', #13410, #16508, #13653, .T. ) ;
#2193=EDGE_CURVE ( 'NONE', #11968, #1456, #15488, .T. ) ;
#2194=FACE_BOUND ( 'NONE', #10461, .T. ) ;
#2195=EDGE_CURVE ( 'NONE', #3989, #6604, #16099, .T. ) ;
#2198=ORIENTED_EDGE ( 'NONE', *, *, #8033, .F. ) ;
#2199=CARTESIAN_POINT ( 'NONE',  ( -0.9046745307415022808, -15.33077501878252136, 1.387778780781445518E-14 ) ) ;
#2200=FACE_BOUND ( 'NONE', #1915, .T. ) ;
#2203=DIRECTION ( 'NONE',  ( -0.9876526153536336894, -0.1566598588826349503, 0.000000000000000000 ) ) ;
#2204=FACE_OUTER_BOUND ( 'NONE', #5437, .T. ) ;
#2205=ORIENTED_EDGE ( 'NONE', *, *, #10209, .F. ) ;
#2206=ORIENTED_EDGE ( 'NONE', *, *, #18096, .T. ) ;
#2207=CARTESIAN_POINT ( 'NONE',  ( -29.25712738926042888, -24.89050393258829175, 4.330127018922217630 ) ) ;
#2210=DIRECTION ( 'NONE',  ( -0.9876526153536336894, -0.1566598588826349503, 0.000000000000000000 ) ) ;
#2211=ORIENTED_EDGE ( 'NONE', *, *, #18409, .T. ) ;
#2213=DIRECTION ( 'NONE',  ( -0.9876526153536336894, -0.1566598588826349503, 0.000000000000000000 ) ) ;
#2214=ADVANCED_FACE ( 'NONE', ( #13941 ), #16722, .F. ) ;
#2215=CIRCLE ( 'NONE', #14013, 1.500000000000000000 ) ;
#2217=DIRECTION ( 'NONE',  ( 0.000000000000000000, 0.000000000000000000, 1.000000000000000000 ) ) ;
#2218=VERTEX_POINT ( 'NONE', #7980 ) ;
#2219=FACE_BOUND ( 'NONE', #4988, .T. ) ;
#2220=CARTESIAN_POINT ( 'NONE',  ( -15.71946376104596155, -17.68067290202200326, 8.660254037844413944 ) ) ;
#2221=CARTESIAN_POINT ( 'NONE',  ( 2.841582609732560272, -19.79905851890276836, 17.32050807568881012 ) ) ;
#2224=VERTEX_POINT ( 'NONE', #786 ) ;
#2226=DIRECTION ( 'NONE',  ( -0.1566598588826321192, 0.9876526153536342445, 7.798540720466730171E-17 ) ) ;
#2229=CARTESIAN_POINT ( 'NONE',  ( -48.80582637539254875, -22.92877817459017109, 8.660254037844417496 ) ) ;
#2230=EDGE_LOOP ( 'NONE', ( #5491, #7299 ) ) ;
#2233=ORIENTED_EDGE ( 'NONE', *, *, #10295, .F. ) ;
#2234=ORIENTED_EDGE ( 'NONE', *, *, #14306, .T. ) ;
#2235=ORIENTED_EDGE ( 'NONE', *, *, #9131, .T. ) ;
#2236=CYLINDRICAL_SURFACE ( 'NONE', #2325, 1.500000000000001554 ) ;
#2237=CARTESIAN_POINT ( 'NONE',  ( -55.22556837519117323, -23.94706725732726582, -17.32050807568878170 ) ) ;
#2238=EDGE_CURVE ( 'NONE', #719, #5148, #6855, .T. ) ;
#2239=CARTESIAN_POINT ( 'NONE',  ( -54.89646037827696290, -86.66284169988483654, 4.330127018922213189 ) ) ;
#2240=EDGE_CURVE ( 'NONE', #6731, #15683, #12755, .T. ) ;
#2241=DIRECTION ( 'NONE',  ( 0.000000000000000000, 0.000000000000000000, 1.000000000000000000 ) ) ;
#2242=ORIENTED_EDGE ( 'NONE', *, *, #17053, .F. ) ;
#2243=CARTESIAN_POINT ( 'NONE',  ( -39.13365354279672914, -26.45710252141460828, 21.65063509461101887 ) ) ;
#2244=EDGE_CURVE ( 'NONE', #14517, #4155, #11239, .T. ) ;
#2245=CARTESIAN_POINT ( 'NONE',  ( -46.50141314777108903, -85.33123289938248490, 21.65063509461101532 ) ) ;
#2246=DIRECTION ( 'NONE',  ( -0.1566598588826321192, 0.9876526153536342445, 7.798540720466731404E-17 ) ) ;
#2249=EDGE_LOOP ( 'NONE', ( #4015, #2353 ) ) ;
#2250=FACE_OUTER_BOUND ( 'NONE', #9511, .T. ) ;
#2251=AXIS2_PLACEMENT_3D ( 'NONE', #18612, #15600, #12407 ) ;
#2252=ORIENTED_EDGE ( 'NONE', *, *, #4677, .F. ) ;
#2253=ORIENTED_EDGE ( 'NONE', *, *, #4651, .T. ) ;
#2254=CARTESIAN_POINT ( 'NONE',  ( -50.28730529842300001, -23.16376796291411821, 8.660254037844417496 ) ) ;
#2255=EDGE_LOOP ( 'NONE', ( #8646, #9606, #6691, #1107 ) ) ;
#2256=DIRECTION ( 'NONE',  ( -0.1566598588826321192, 0.9876526153536342445, 7.798540720466731404E-17 ) ) ;
#2257=CARTESIAN_POINT ( 'NONE',  ( -12.75650591498505371, -17.21069332537410901, -17.32050807568878170 ) ) ;
#2259=CARTESIAN_POINT ( 'NONE',  ( -31.68662391746665463, -82.98133501614299234, -4.330127018922185655 ) ) ;
#2261=EDGE_CURVE ( 'NONE', #18705, #11379, #4589, .T. ) ;
#2262=CARTESIAN_POINT ( 'NONE',  ( 1.360103686702108128, -20.03404830722672259, 1.348786077179111942E-14 ) ) ;
#2265=DIRECTION ( 'NONE',  ( -0.1566598588826321192, 0.9876526153536342445, 7.798540720466730171E-17 ) ) ;
#2266=EDGE_LOOP ( 'NONE', ( #6257, #16011 ) ) ;
#2267=FACE_BOUND ( 'NONE', #167, .T. ) ;
#2269=DIRECTION ( 'NONE',  ( 0.000000000000000000, 0.000000000000000000, 1.000000000000000000 ) ) ;
#2270=DIRECTION ( 'NONE',  ( -0.9876526153536341335, -0.1566598588826327021, 0.000000000000000000 ) ) ;
#2271=EDGE_CURVE ( 'NONE', #17176, #14148, #5818, .T. ) ;
#2272=FACE_OUTER_BOUND ( 'NONE', #18170, .T. ) ;
#2274=ORIENTED_EDGE ( 'NONE', *, *, #11748, .T. ) ;
#2275=EDGE_LOOP ( 'NONE', ( #3398, #12045, #9731, #10897 ) ) ;
#2277=VECTOR ( 'NONE', #6489, 1000.000000000000000 ) ;
#2278=FACE_BOUND ( 'NONE', #7998, .T. ) ;
#2279=VERTEX_POINT ( 'NONE', #12517 ) ;
#2280=CARTESIAN_POINT ( 'NONE',  ( -6.995308533625909320, -79.06483854407721878, 12.99038105676660848 ) ) ;
#2281=CIRCLE ( 'NONE', #3780, 1.500000000000000000 ) ;
#2282=EDGE_CURVE ( 'NONE', #14381, #16999, #10900, .T. ) ;
#2283=DIRECTION ( 'NONE',  ( -0.1566598588826321192, 0.9876526153536342445, 7.798540720466730171E-17 ) ) ;
#2284=FACE_BOUND ( 'NONE', #18682, .T. ) ;
#2286=VERTEX_POINT ( 'NONE', #9703 ) ;
#2288=LINE ( 'NONE', #4935, #4220 ) ;
#2289=EDGE_CURVE ( 'NONE', #7636, #3282, #2491, .T. ) ;
#2291=ORIENTED_EDGE ( 'NONE', *, *, #15337, .T. ) ;
#2292=EDGE_LOOP ( 'NONE', ( #4470, #14480 ) ) ;
#2293=CYLINDRICAL_SURFACE ( 'NONE', #8428, 1.500000000000001554 ) ;
#2296=ORIENTED_EDGE ( 'NONE', *, *, #15182, .F. ) ;
#2297=ORIENTED_EDGE ( 'NONE', *, *, #9033, .F. ) ;
#2298=FACE_OUTER_BOUND ( 'NONE', #4277, .T. ) ;
#2299=AXIS2_PLACEMENT_3D ( 'NONE', #6386, #8924, #10627 ) ;
#2300=VERTEX_POINT ( 'NONE', #3980 ) ;
#2302=AXIS2_PLACEMENT_3D ( 'NONE', #16083, #8408, #15979 ) ;
#2303=CYLINDRICAL_SURFACE ( 'NONE', #1831, 1.500000000000001554 ) ;
#2304=CARTESIAN_POINT ( 'NONE',  ( -51.27495791377663181, -23.32042782179674489, -4.330127018922180326 ) ) ;
#2307=EDGE_CURVE ( 'NONE', #4718, #4101, #9786, .T. ) ;
#2308=ADVANCED_FACE ( 'NONE', ( #4070 ), #13740, .F. ) ;
#2309=ADVANCED_FACE ( 'NONE', ( #7040 ), #11261, .F. ) ;
#2310=AXIS2_PLACEMENT_3D ( 'NONE', #3116, #8905, #17744 ) ;
#2312=CARTESIAN_POINT ( 'NONE',  ( -42.38608437559395981, -21.91048909185306215, -8.660254037844380193 ) ) ;
#2313=ADVANCED_FACE ( 'NONE', ( #12784 ), #18629, .F. ) ;
#2317=FACE_BOUND ( 'NONE', #14050, .T. ) ;
#2318=CARTESIAN_POINT ( 'NONE',  ( -67.73594437787414790, -88.69941986535906153, -4.330127018922185655 ) ) ;
#2319=VERTEX_POINT ( 'NONE', #15724 ) ;
#2320=CARTESIAN_POINT ( 'NONE',  ( -9.464440072009985272, -79.45648819128378193, -8.660254037844385522 ) ) ;
#2321=ORIENTED_EDGE ( 'NONE', *, *, #3926, .T. ) ;
#2322=ORIENTED_EDGE ( 'NONE', *, *, #16408, .T. ) ;
#2323=CARTESIAN_POINT ( 'NONE',  ( -10.45209268736360997, -79.61314805016640150, -21.65063509461098690 ) ) ;
#2325=AXIS2_PLACEMENT_3D ( 'NONE', #18306, #16771, #8116 ) ;
#2326=CARTESIAN_POINT ( 'NONE',  ( -3.373806069125583562, -15.72242466598909871, -21.65063509461098334 ) ) ;
#2327=DIRECTION ( 'NONE',  ( -0.9876526153536336894, -0.1566598588826349503, 0.000000000000000000 ) ) ;
#2328=VERTEX_POINT ( 'NONE', #9674 ) ;
#2330=DIRECTION ( 'NONE',  ( -0.1566598588826321747, 0.9876526153536343555, 0.000000000000000000 ) ) ;
#2331=CIRCLE ( 'NONE', #3829, 1.499999999999999556 ) ;
#2333=DIRECTION ( 'NONE',  ( -0.1566598588826321192, 0.9876526153536342445, 7.798540720466730171E-17 ) ) ;
#2334=ADVANCED_FACE ( 'NONE', ( #18343 ), #2747, .F. ) ;
#2335=EDGE_CURVE ( 'NONE', #6102, #10673, #6118, .T. ) ;
#2337=CARTESIAN_POINT ( 'NONE',  ( -67.57122606711153878, -25.90531549336017392, 12.99038105676661736 ) ) ;
#2338=CIRCLE ( 'NONE', #13524, 1.500000000000001332 ) ;
#2339=DIRECTION ( 'NONE',  ( -0.9876526153536336894, -0.1566598588826350336, 0.000000000000000000 ) ) ;
#2340=ORIENTED_EDGE ( 'NONE', *, *, #14918, .T. ) ;
#2341=EDGE_CURVE ( 'NONE', #18706, #11180, #17027, .T. ) ;
#2342=FACE_OUTER_BOUND ( 'NONE', #4630, .T. ) ;
#2343=ORIENTED_EDGE ( 'NONE', *, *, #7518, .F. ) ;
#2344=CYLINDRICAL_SURFACE ( 'NONE', #15747, 1.500000000000001554 ) ;
#2345=EDGE_LOOP ( 'NONE', ( #17280, #16458, #17068, #1845 ) ) ;
#2346=AXIS2_PLACEMENT_3D ( 'NONE', #7532, #6313, #9144 ) ;
#2348=CARTESIAN_POINT ( 'NONE',  ( -62.83731631128386397, -30.21693913459777647, 1.869203119972154228E-14 ) ) ;
#2349=ORIENTED_EDGE ( 'NONE', *, *, #15969, .F. ) ;
#2350=CARTESIAN_POINT ( 'NONE',  ( -1.069392841504132052, -78.12487939078141608, -8.660254037844385522 ) ) ;
#2352=CYLINDRICAL_SURFACE ( 'NONE', #6764, 2.000000000000000000 ) ;
#2353=ORIENTED_EDGE ( 'NONE', *, *, #2088, .F. ) ;
#2354=DIRECTION ( 'NONE',  ( 0.000000000000000000, 0.000000000000000000, 1.000000000000000000 ) ) ;
#2355=CARTESIAN_POINT ( 'NONE',  ( 5.350349158294472218, -77.10659030804430358, 1.077796531449093893E-14 ) ) ;
#2356=AXIS2_PLACEMENT_3D ( 'NONE', #17243, #10657, #16172 ) ;
#2357=CARTESIAN_POINT ( 'NONE',  ( 0.3724510713484854851, -20.19070816610934926, -12.99038105676658361 ) ) ;
#2358=DIRECTION ( 'NONE',  ( -0.1566598588826321192, 0.9876526153536342445, 7.798540720466730171E-17 ) ) ;
#2360=VECTOR ( 'NONE', #90, 1000.000000000000000 ) ;
#2361=DIRECTION ( 'NONE',  ( -0.9876526153536341335, -0.1566598588826327021, 0.000000000000000000 ) ) ;
#2362=EDGE_CURVE ( 'NONE', #7723, #795, #18279, .T. ) ;
#2363=CARTESIAN_POINT ( 'NONE',  ( 5.350349158294472218, -77.10659030804430358, -17.32050807568878525 ) ) ;
#2364=EDGE_CURVE ( 'NONE', #14520, #17136, #12030, .T. ) ;
#2366=ORIENTED_EDGE ( 'NONE', *, *, #10826, .F. ) ;
#2367=ORIENTED_EDGE ( 'NONE', *, *, #7350, .F. ) ;
#2368=ORIENTED_EDGE ( 'NONE', *, *, #980, .F. ) ;
#2369=ORIENTED_EDGE ( 'NONE', *, *, #18134, .T. ) ;
#2370=CARTESIAN_POINT ( 'NONE',  ( -11.93357161039406300, -79.84813783849037350, 4.330127018922213189 ) ) ;
#2373=CIRCLE ( 'NONE', #18770, 1.500000000000001332 ) ;
#2374=FACE_BOUND ( 'NONE', #11193, .T. ) ;
#2375=CIRCLE ( 'NONE', #16922, 1.500000000000000888 ) ;
#2376=LINE ( 'NONE', #3779, #12779 ) ;
#2377=CIRCLE ( 'NONE', #5418, 2.000000000000000000 ) ;
#2379=CARTESIAN_POINT ( 'NONE',  ( -8.476787456656362352, -79.29982833240116236, 4.330127018922213189 ) ) ;
#2380=AXIS2_PLACEMENT_3D ( 'NONE', #7309, #11620, #1688 ) ;
#2383=CIRCLE ( 'NONE', #12356, 1.500000000000000888 ) ;
#2384=ORIENTED_EDGE ( 'NONE', *, *, #7202, .T. ) ;
#2385=CARTESIAN_POINT ( 'NONE',  ( -75.96627329761737712, -27.23692429386253977, 4.330127018922218518 ) ) ;
#2386=DIRECTION ( 'NONE',  ( -0.1566598588826321192, 0.9876526153536342445, 7.798540720466731404E-17 ) ) ;
#2387=DIRECTION ( 'NONE',  ( 0.000000000000000000, 0.000000000000000000, 1.000000000000000000 ) ) ;
#2388=CARTESIAN_POINT ( 'NONE',  ( -58.88670584986932965, -29.59029969906724844, 4.330127018922217630 ) ) ;
#2391=CIRCLE ( 'NONE', #11755, 1.500000000000000444 ) ;
#2392=ORIENTED_EDGE ( 'NONE', *, *, #9208, .F. ) ;
#2393=CYLINDRICAL_SURFACE ( 'NONE', #5847, 1.500000000000001554 ) ;
#2394=ADVANCED_FACE ( 'NONE', ( #4758 ), #17779, .F. ) ;
#2395=CIRCLE ( 'NONE', #15711, 1.500000000000000888 ) ;
#2396=ORIENTED_EDGE ( 'NONE', *, *, #18794, .T. ) ;
#2398=CYLINDRICAL_SURFACE ( 'NONE', #10023, 1.500000000000001554 ) ;
#2399=DIRECTION ( 'NONE',  ( -0.1566598588826321747, 0.9876526153536343555, 0.000000000000000000 ) ) ;
#2400=CIRCLE ( 'NONE', #6347, 1.500000000000000000 ) ;
#2401=AXIS2_PLACEMENT_3D ( 'NONE', #4129, #2728, #15985 ) ;
#2402=AXIS2_PLACEMENT_3D ( 'NONE', #4373, #10060, #7065 ) ;
#2403=FACE_BOUND ( 'NONE', #10267, .T. ) ;
#2404=EDGE_CURVE ( 'NONE', #10467, #6767, #3682, .T. ) ;
#2406=EDGE_CURVE ( 'NONE', #11338, #2916, #10344, .T. ) ;
#2407=DIRECTION ( 'NONE',  ( 0.000000000000000000, 0.000000000000000000, 1.000000000000000000 ) ) ;
#2411=CIRCLE ( 'NONE', #12385, 1.499999999999999556 ) ;
#2413=AXIS2_PLACEMENT_3D ( 'NONE', #10642, #17598, #6205 ) ;
#2414=CARTESIAN_POINT ( 'NONE',  ( -41.56315007100297265, -84.54793360496931598, -12.99038105676658539 ) ) ;
#2416=CARTESIAN_POINT ( 'NONE',  ( -51.97313754239392836, -28.49368068688882971, 4.330127018922217630 ) ) ;
#2417=CARTESIAN_POINT ( 'NONE',  ( -1.892327146095121204, -15.48743487766515337, 4.330127018922213189 ) ) ;
#2418=VECTOR ( 'NONE', #15957, 1000.000000000000000 ) ;
#2419=ORIENTED_EDGE ( 'NONE', *, *, #3895, .T. ) ;
#2420=VERTEX_POINT ( 'NONE', #15930 ) ;
#2423=VERTEX_POINT ( 'NONE', #9108 ) ;
#2424=ORIENTED_EDGE ( 'NONE', *, *, #16634, .T. ) ;
#2425=FACE_OUTER_BOUND ( 'NONE', #6337, .T. ) ;
#2426=CYLINDRICAL_SURFACE ( 'NONE', #13314, 1.500000000000000666 ) ;
#2427=ORIENTED_EDGE ( 'NONE', *, *, #11947, .T. ) ;
#2428=DIRECTION ( 'NONE',  ( -0.1566598588826321747, 0.9876526153536343555, 0.000000000000000000 ) ) ;
#2429=CARTESIAN_POINT ( 'NONE',  ( -62.83731631128386397, -30.21693913459777647, -17.32050807568878170 ) ) ;
#2430=VECTOR ( 'NONE', #835, 1000.000000000000000 ) ;
#2432=EDGE_CURVE ( 'NONE', #3894, #8207, #1712, .T. ) ;
#2433=VECTOR ( 'NONE', #2164, 1000.000000000000000 ) ;
#2434=DIRECTION ( 'NONE',  ( -0.1566598588826321747, 0.9876526153536343555, 0.000000000000000000 ) ) ;
#2435=CYLINDRICAL_SURFACE ( 'NONE', #18191, 1.500000000000000666 ) ;
#2436=EDGE_CURVE ( 'NONE', #15692, #14720, #2938, .T. ) ;
#2437=ORIENTED_EDGE ( 'NONE', *, *, #16111, .T. ) ;
#2438=VECTOR ( 'NONE', #12223, 1000.000000000000000 ) ;
#2439=FACE_OUTER_BOUND ( 'NONE', #4415, .T. ) ;
#2440=CARTESIAN_POINT ( 'NONE',  ( -2.000000000000000000, 0.000000000000000000, 30.00000000000000000 ) ) ;
#2442=VECTOR ( 'NONE', #5275, 1000.000000000000000 ) ;
#2443=FACE_OUTER_BOUND ( 'NONE', #18447, .T. ) ;
#2444=DIRECTION ( 'NONE',  ( -0.1566598588826321747, 0.9876526153536343555, 0.000000000000000000 ) ) ;
#2445=ORIENTED_EDGE ( 'NONE', *, *, #7202, .F. ) ;
#2447=EDGE_LOOP ( 'NONE', ( #5086, #2274, #17953, #17450 ) ) ;
#2450=AXIS2_PLACEMENT_3D ( 'NONE', #7655, #13488, #9165 ) ;
#2451=LINE ( 'NONE', #8237, #6914 ) ;
#2452=VERTEX_POINT ( 'NONE', #114 ) ;
#2454=DIRECTION ( 'NONE',  ( -0.9876526153536341335, -0.1566598588826327021, 0.000000000000000000 ) ) ;
#2455=VERTEX_POINT ( 'NONE', #3307 ) ;
#2456=CIRCLE ( 'NONE', #7317, 1.500000000000000888 ) ;
#2457=DIRECTION ( 'NONE',  ( -0.1566598588826321747, 0.9876526153536343555, 0.000000000000000000 ) ) ;
#2458=EDGE_CURVE ( 'NONE', #15004, #2601, #993, .T. ) ;
#2459=CARTESIAN_POINT ( 'NONE',  ( -24.31886431249228409, -24.10720463817513703, 21.65063509461101887 ) ) ;
#2460=ORIENTED_EDGE ( 'NONE', *, *, #9208, .T. ) ;
#2461=AXIS2_PLACEMENT_3D ( 'NONE', #7999, #14263, #12824 ) ;
#2463=DIRECTION ( 'NONE',  ( 0.000000000000000000, 0.000000000000000000, 1.000000000000000000 ) ) ;
#2464=CARTESIAN_POINT ( 'NONE',  ( -67.07739975943471222, -25.82698556391886058, 8.660254037844417496 ) ) ;
#2466=FACE_OUTER_BOUND ( 'NONE', #6512, .T. ) ;
#2467=DIRECTION ( 'NONE',  ( -0.1566598588826321192, 0.9876526153536342445, 7.798540720466730171E-17 ) ) ;
#2468=DIRECTION ( 'NONE',  ( -0.9876526153536336894, -0.1566598588826349503, 0.000000000000000000 ) ) ;
#2469=VERTEX_POINT ( 'NONE', #6089 ) ;
#2473=CARTESIAN_POINT ( 'NONE',  ( 3.231158466157545206, -19.73726462726228092, 25.00000000000000711 ) ) ;
#2474=AXIS2_PLACEMENT_3D ( 'NONE', #2902, #12776, #7301 ) ;
#2475=VECTOR ( 'NONE', #16615, 1000.000000000000000 ) ;
#2476=VERTEX_POINT ( 'NONE', #17572 ) ;
#2479=ORIENTED_EDGE ( 'NONE', *, *, #7099, .T. ) ;
#2482=AXIS2_PLACEMENT_3D ( 'NONE', #16984, #11258, #2640 ) ;
#2483=FACE_BOUND ( 'NONE', #9992, .T. ) ;
#2484=VECTOR ( 'NONE', #16297, 1000.000000000000000 ) ;
#2488=AXIS2_PLACEMENT_3D ( 'NONE', #10977, #1992, #13720 ) ;
#2490=CARTESIAN_POINT ( 'NONE',  ( -71.02801022084922522, -26.45362499944938151, 4.330127018922218518 ) ) ;
#2491=LINE ( 'NONE', #3699, #13363 ) ;
#2493=LINE ( 'NONE', #6858, #4409 ) ;
#2495=FACE_OUTER_BOUND ( 'NONE', #10053, .T. ) ;
#2496=CARTESIAN_POINT ( 'NONE',  ( -20.86208015875457988, -23.55889513208593655, -12.99038105676658006 ) ) ;
#2497=CARTESIAN_POINT ( 'NONE',  ( -62.63296299034337977, -25.12201619894701565, 12.99038105676661736 ) ) ;
#2498=DIRECTION ( 'NONE',  ( -0.1566598588826321747, 0.9876526153536343555, 0.000000000000000000 ) ) ;
#2499=FACE_OUTER_BOUND ( 'NONE', #7986, .T. ) ;
#2500=CARTESIAN_POINT ( 'NONE',  ( 10.28861223506262412, -76.32329101363113466, 9.043241838514131834E-15 ) ) ;
#2501=ORIENTED_EDGE ( 'NONE', *, *, #2145, .T. ) ;
#2503=LINE ( 'NONE', #9603, #6718 ) ;
#2504=ORIENTED_EDGE ( 'NONE', *, *, #16437, .T. ) ;
#2505=FACE_OUTER_BOUND ( 'NONE', #7205, .T. ) ;
#2506=EDGE_LOOP ( 'NONE', ( #4361, #9243 ) ) ;
#2507=CIRCLE ( 'NONE', #8266, 1.499999999999999556 ) ;
#2509=DIRECTION ( 'NONE',  ( -0.9876526153536336894, -0.1566598588826349503, 0.000000000000000000 ) ) ;
#2510=EDGE_CURVE ( 'NONE', #1139, #18416, #8247, .T. ) ;
#2511=DIRECTION ( 'NONE',  ( -0.9876526153536336894, -0.1566598588826349503, 0.000000000000000000 ) ) ;
#2513=DIRECTION ( 'NONE',  ( -0.9876526153536344665, -0.1566598588826304539, 0.000000000000000000 ) ) ;
#2516=ORIENTED_EDGE ( 'NONE', *, *, #15678, .F. ) ;
#2517=CIRCLE ( 'NONE', #18298, 1.500000000000000888 ) ;
#2518=FACE_BOUND ( 'NONE', #2760, .T. ) ;
#2519=DIRECTION ( 'NONE',  ( -0.1566598588826321192, 0.9876526153536342445, 7.798540720466731404E-17 ) ) ;
#2520=ORIENTED_EDGE ( 'NONE', *, *, #12264, .F. ) ;
#2521=EDGE_CURVE ( 'NONE', #11293, #12109, #8557, .T. ) ;
#2522=EDGE_LOOP ( 'NONE', ( #6844, #9418, #6094, #18318 ) ) ;
#2523=EDGE_LOOP ( 'NONE', ( #13795, #17664 ) ) ;
#2524=LINE ( 'NONE', #1123, #10007 ) ;
#2525=CARTESIAN_POINT ( 'NONE',  ( 5.350349158294472218, -77.10659030804430358, -17.32050807568878525 ) ) ;
#2526=DIRECTION ( 'NONE',  ( -0.1566598588826321192, 0.9876526153536342445, 7.798540720466731404E-17 ) ) ;
#2527=DIRECTION ( 'NONE',  ( 0.000000000000000000, 0.000000000000000000, 1.000000000000000000 ) ) ;
#2528=VECTOR ( 'NONE', #7212, 1000.000000000000000 ) ;
#2529=DIRECTION ( 'NONE',  ( -0.9876526153536341335, -0.1566598588826327021, 0.000000000000000000 ) ) ;
#2532=EDGE_CURVE ( 'NONE', #15648, #13882, #3979, .T. ) ;
#2534=EDGE_LOOP ( 'NONE', ( #16425, #7412 ) ) ;
#2535=DIRECTION ( 'NONE',  ( -0.1566598588826321192, 0.9876526153536342445, 7.798540720466731404E-17 ) ) ;
#2538=ORIENTED_EDGE ( 'NONE', *, *, #5486, .T. ) ;
#2539=CARTESIAN_POINT ( 'NONE',  ( -77.44775222064782838, -27.47191408218647979, -12.99038105676658006 ) ) ;
#2540=EDGE_CURVE ( 'NONE', #3070, #17772, #13819, .T. ) ;
#2541=DIRECTION ( 'NONE',  ( -0.9876526153536341335, -0.1566598588826327021, 0.000000000000000000 ) ) ;
#2542=ORIENTED_EDGE ( 'NONE', *, *, #7949, .T. ) ;
#2543=ADVANCED_FACE ( 'NONE', ( #10779 ), #15168, .F. ) ;
#2545=VERTEX_POINT ( 'NONE', #17850 ) ;
#2547=ORIENTED_EDGE ( 'NONE', *, *, #7098, .F. ) ;
#2548=DIRECTION ( 'NONE',  ( 0.000000000000000000, 0.000000000000000000, 1.000000000000000000 ) ) ;
#2550=CYLINDRICAL_SURFACE ( 'NONE', #10032, 1.500000000000001554 ) ;
#2551=DIRECTION ( 'NONE',  ( -0.1566598588826321192, 0.9876526153536342445, 7.798540720466731404E-17 ) ) ;
#2552=EDGE_CURVE ( 'NONE', #10229, #10439, #2183, .T. ) ;
#2553=DIRECTION ( 'NONE',  ( -0.9876526153536341335, -0.1566598588826327021, 0.000000000000000000 ) ) ;
#2555=EDGE_CURVE ( 'NONE', #7813, #5152, #10948, .T. ) ;
#2556=EDGE_CURVE ( 'NONE', #139, #7759, #11252, .T. ) ;
#2558=CARTESIAN_POINT ( 'NONE',  ( -43.08426400421124924, -27.08374195694514341, 17.32050807568881723 ) ) ;
#2559=EDGE_CURVE ( 'NONE', #7022, #13460, #2801, .T. ) ;
#2560=VERTEX_POINT ( 'NONE', #5001 ) ;
#2562=CARTESIAN_POINT ( 'NONE',  ( -88.82622559915370175, -29.27674910825304622, -24.99999999999999645 ) ) ;
#2563=ORIENTED_EDGE ( 'NONE', *, *, #9742, .T. ) ;
#2564=ORIENTED_EDGE ( 'NONE', *, *, #7249, .F. ) ;
#2565=CARTESIAN_POINT ( 'NONE',  ( -52.96079015774756726, -28.65034054577146705, -17.32050807568878170 ) ) ;
#2566=FACE_BOUND ( 'NONE', #17922, .T. ) ;
#2567=CARTESIAN_POINT ( 'NONE',  ( -10.45209268736360997, -79.61314805016641571, 12.99038105676661203 ) ) ;
#2568=CIRCLE ( 'NONE', #13150, 1.500000000000000888 ) ;
#2569=ORIENTED_EDGE ( 'NONE', *, *, #11692, .F. ) ;
#2570=CARTESIAN_POINT ( 'NONE',  ( -30.04042668367358360, -19.95224085582017182, 4.330127018922218518 ) ) ;
#2571=CARTESIAN_POINT ( 'NONE',  ( -45.51376053241748565, -85.17457304049985112, 8.660254037844412167 ) ) ;
#2573=ORIENTED_EDGE ( 'NONE', *, *, #17229, .T. ) ;
#2576=DIRECTION ( 'NONE',  ( 0.000000000000000000, 0.000000000000000000, 1.000000000000000000 ) ) ;
#2579=CARTESIAN_POINT ( 'NONE',  ( -14.44233815895597672, -22.54060604934882051, 21.65063509461101177 ) ) ;
#2580=DIRECTION ( 'NONE',  ( -0.1566598588826321747, 0.9876526153536343555, 0.000000000000000000 ) ) ;
#2581=VERTEX_POINT ( 'NONE', #18140 ) ;
#2582=EDGE_CURVE ( 'NONE', #7610, #13224, #5110, .T. ) ;
#2583=VERTEX_POINT ( 'NONE', #3768 ) ;
#2584=ORIENTED_EDGE ( 'NONE', *, *, #5946, .F. ) ;
#2585=CARTESIAN_POINT ( 'NONE',  ( -70.20507591625822386, -89.09106951256565310, 8.660254037844412167 ) ) ;
#2587=EDGE_LOOP ( 'NONE', ( #16141, #7529, #1388, #12352 ) ) ;
#2588=DIRECTION ( 'NONE',  ( -0.1566598588826321192, 0.9876526153536342445, 7.798540720466730171E-17 ) ) ;
#2589=CARTESIAN_POINT ( 'NONE',  ( -67.57122606711153878, -25.90531549336016326, -12.99038105676658006 ) ) ;
#2590=PRODUCT ( 'Heavy-Duty Perforated Sieve Plate', 'Heavy-Duty Perforated Sieve Plate', '', ( #6883 ) ) ;
#2591=MANIFOLD_SOLID_BREP ( 'Boss-Extrude3', #16010 ) ;
#2592=CARTESIAN_POINT ( 'NONE',  ( -77.44775222064782838, -27.47191408218648689, 4.330127018922218518 ) ) ;
#2598=DIRECTION ( 'NONE',  ( -0.9876526153536344665, -0.1566598588826304539, 0.000000000000000000 ) ) ;
#2599=DIRECTION ( 'NONE',  ( -0.1566598588826321747, 0.9876526153536343555, 0.000000000000000000 ) ) ;
#2600=DIRECTION ( 'NONE',  ( -0.1566598588826321192, 0.9876526153536342445, 7.798540720466731404E-17 ) ) ;
#2601=VERTEX_POINT ( 'NONE', #6748 ) ;
#2602=ORIENTED_EDGE ( 'NONE', *, *, #7468, .T. ) ;
#2603=DIRECTION ( 'NONE',  ( -0.1566598588826321747, 0.9876526153536343555, 0.000000000000000000 ) ) ;
#2604=LINE ( 'NONE', #4012, #7607 ) ;
#2605=AXIS2_PLACEMENT_3D ( 'NONE', #10255, #13184, #5234 ) ;
#2607=EDGE_CURVE ( 'NONE', #6427, #15608, #6736, .T. ) ;
#2609=ORIENTED_EDGE ( 'NONE', *, *, #9681, .F. ) ;
#2611=EDGE_CURVE ( 'NONE', #5881, #15709, #11554, .T. ) ;
#2612=DIRECTION ( 'NONE',  ( -0.1566598588826321192, 0.9876526153536342445, 7.798540720466730171E-17 ) ) ;
#2613=CARTESIAN_POINT ( 'NONE',  ( -59.67000514428248437, -24.65203662229911785, -4.330127018922180326 ) ) ;
#2614=EDGE_LOOP ( 'NONE', ( #11880, #14288 ) ) ;
#2615=CARTESIAN_POINT ( 'NONE',  ( -44.03228160938702018, -84.93958325217590755, 17.32050807568881368 ) ) ;
#2617=DIRECTION ( 'NONE',  ( -0.000000000000000000, -0.000000000000000000, -1.000000000000000000 ) ) ;
#2618=DIRECTION ( 'NONE',  ( -0.1566598588826321747, 0.9876526153536343555, 0.000000000000000000 ) ) ;
#2619=CARTESIAN_POINT ( 'NONE',  ( -3.578159390066044665, -20.81734760163988440, -8.660254037844383745 ) ) ;
#2620=AXIS2_PLACEMENT_3D ( 'NONE', #7373, #18779, #13126 ) ;
#2621=DIRECTION ( 'NONE',  ( -0.9876526153536336894, -0.1566598588826349503, 0.000000000000000000 ) ) ;
#2623=LINE ( 'NONE', #15323, #15956 ) ;
#2625=DIRECTION ( 'NONE',  ( -0.1566598588826326743, -0.9876526153536341335, 0.000000000000000000 ) ) ;
#2627=ORIENTED_EDGE ( 'NONE', *, *, #7093, .F. ) ;
#2628=CIRCLE ( 'NONE', #9279, 1.500000000000001332 ) ;
#2629=VECTOR ( 'NONE', #6174, 1000.000000000000000 ) ;
#2630=DIRECTION ( 'NONE',  ( -0.1566598588826321747, 0.9876526153536343555, 0.000000000000000000 ) ) ;
#2631=EDGE_LOOP ( 'NONE', ( #14433, #10981 ) ) ;
#2632=ORIENTED_EDGE ( 'NONE', *, *, #5302, .F. ) ;
#2633=EDGE_CURVE ( 'NONE', #7092, #13293, #3379, .T. ) ;
#2634=CIRCLE ( 'NONE', #14437, 1.500000000000001332 ) ;
#2635=LINE ( 'NONE', #18792, #6423 ) ;
#2636=CIRCLE ( 'NONE', #6587, 1.500000000000000000 ) ;
#2639=ORIENTED_EDGE ( 'NONE', *, *, #6124, .F. ) ;
#2640=DIRECTION ( 'NONE',  ( 0.000000000000000000, 0.000000000000000000, 1.000000000000000000 ) ) ;
#2641=FACE_OUTER_BOUND ( 'NONE', #10045, .T. ) ;
#2642=ADVANCED_FACE ( 'NONE', ( #3965 ), #4259, .F. ) ;
#2643=VECTOR ( 'NONE', #8593, 1000.000000000000000 ) ;
#2644=DIRECTION ( 'NONE',  ( -0.1566598588826321192, 0.9876526153536342445, 7.798540720466731404E-17 ) ) ;
#2645=CYLINDRICAL_SURFACE ( 'NONE', #6979, 1.500000000000000888 ) ;
#2646=DIRECTION ( 'NONE',  ( -0.1566598588826321747, 0.9876526153536343555, 0.000000000000000000 ) ) ;
#2648=CARTESIAN_POINT ( 'NONE',  ( -31.68662391746665463, -82.98133501614300656, 4.330127018922213189 ) ) ;
#2649=CARTESIAN_POINT ( 'NONE',  ( -71.02801022084922522, -26.45362499944937795, -4.330127018922180326 ) ) ;
#2651=ORIENTED_EDGE ( 'NONE', *, *, #3022, .F. ) ;
#2652=CIRCLE ( 'NONE', #14753, 1.500000000000000888 ) ;
#2653=ORIENTED_EDGE ( 'NONE', *, *, #14593, .T. ) ;
#2655=DIRECTION ( 'NONE',  ( -0.9876526153536336894, -0.1566598588826349503, 0.000000000000000000 ) ) ;
#2656=ORIENTED_EDGE ( 'NONE', *, *, #11281, .F. ) ;
#2657=ORIENTED_EDGE ( 'NONE', *, *, #10702, .T. ) ;
#2658=DIRECTION ( 'NONE',  ( 0.000000000000000000, 0.000000000000000000, 1.000000000000000000 ) ) ;
#2659=FACE_BOUND ( 'NONE', #9383, .T. ) ;
#2661=ADVANCED_FACE ( 'NONE', ( #1072 ), #15540, .F. ) ;
#2662=CARTESIAN_POINT ( 'NONE',  ( -44.07191661956488105, -27.24040181582776299, -12.99038105676658006 ) ) ;
#2663=ORIENTED_EDGE ( 'NONE', *, *, #18603, .F. ) ;
#2665=ADVANCED_FACE ( 'NONE', ( #4151 ), #9855, .F. ) ;
#2666=DIRECTION ( 'NONE',  ( -0.1566598588826321192, 0.9876526153536342445, 7.798540720466730171E-17 ) ) ;
#2668=ORIENTED_EDGE ( 'NONE', *, *, #15638, .T. ) ;
#2669=AXIS2_PLACEMENT_3D ( 'NONE', #7851, #14950, #12083 ) ;
#2670=CARTESIAN_POINT ( 'NONE',  ( -40.41077914488671041, -21.59716937408779458, -8.660254037844380193 ) ) ;
#2672=AXIS2_PLACEMENT_3D ( 'NONE', #15675, #5922, #2702 ) ;
#2673=CARTESIAN_POINT ( 'NONE',  ( -55.42992169613162190, -29.04199019297804085, 12.99038105676661736 ) ) ;
#2675=AXIS2_PLACEMENT_3D ( 'NONE', #1611, #5594, #13142 ) ;
#2676=ORIENTED_EDGE ( 'NONE', *, *, #16258, .F. ) ;
#2677=EDGE_LOOP ( 'NONE', ( #5363, #7131 ) ) ;
#2678=DIRECTION ( 'NONE',  ( -0.1566598588826321747, 0.9876526153536343555, 0.000000000000000000 ) ) ;
#2679=ORIENTED_EDGE ( 'NONE', *, *, #1905, .F. ) ;
#2680=EDGE_LOOP ( 'NONE', ( #18041, #3184, #7910, #2999 ) ) ;
#2681=VERTEX_POINT ( 'NONE', #14111 ) ;
#2682=CARTESIAN_POINT ( 'NONE',  ( 2.000000000000000000, 2.449293598294706414E-16, 24.99999999999999289 ) ) ;
#2683=AXIS2_PLACEMENT_3D ( 'NONE', #14973, #16306, #14611 ) ;
#2684=CYLINDRICAL_SURFACE ( 'NONE', #16025, 144.0000000000000284 ) ;
#2685=ADVANCED_FACE ( 'NONE', ( #12676 ), #5407, .F. ) ;
#2686=VECTOR ( 'NONE', #8972, 1000.000000000000000 ) ;
#2690=CARTESIAN_POINT ( 'NONE',  ( -24.81269062016911064, -24.18553456761645393, -8.660254037844380193 ) ) ;
#2692=VERTEX_POINT ( 'NONE', #8439 ) ;
#2693=DIRECTION ( 'NONE',  ( -0.1566598588826321192, 0.9876526153536342445, 7.798540720466731404E-17 ) ) ;
#2694=DIRECTION ( 'NONE',  ( -0.9876526153536344665, -0.1566598588826304539, 0.000000000000000000 ) ) ;
#2695=VERTEX_POINT ( 'NONE', #10123 ) ;
#2696=DIRECTION ( 'NONE',  ( -0.1566598588826321747, 0.9876526153536343555, 0.000000000000000000 ) ) ;
#2697=VECTOR ( 'NONE', #11946, 1000.000000000000000 ) ;
#2698=CARTESIAN_POINT ( 'NONE',  ( -34.19539046602857724, -25.67380322700145356, -4.330127018922181215 ) ) ;
#2699=VERTEX_POINT ( 'NONE', #1784 ) ;
#2701=CARTESIAN_POINT ( 'NONE',  ( -43.86756329862441817, -22.14547888017700572, -8.660254037844380193 ) ) ;
#2702=DIRECTION ( 'NONE',  ( -0.9876526153536336894, -0.1566598588826349503, 0.000000000000000000 ) ) ;
#2703=CIRCLE ( 'NONE', #13278, 1.500000000000000888 ) ;
#2704=LINE ( 'NONE', #16071, #12408 ) ;
#2705=VECTOR ( 'NONE', #15391, 1000.000000000000000 ) ;
#2706=VECTOR ( 'NONE', #9460, 1000.000000000000000 ) ;
#2708=EDGE_LOOP ( 'NONE', ( #1911, #14500, #1537, #1738 ) ) ;
#2709=LINE ( 'NONE', #6716, #12422 ) ;
#2710=CARTESIAN_POINT ( 'NONE',  ( -16.70711637639958269, -17.83733276090463704, -4.330127018922180326 ) ) ;
#2711=VECTOR ( 'NONE', #4016, 1000.000000000000000 ) ;
#2712=AXIS2_PLACEMENT_3D ( 'NONE', #18399, #18501, #9904 ) ;
#2714=FACE_OUTER_BOUND ( 'NONE', #8482, .T. ) ;
#2715=CYLINDRICAL_SURFACE ( 'NONE', #5709, 2.500000000000002220 ) ;
#2716=EDGE_CURVE ( 'NONE', #1265, #2879, #5705, .T. ) ;
#2717=ORIENTED_EDGE ( 'NONE', *, *, #13276, .T. ) ;
#2718=AXIS2_PLACEMENT_3D ( 'NONE', #435, #345, #9052 ) ;
#2719=ADVANCED_FACE ( 'NONE', ( #10488 ), #5959, .F. ) ;
#2721=CIRCLE ( 'NONE', #13301, 1.500000000000000000 ) ;
#2722=CARTESIAN_POINT ( 'NONE',  ( -59.38053215754615621, -29.66862962850855112, 17.32050807568881723 ) ) ;
#2724=CARTESIAN_POINT ( 'NONE',  ( -42.87991068327077926, -21.98881902129437904, 4.330127018922218518 ) ) ;
#2725=ORIENTED_EDGE ( 'NONE', *, *, #4906, .F. ) ;
#2727=EDGE_CURVE ( 'NONE', #4996, #6863, #17526, .T. ) ;
#2728=DIRECTION ( 'NONE',  ( -0.1566598588826321192, 0.9876526153536342445, 7.798540720466731404E-17 ) ) ;
#2729=ORIENTED_EDGE ( 'NONE', *, *, #9852, .T. ) ;
#2730=AXIS2_PLACEMENT_3D ( 'NONE', #1963, #2055, #2509 ) ;
#2732=VERTEX_POINT ( 'NONE', #7313 ) ;
#2733=CARTESIAN_POINT ( 'NONE',  ( -66.25446545484369665, -88.46443007703511796, 12.99038105676661203 ) ) ;
#2734=DIRECTION ( 'NONE',  ( -0.9876526153536341335, -0.1566598588826327021, 0.000000000000000000 ) ) ;
#2735=CIRCLE ( 'NONE', #3320, 1.500000000000001332 ) ;
#2736=ORIENTED_EDGE ( 'NONE', *, *, #11008, .F. ) ;
#2737=ORIENTED_EDGE ( 'NONE', *, *, #4285, .T. ) ;
#2738=AXIS2_PLACEMENT_3D ( 'NONE', #17596, #4579, #8487 ) ;
#2739=CIRCLE ( 'NONE', #329, 1.500000000000000888 ) ;
#2743=CARTESIAN_POINT ( 'NONE',  ( -63.62061560569701157, -25.27867605782964588, 8.660254037844417496 ) ) ;
#2745=AXIS2_PLACEMENT_3D ( 'NONE', #9541, #3454, #13780 ) ;
#2746=CARTESIAN_POINT ( 'NONE',  ( -57.89905323451569785, -29.43363984018461466, 8.660254037844417496 ) ) ;
#2747=CYLINDRICAL_SURFACE ( 'NONE', #1579, 1.500000000000001554 ) ;
#2748=VECTOR ( 'NONE', #8691, 1000.000000000000000 ) ;
#2749=DIRECTION ( 'NONE',  ( -0.9876526153536336894, -0.1566598588826349503, 0.000000000000000000 ) ) ;
#2750=DIRECTION ( 'NONE',  ( -0.1566598588826321747, 0.9876526153536343555, 0.000000000000000000 ) ) ;
#2751=CARTESIAN_POINT ( 'NONE',  ( -52.75643683680708307, -23.55541761012069557, 4.330127018922218518 ) ) ;
#2752=EDGE_CURVE ( 'NONE', #4620, #17453, #3853, .T. ) ;
#2753=CARTESIAN_POINT ( 'NONE',  ( -1.892327146095121204, -15.48743487766515337, -4.330127018922183879 ) ) ;
#2754=CIRCLE ( 'NONE', #16365, 1.500000000000000888 ) ;
#2756=VERTEX_POINT ( 'NONE', #265 ) ;
#2757=AXIS2_PLACEMENT_3D ( 'NONE', #17132, #8113, #18209 ) ;
#2758=ORIENTED_EDGE ( 'NONE', *, *, #9726, .T. ) ;
#2759=DIRECTION ( 'NONE',  ( -0.1566598588826321192, 0.9876526153536342445, 7.798540720466730171E-17 ) ) ;
#2760=EDGE_LOOP ( 'NONE', ( #6345, #14303 ) ) ;
#2761=EDGE_CURVE ( 'NONE', #16216, #4058, #15070, .T. ) ;
#2762=ORIENTED_EDGE ( 'NONE', *, *, #3409, .T. ) ;
#2765=CARTESIAN_POINT ( 'NONE',  ( -59.67000514428248437, -24.65203662229911075, -21.65063509461098334 ) ) ;
#2766=EDGE_CURVE ( 'NONE', #14892, #18229, #250, .T. ) ;
#2767=AXIS2_PLACEMENT_3D ( 'NONE', #16850, #12543, #14067 ) ;
#2768=FACE_BOUND ( 'NONE', #962, .T. ) ;
#2769=CIRCLE ( 'NONE', #4275, 1.500000000000000888 ) ;
#2771=CYLINDRICAL_SURFACE ( 'NONE', #4192, 1.500000000000001554 ) ;
#2772=FACE_BOUND ( 'NONE', #16689, .T. ) ;
#2773=VECTOR ( 'NONE', #4247, 1000.000000000000000 ) ;
#2774=AXIS2_PLACEMENT_3D ( 'NONE', #5353, #15659, #4301 ) ;
#2776=DIRECTION ( 'NONE',  ( -0.9876526153536336894, -0.1566598588826349503, 0.000000000000000000 ) ) ;
#2777=CARTESIAN_POINT ( 'NONE',  ( 55.85952145814821534, 6.938893903907228378E-15, 30.00000000000000000 ) ) ;
#2781=EDGE_LOOP ( 'NONE', ( #13137, #4159, #18241, #13078 ) ) ;
#2782=EDGE_CURVE ( 'NONE', #16444, #8059, #4710, .T. ) ;
#2783=CIRCLE ( 'NONE', #8239, 1.500000000000001332 ) ;
#2784=ORIENTED_EDGE ( 'NONE', *, *, #14509, .T. ) ;
#2785=ORIENTED_EDGE ( 'NONE', *, *, #543, .T. ) ;
#2786=CARTESIAN_POINT ( 'NONE',  ( 1.893565004556770903, -77.65489981413351472, 8.660254037844408614 ) ) ;
#2788=ORIENTED_EDGE ( 'NONE', *, *, #9097, .T. ) ;
#2789=FACE_BOUND ( 'NONE', #10321, .T. ) ;
#2790=VECTOR ( 'NONE', #18267, 1000.000000000000000 ) ;
#2791=CYLINDRICAL_SURFACE ( 'NONE', #15414, 1.500000000000001554 ) ;
#2792=ORIENTED_EDGE ( 'NONE', *, *, #3504, .F. ) ;
#2793=FACE_OUTER_BOUND ( 'NONE', #14555, .T. ) ;
#2794=CYLINDRICAL_SURFACE ( 'NONE', #1847, 1.500000000000001554 ) ;
#2795=AXIS2_PLACEMENT_3D ( 'NONE', #13893, #2618, #8317 ) ;
#2796=DIRECTION ( 'NONE',  ( -0.1566598588826321192, 0.9876526153536342445, 7.798540720466730171E-17 ) ) ;
#2798=CARTESIAN_POINT ( 'NONE',  ( -84.23462711737164454, 33.01666666666666572, 35.00000000000000000 ) ) ;
#2799=CARTESIAN_POINT ( 'NONE',  ( -19.34096622554629263, -81.02308678011009135, -17.32050807568878525 ) ) ;
#2800=ADVANCED_FACE ( 'NONE', ( #11893 ), #8713, .F. ) ;
#2801=CIRCLE ( 'NONE', #2488, 1.499999999999999556 ) ;
#2802=CARTESIAN_POINT ( 'NONE',  ( -33.20773785067495254, -25.51714336811882688, 1.869203119972154228E-14 ) ) ;
#2803=EDGE_CURVE ( 'NONE', #10018, #2423, #14766, .T. ) ;
#2804=EDGE_LOOP ( 'NONE', ( #13674, #17767 ) ) ;
#2805=ORIENTED_EDGE ( 'NONE', *, *, #727, .F. ) ;
#2806=LINE ( 'NONE', #12738, #16601 ) ;
#2807=DIRECTION ( 'NONE',  ( -0.1566598588826321192, 0.9876526153536342445, 7.798540720466731404E-17 ) ) ;
#2808=CARTESIAN_POINT ( 'NONE',  ( -11.97320662057189899, -22.14895640214223960, 17.32050807568881012 ) ) ;
#2809=CIRCLE ( 'NONE', #9775, 1.500000000000000444 ) ;
#2810=ORIENTED_EDGE ( 'NONE', *, *, #8805, .T. ) ;
#2811=CARTESIAN_POINT ( 'NONE',  ( -36.46016868347219742, -20.97052993855726655, -21.65063509461097979 ) ) ;
#2812=LINE ( 'NONE', #14077, #6084 ) ;
#2813=DIRECTION ( 'NONE',  ( -0.1566598588826321192, 0.9876526153536342445, 7.798540720466730171E-17 ) ) ;
#2814=DIRECTION ( 'NONE',  ( -0.1566598588826321747, 0.9876526153536343555, 0.000000000000000000 ) ) ;
#2815=ORIENTED_EDGE ( 'NONE', *, *, #6698, .T. ) ;
#2816=AXIS2_PLACEMENT_3D ( 'NONE', #2075, #13632, #18035 ) ;
#2817=DIRECTION ( 'NONE',  ( -0.1566598588826321747, 0.9876526153536343555, 0.000000000000000000 ) ) ;
#2818=DIRECTION ( 'NONE',  ( -0.1566598588826321192, 0.9876526153536342445, 7.798540720466730171E-17 ) ) ;
#2819=CARTESIAN_POINT ( 'NONE',  ( -20.65772683781411345, -18.46397219643516507, 17.32050807568881012 ) ) ;
#2820=DIRECTION ( 'NONE',  ( -0.1566598588826321192, 0.9876526153536342445, 7.798540720466730171E-17 ) ) ;
#2821=ORIENTED_EDGE ( 'NONE', *, *, #1702, .F. ) ;
#2822=DIRECTION ( 'NONE',  ( -0.9876526153536341335, -0.1566598588826327021, 0.000000000000000000 ) ) ;
#2823=CARTESIAN_POINT ( 'NONE',  ( -40.41077914488671041, -21.59716937408780169, 8.660254037844417496 ) ) ;
#2824=ORIENTED_EDGE ( 'NONE', *, *, #6269, .T. ) ;
#2825=ORIENTED_EDGE ( 'NONE', *, *, #123, .T. ) ;
#2826=CARTESIAN_POINT ( 'NONE',  ( -19.38060123572413218, -23.32390534376198232, 21.65063509461101177 ) ) ;
#2828=EDGE_CURVE ( 'NONE', #626, #8310, #9321, .T. ) ;
#2829=EDGE_CURVE ( 'NONE', #8415, #719, #4475, .T. ) ;
#2830=EDGE_LOOP ( 'NONE', ( #2296, #12859, #3885, #737 ) ) ;
#2831=CARTESIAN_POINT ( 'NONE',  ( -77.65210554158829837, -32.56683701783724416, -17.32050807568878170 ) ) ;
#2832=DIRECTION ( 'NONE',  ( -0.1566598588826321192, 0.9876526153536342445, 7.798540720466731404E-17 ) ) ;
#2833=DIRECTION ( 'NONE',  ( -0.1566598588826321192, 0.9876526153536342445, 7.798540720466730171E-17 ) ) ;
#2834=CARTESIAN_POINT ( 'NONE',  ( -43.08426400421124924, -27.08374195694514341, 8.660254037844417496 ) ) ;
#2835=DIRECTION ( 'NONE',  ( -0.1566598588826321192, 0.9876526153536342445, 7.798540720466730171E-17 ) ) ;
#2836=DIRECTION ( 'NONE',  ( -0.1566598588826321192, 0.9876526153536342445, 7.798540720466731404E-17 ) ) ;
#2837=LINE ( 'NONE', #10122, #18396 ) ;
#2838=CIRCLE ( 'NONE', #8602, 1.500000000000000444 ) ;
#2839=CARTESIAN_POINT ( 'NONE',  ( -35.14340807120434818, -83.52964452223221770, 21.65063509461101532 ) ) ;
#2840=ORIENTED_EDGE ( 'NONE', *, *, #12389, .T. ) ;
#2841=DIRECTION ( 'NONE',  ( -0.9876526153536341335, -0.1566598588826327021, 0.000000000000000000 ) ) ;
#2843=EDGE_LOOP ( 'NONE', ( #15234, #11312, #5562, #5738 ) ) ;
#2845=ORIENTED_EDGE ( 'NONE', *, *, #17537, .F. ) ;
#2846=CARTESIAN_POINT ( 'NONE',  ( -36.46016868347219742, -20.97052993855726655, -21.65063509461097979 ) ) ;
#2847=EDGE_CURVE ( 'NONE', #3794, #16655, #1431, .T. ) ;
#2848=DIRECTION ( 'NONE',  ( -0.1566598588826321192, 0.9876526153536342445, 7.798540720466730171E-17 ) ) ;
#2850=EDGE_CURVE ( 'NONE', #4660, #11687, #14171, .T. ) ;
#2852=DIRECTION ( 'NONE',  ( -0.9876526153536336894, -0.1566598588826350336, 0.000000000000000000 ) ) ;
#2854=FACE_BOUND ( 'NONE', #11269, .T. ) ;
#2855=DIRECTION ( 'NONE',  ( -0.9876526153536344665, -0.1566598588826304539, 0.000000000000000000 ) ) ;
#2856=ORIENTED_EDGE ( 'NONE', *, *, #12161, .T. ) ;
#2857=ORIENTED_EDGE ( 'NONE', *, *, #10238, .F. ) ;
#2858=ORIENTED_EDGE ( 'NONE', *, *, #18462, .F. ) ;
#2860=ORIENTED_EDGE ( 'NONE', *, *, #12840, .F. ) ;
#2862=FACE_OUTER_BOUND ( 'NONE', #16925, .T. ) ;
#2863=CARTESIAN_POINT ( 'NONE',  ( -62.13913668266656032, -25.04368626950570231, 8.660254037844417496 ) ) ;
#2866=CARTESIAN_POINT ( 'NONE',  ( 0.5768043922889515285, -15.09578523045857601, -17.32050807568878170 ) ) ;
#2867=ADVANCED_FACE ( 'NONE', ( #11536 ), #10216, .F. ) ;
#2869=VECTOR ( 'NONE', #13484, 1000.000000000000000 ) ;
#2873=VERTEX_POINT ( 'NONE', #13147 ) ;
#2874=ORIENTED_EDGE ( 'NONE', *, *, #14245, .F. ) ;
#2875=CYLINDRICAL_SURFACE ( 'NONE', #2672, 1.500000000000001554 ) ;
#2876=DIRECTION ( 'NONE',  ( -0.1566598588826321192, 0.9876526153536342445, 7.798540720466730171E-17 ) ) ;
#2877=CYLINDRICAL_SURFACE ( 'NONE', #2346, 1.500000000000001554 ) ;
#2878=CARTESIAN_POINT ( 'NONE',  ( -43.08426400421124924, -27.08374195694514341, 1.869203119972154228E-14 ) ) ;
#2879=VERTEX_POINT ( 'NONE', #179 ) ;
#2880=LINE ( 'NONE', #14556, #11796 ) ;
#2881=AXIS2_PLACEMENT_3D ( 'NONE', #15193, #7984, #1837 ) ;
#2885=CARTESIAN_POINT ( 'NONE',  ( -31.52190560670403841, -20.18723064414411894, 12.99038105676661736 ) ) ;
#2887=ADVANCED_FACE ( 'NONE', ( #9260 ), #18114, .F. ) ;
#2888=ADVANCED_FACE ( 'NONE', ( #16783 ), #13512, .F. ) ;
#2889=AXIS2_PLACEMENT_3D ( 'NONE', #15164, #7960, #4995 ) ;
#2891=CARTESIAN_POINT ( 'NONE',  ( -19.38060123572413218, -23.32390534376198232, 12.99038105676661736 ) ) ;
#2892=LINE ( 'NONE', #14566, #14076 ) ;
#2894=ORIENTED_EDGE ( 'NONE', *, *, #1675, .F. ) ;
#2896=CIRCLE ( 'NONE', #10158, 1.500000000000000888 ) ;
#2897=CARTESIAN_POINT ( 'NONE',  ( 10.28861223506262412, -76.32329101363113466, -8.660254037844389075 ) ) ;
#2898=VERTEX_POINT ( 'NONE', #659 ) ;
#2900=ORIENTED_EDGE ( 'NONE', *, *, #15510, .F. ) ;
#2901=CIRCLE ( 'NONE', #1127, 1.499999999999999556 ) ;
#2902=CARTESIAN_POINT ( 'NONE',  ( -57.89905323451571206, -29.43363984018462176, 1.869203119972154228E-14 ) ) ;
#2904=CARTESIAN_POINT ( 'NONE',  ( -32.50955822205765600, -20.34389050302675273, 8.660254037844417496 ) ) ;
#2905=CARTESIAN_POINT ( 'NONE',  ( -8.312069145893737243, -16.50572396040226053, 21.65063509461101177 ) ) ;
#2906=CIRCLE ( 'NONE', #12891, 1.500000000000001332 ) ;
#2907=DIRECTION ( 'NONE',  ( -0.1566598588826321192, 0.9876526153536342445, 7.798540720466730171E-17 ) ) ;
#2909=CARTESIAN_POINT ( 'NONE',  ( -46.54104815794894279, -27.63205146303435100, 8.660254037844417496 ) ) ;
#2910=ORIENTED_EDGE ( 'NONE', *, *, #11115, .F. ) ;
#2911=CARTESIAN_POINT ( 'NONE',  ( -25.59598991458226536, -19.24727149084832689, 8.660254037844417496 ) ) ;
#2912=EDGE_CURVE ( 'NONE', #6362, #13731, #9458, .T. ) ;
#2913=ADVANCED_FACE ( 'NONE', ( #7947 ), #12378, .F. ) ;
#2914=DIRECTION ( 'NONE',  ( -0.1566598588826321747, 0.9876526153536343555, 0.000000000000000000 ) ) ;
#2915=DIRECTION ( 'NONE',  ( -0.9876526153536341335, -0.1566598588826327021, 0.000000000000000000 ) ) ;
#2916=VERTEX_POINT ( 'NONE', #15142 ) ;
#2917=CIRCLE ( 'NONE', #13495, 1.499999999999999556 ) ;
#2918=ORIENTED_EDGE ( 'NONE', *, *, #9984, .T. ) ;
#2919=EDGE_LOOP ( 'NONE', ( #18566, #13331, #9738, #11569 ) ) ;
#2921=CYLINDRICAL_SURFACE ( 'NONE', #1791, 1.500000000000001554 ) ;
#2922=VECTOR ( 'NONE', #158, 1000.000000000000000 ) ;
#2925=EDGE_LOOP ( 'NONE', ( #10432, #14885 ) ) ;
#2926=DIRECTION ( 'NONE',  ( -0.1566598588826321192, 0.9876526153536342445, 7.798540720466731404E-17 ) ) ;
#2928=FACE_BOUND ( 'NONE', #13748, .T. ) ;
#2929=ORIENTED_EDGE ( 'NONE', *, *, #7920, .F. ) ;
#2930=AXIS2_PLACEMENT_3D ( 'NONE', #5057, #2039, #12251 ) ;
#2932=ORIENTED_EDGE ( 'NONE', *, *, #15041, .T. ) ;
#2934=CARTESIAN_POINT ( 'NONE',  ( -45.01993422474066620, -85.09624311105851291, -21.65063509461098690 ) ) ;
#2936=ADVANCED_FACE ( 'NONE', ( #6622 ), #6528, .F. ) ;
#2937=AXIS2_PLACEMENT_3D ( 'NONE', #1093, #6865, #3611 ) ;
#2938=LINE ( 'NONE', #8733, #13378 ) ;
#2939=ADVANCED_FACE ( 'NONE', ( #13702 ), #5198, .F. ) ;
#2940=DIRECTION ( 'NONE',  ( -0.9876526153536341335, -0.1566598588826327021, 0.000000000000000000 ) ) ;
#2942=LINE ( 'NONE', #11732, #10555 ) ;
#2944=FACE_OUTER_BOUND ( 'NONE', #18556, .T. ) ;
#2945=ADVANCED_FACE ( 'NONE', ( #9080 ), #3374, .F. ) ;
#2946=VERTEX_POINT ( 'NONE', #9181 ) ;
#2947=ORIENTED_EDGE ( 'NONE', *, *, #10175, .T. ) ;
#2948=ORIENTED_EDGE ( 'NONE', *, *, #10985, .F. ) ;
#2949=DIRECTION ( 'NONE',  ( 0.000000000000000000, 0.000000000000000000, 1.000000000000000000 ) ) ;
#2952=AXIS2_PLACEMENT_3D ( 'NONE', #18531, #2551, #3760 ) ;
#2953=LINE ( 'NONE', #11296, #903 ) ;
#2955=DIRECTION ( 'NONE',  ( -0.1566598588826321192, 0.9876526153536342445, 7.798540720466731404E-17 ) ) ;
#2957=CARTESIAN_POINT ( 'NONE',  ( -8.476787456656362352, -79.29982833240114815, -21.65063509461098690 ) ) ;
#2958=VECTOR ( 'NONE', #13636, 1000.000000000000000 ) ;
#2959=AXIS2_PLACEMENT_3D ( 'NONE', #17065, #4236, #11608 ) ;
#2960=CARTESIAN_POINT ( 'NONE',  ( -51.27495791377661760, -23.32042782179675200, 12.99038105676661736 ) ) ;
#2961=DIRECTION ( 'NONE',  ( -0.1566598588826321192, 0.9876526153536342445, 7.798540720466730171E-17 ) ) ;
#2962=AXIS2_PLACEMENT_3D ( 'NONE', #11344, #1426, #8893 ) ;
#2965=VERTEX_POINT ( 'NONE', #747 ) ;
#2967=EDGE_CURVE ( 'NONE', #13690, #14963, #3552, .T. ) ;
#2968=DIRECTION ( 'NONE',  ( -0.9876526153536341335, -0.1566598588826327021, 0.000000000000000000 ) ) ;
#2969=DIRECTION ( 'NONE',  ( -0.1566598588826321192, 0.9876526153536342445, 7.798540720466731404E-17 ) ) ;
#2971=ORIENTED_EDGE ( 'NONE', *, *, #191, .T. ) ;
#2972=DIRECTION ( 'NONE',  ( -0.1566598588826321192, 0.9876526153536342445, 7.798540720466730171E-17 ) ) ;
#2973=EDGE_CURVE ( 'NONE', #16508, #13410, #8109, .T. ) ;
#2974=ORIENTED_EDGE ( 'NONE', *, *, #11771, .T. ) ;
#2975=CIRCLE ( 'NONE', #10242, 1.500000000000000444 ) ;
#2976=CIRCLE ( 'NONE', #1200, 1.500000000000000888 ) ;
#2977=DIRECTION ( 'NONE',  ( -0.1566598588826321747, 0.9876526153536343555, 0.000000000000000000 ) ) ;
#2978=CARTESIAN_POINT ( 'NONE',  ( -51.97313754239392125, -28.49368068688882261, 12.99038105676661736 ) ) ;
#2980=ORIENTED_EDGE ( 'NONE', *, *, #492, .T. ) ;
#2981=VECTOR ( 'NONE', #14334, 1000.000000000000000 ) ;
#2983=ADVANCED_FACE ( 'NONE', ( #13615 ), #10756, .F. ) ;
#2984=CIRCLE ( 'NONE', #13574, 1.500000000000001332 ) ;
#2985=LINE ( 'NONE', #17248, #2922 ) ;
#2987=CIRCLE ( 'NONE', #8458, 1.500000000000000888 ) ;
#2988=EDGE_LOOP ( 'NONE', ( #6583, #13387, #15258, #4299 ) ) ;
#2989=LINE ( 'NONE', #7377, #6400 ) ;
#2990=VERTEX_POINT ( 'NONE', #12184 ) ;
#2991=CIRCLE ( 'NONE', #16020, 1.499999999999999556 ) ;
#2992=CYLINDRICAL_SURFACE ( 'NONE', #11129, 1.500000000000001554 ) ;
#2993=EDGE_LOOP ( 'NONE', ( #10365, #3487, #195, #4253 ) ) ;
#2994=EDGE_CURVE ( 'NONE', #1938, #9527, #4772, .T. ) ;
#2995=EDGE_CURVE ( 'NONE', #999, #12526, #12653, .T. ) ;
#2996=DIRECTION ( 'NONE',  ( -0.1566598588826321747, 0.9876526153536343555, 0.000000000000000000 ) ) ;
#2997=EDGE_LOOP ( 'NONE', ( #16490, #7785 ) ) ;
#2999=ORIENTED_EDGE ( 'NONE', *, *, #14727, .T. ) ;
#3000=AXIS2_PLACEMENT_3D ( 'NONE', #6875, #5042, #5156 ) ;
#3002=DIRECTION ( 'NONE',  ( -0.1566598588826321192, 0.9876526153536342445, 7.798540720466731404E-17 ) ) ;
#3003=CIRCLE ( 'NONE', #7565, 1.500000000000000888 ) ;
#3004=CARTESIAN_POINT ( 'NONE',  ( -66.25446545484369665, -88.46443007703511796, -12.99038105676658539 ) ) ;
#3006=AXIS2_PLACEMENT_3D ( 'NONE', #17654, #7826, #14674 ) ;
#3007=CIRCLE ( 'NONE', #7557, 1.500000000000000444 ) ;
#3008=EDGE_LOOP ( 'NONE', ( #16125, #14065, #17785, #18030 ) ) ;
#3009=CARTESIAN_POINT ( 'NONE',  ( -44.85521591397802155, -22.30213873905965016, 12.99038105676661736 ) ) ;
#3011=LINE ( 'NONE', #7215, #15376 ) ;
#3013=ORIENTED_EDGE ( 'NONE', *, *, #1702, .T. ) ;
#3015=FACE_BOUND ( 'NONE', #3640, .T. ) ;
#3016=CIRCLE ( 'NONE', #16041, 1.500000000000001332 ) ;
#3018=CIRCLE ( 'NONE', #12071, 1.500000000000000000 ) ;
#3020=ORIENTED_EDGE ( 'NONE', *, *, #9089, .T. ) ;
#3021=CIRCLE ( 'NONE', #13014, 1.500000000000000888 ) ;
#3022=EDGE_CURVE ( 'NONE', #11092, #17712, #18438, .T. ) ;
#3024=CARTESIAN_POINT ( 'NONE',  ( -32.67427653282027933, -83.13799487502562613, 17.32050807568881368 ) ) ;
#3025=VECTOR ( 'NONE', #709, 1000.000000000000000 ) ;
#3026=ORIENTED_EDGE ( 'NONE', *, *, #13251, .F. ) ;
#3028=DIRECTION ( 'NONE',  ( -0.1566598588826321192, 0.9876526153536342445, 7.798540720466731404E-17 ) ) ;
#3029=DIRECTION ( 'NONE',  ( -0.1566598588826321192, 0.9876526153536342445, 7.798540720466731404E-17 ) ) ;
#3030=EDGE_LOOP ( 'NONE', ( #8367, #11077 ) ) ;
#3031=CIRCLE ( 'NONE', #13614, 1.500000000000001332 ) ;
#3032=DIRECTION ( 'NONE',  ( -0.9876526153536341335, -0.1566598588826327021, 0.000000000000000000 ) ) ;
#3033=CIRCLE ( 'NONE', #1540, 1.500000000000000000 ) ;
#3035=AXIS2_PLACEMENT_3D ( 'NONE', #10057, #8460, #11560 ) ;
#3038=DIRECTION ( 'NONE',  ( 0.000000000000000000, 0.000000000000000000, 1.000000000000000000 ) ) ;
#3039=VECTOR ( 'NONE', #11130, 1000.000000000000000 ) ;
#3040=EDGE_LOOP ( 'NONE', ( #6079, #12116 ) ) ;
#3041=FACE_BOUND ( 'NONE', #12525, .T. ) ;
#3043=ORIENTED_EDGE ( 'NONE', *, *, #14558, .F. ) ;
#3045=DIRECTION ( 'NONE',  ( -0.1566598588826321192, 0.9876526153536342445, 7.798540720466730171E-17 ) ) ;
#3047=AXIS2_PLACEMENT_3D ( 'NONE', #5656, #18602, #5474 ) ;
#3048=DIRECTION ( 'NONE',  ( -0.9876526153536341335, -0.1566598588826327021, 0.000000000000000000 ) ) ;
#3049=AXIS2_PLACEMENT_3D ( 'NONE', #16181, #3261, #7554 ) ;
#3050=ORIENTED_EDGE ( 'NONE', *, *, #11365, .T. ) ;
#3051=EDGE_LOOP ( 'NONE', ( #594, #13177, #15838, #8981 ) ) ;
#3052=ORIENTED_EDGE ( 'NONE', *, *, #7099, .F. ) ;
#3053=ORIENTED_EDGE ( 'NONE', *, *, #9542, .T. ) ;
#3055=EDGE_CURVE ( 'NONE', #7702, #344, #2623, .T. ) ;
#3056=VECTOR ( 'NONE', #4496, 1000.000000000000000 ) ;
#3057=DIRECTION ( 'NONE',  ( -0.1566598588826321192, 0.9876526153536342445, 7.798540720466731404E-17 ) ) ;
#3058=EDGE_CURVE ( 'NONE', #62, #14796, #11979, .T. ) ;
#3059=ORIENTED_EDGE ( 'NONE', *, *, #15182, .T. ) ;
#3060=VERTEX_POINT ( 'NONE', #9914 ) ;
#3063=AXIS2_PLACEMENT_3D ( 'NONE', #4292, #10068, #12714 ) ;
#3064=CYLINDRICAL_SURFACE ( 'NONE', #10599, 1.500000000000000888 ) ;
#3065=DIRECTION ( 'NONE',  ( -0.1566598588826321192, 0.9876526153536342445, 7.798540720466730171E-17 ) ) ;
#3068=CARTESIAN_POINT ( 'NONE',  ( -54.44226908077801141, -28.88533033409540351, 1.869203119972154228E-14 ) ) ;
#3070=VERTEX_POINT ( 'NONE', #8130 ) ;
#3071=CYLINDRICAL_SURFACE ( 'NONE', #15386, 1.500000000000001554 ) ;
#3072=CARTESIAN_POINT ( 'NONE',  ( -13.45468554360235203, -22.38394619046619383, -17.32050807568878170 ) ) ;
#3073=CIRCLE ( 'NONE', #17644, 1.500000000000000000 ) ;
#3075=EDGE_LOOP ( 'NONE', ( #14299, #12328 ) ) ;
#3076=CARTESIAN_POINT ( 'NONE',  ( -58.88670584986932965, -29.59029969906724844, -4.330127018922181215 ) ) ;
#3078=CARTESIAN_POINT ( 'NONE',  ( -39.13365354279672204, -26.45710252141460828, -4.330127018922181215 ) ) ;
#3079=EDGE_CURVE ( 'NONE', #1095, #5465, #1442, .T. ) ;
#3080=DIRECTION ( 'NONE',  ( 0.000000000000000000, 0.000000000000000000, 1.000000000000000000 ) ) ;
#3082=DIRECTION ( 'NONE',  ( -0.1566598588826321192, 0.9876526153536342445, 7.798540720466730171E-17 ) ) ;
#3084=ADVANCED_FACE ( 'NONE', ( #5289 ), #3941, .F. ) ;
#3085=CYLINDRICAL_SURFACE ( 'NONE', #6836, 1.500000000000001554 ) ;
#3086=ORIENTED_EDGE ( 'NONE', *, *, #11575, .F. ) ;
#3088=VECTOR ( 'NONE', #14399, 1000.000000000000000 ) ;
#3089=CARTESIAN_POINT ( 'NONE',  ( -23.12685837619818940, -18.85562184364174598, 21.65063509461101177 ) ) ;
#3090=ORIENTED_EDGE ( 'NONE', *, *, #467, .F. ) ;
#3091=ORIENTED_EDGE ( 'NONE', *, *, #15821, .T. ) ;
#3092=CARTESIAN_POINT ( 'NONE',  ( -60.36818477289978091, -29.82528948739120267, -21.65063509461098334 ) ) ;
#3093=VERTEX_POINT ( 'NONE', #11243 ) ;
#3094=EDGE_LOOP ( 'NONE', ( #10235, #15609 ) ) ;
#3096=CARTESIAN_POINT ( 'NONE',  ( 9.300959619709004755, -76.47995087251376845, -4.330127018922189208 ) ) ;
#3097=DIRECTION ( 'NONE',  ( -0.1566598588826321747, 0.9876526153536343555, 0.000000000000000000 ) ) ;
#3098=EDGE_CURVE ( 'NONE', #3317, #14743, #15520, .T. ) ;
#3099=CARTESIAN_POINT ( 'NONE',  ( -20.32861884089991023, -81.17974663899273935, 12.99038105676661203 ) ) ;
#3100=CARTESIAN_POINT ( 'NONE',  ( -5.059638313096497697, -21.05233738996382797, -8.660254037844383745 ) ) ;
#3101=CARTESIAN_POINT ( 'NONE',  ( -75.18297400320422241, -32.17518737063066681, 12.99038105676661736 ) ) ;
#3102=FACE_OUTER_BOUND ( 'NONE', #193, .T. ) ;
#3103=DIRECTION ( 'NONE',  ( -0.1566598588826321192, 0.9876526153536342445, 7.798540720466730171E-17 ) ) ;
#3104=DIRECTION ( 'NONE',  ( -0.1566598588826321747, 0.9876526153536343555, 0.000000000000000000 ) ) ;
#3106=DIRECTION ( 'NONE',  ( -0.9876526153536341335, -0.1566598588826327021, 0.000000000000000000 ) ) ;
#3109=ORIENTED_EDGE ( 'NONE', *, *, #15067, .F. ) ;
#3110=ORIENTED_EDGE ( 'NONE', *, *, #13827, .F. ) ;
#3111=EDGE_LOOP ( 'NONE', ( #12315, #6151, #1508, #14266 ) ) ;
#3112=DIRECTION ( 'NONE',  ( -0.1566598588826321192, 0.9876526153536342445, 7.798540720466730171E-17 ) ) ;
#3113=CIRCLE ( 'NONE', #3399, 1.500000000000000000 ) ;
#3114=ORIENTED_EDGE ( 'NONE', *, *, #8242, .F. ) ;
#3115=ORIENTED_EDGE ( 'NONE', *, *, #11766, .T. ) ;
#3116=CARTESIAN_POINT ( 'NONE',  ( -4.361458684479201153, -15.87908452487173427, 17.32050807568881368 ) ) ;
#3117=EDGE_CURVE ( 'NONE', #4380, #6069, #9755, .T. ) ;
#3120=CARTESIAN_POINT ( 'NONE',  ( -33.99103714508810725, -20.57888029135069630, 8.660254037844417496 ) ) ;
#3121=EDGE_LOOP ( 'NONE', ( #13324, #1618, #17761, #5458 ) ) ;
#3122=EDGE_CURVE ( 'NONE', #4463, #16997, #17479, .T. ) ;
#3124=CIRCLE ( 'NONE', #9481, 1.500000000000000000 ) ;
#3125=EDGE_CURVE ( 'NONE', #10450, #11814, #7477, .T. ) ;
#3126=EDGE_LOOP ( 'NONE', ( #3180, #13855 ) ) ;
#3127=VERTEX_POINT ( 'NONE', #2724 ) ;
#3128=DIRECTION ( 'NONE',  ( -0.1566598588826321747, 0.9876526153536343555, 0.000000000000000000 ) ) ;
#3130=DIRECTION ( 'NONE',  ( -0.1566598588826321192, 0.9876526153536342445, 7.798540720466730171E-17 ) ) ;
#3131=ORIENTED_EDGE ( 'NONE', *, *, #14004, .F. ) ;
#3132=ORIENTED_EDGE ( 'NONE', *, *, #8587, .F. ) ;
#3133=ORIENTED_EDGE ( 'NONE', *, *, #11487, .T. ) ;
#3134=ORIENTED_EDGE ( 'NONE', *, *, #3540, .T. ) ;
#3135=CARTESIAN_POINT ( 'NONE',  ( -46.54104815794894279, -27.63205146303435100, 17.32050807568881723 ) ) ;
#3136=FACE_BOUND ( 'NONE', #15085, .T. ) ;
#3137=DIRECTION ( 'NONE',  ( 0.000000000000000000, 0.000000000000000000, 1.000000000000000000 ) ) ;
#3139=CARTESIAN_POINT ( 'NONE',  ( -21.84973277410820458, -23.71555499096855613, -8.660254037844380193 ) ) ;
#3140=ORIENTED_EDGE ( 'NONE', *, *, #6747, .F. ) ;
#3141=EDGE_LOOP ( 'NONE', ( #2632, #13388, #18583, #396 ) ) ;
#3142=FACE_BOUND ( 'NONE', #4869, .T. ) ;
#3143=ORIENTED_EDGE ( 'NONE', *, *, #15952, .T. ) ;
#3144=CARTESIAN_POINT ( 'NONE',  ( -53.74408945216070776, -23.71207746900332580, 1.908195823574487804E-14 ) ) ;
#3145=CARTESIAN_POINT ( 'NONE',  ( -17.40529600501688279, -23.01058562599671831, 21.65063509461101177 ) ) ;
#3146=EDGE_CURVE ( 'NONE', #855, #2319, #350, .T. ) ;
#3150=EDGE_CURVE ( 'NONE', #8286, #4960, #6034, .T. ) ;
#3151=ORIENTED_EDGE ( 'NONE', *, *, #3615, .T. ) ;
#3152=DIRECTION ( 'NONE',  ( -0.9876526153536336894, -0.1566598588826349503, 0.000000000000000000 ) ) ;
#3153=AXIS2_PLACEMENT_3D ( 'NONE', #2089, #10332, #9110 ) ;
#3154=LINE ( 'NONE', #1479, #2643 ) ;
#3155=FACE_OUTER_BOUND ( 'NONE', #8925, .T. ) ;
#3156=EDGE_LOOP ( 'NONE', ( #12323, #13204, #7873, #9776 ) ) ;
#3157=DIRECTION ( 'NONE',  ( -0.1566598588826321192, 0.9876526153536342445, 7.798540720466731404E-17 ) ) ;
#3159=DIRECTION ( 'NONE',  ( -0.1566598588826321192, 0.9876526153536342445, 7.798540720466730171E-17 ) ) ;
#3161=VERTEX_POINT ( 'NONE', #10188 ) ;
#3164=ADVANCED_FACE ( 'NONE', ( #6138 ), #75, .F. ) ;
#3165=CARTESIAN_POINT ( 'NONE',  ( -43.86756329862441817, -22.14547888017700572, -8.660254037844380193 ) ) ;
#3166=CARTESIAN_POINT ( 'NONE',  ( 0.4120860815263194254, -77.88988960245745830, -8.660254037844385522 ) ) ;
#3168=CARTESIAN_POINT ( 'NONE',  ( -66.08974714408107332, -25.67032570503623035, 21.65063509461102242 ) ) ;
#3169=VERTEX_POINT ( 'NONE', #8611 ) ;
#3170=EDGE_CURVE ( 'NONE', #15663, #4041, #3823, .T. ) ;
#3171=AXIS2_PLACEMENT_3D ( 'NONE', #14041, #13843, #12320 ) ;
#3172=ORIENTED_EDGE ( 'NONE', *, *, #13765, .T. ) ;
#3173=CYLINDRICAL_SURFACE ( 'NONE', #8496, 1.500000000000001554 ) ;
#3174=CARTESIAN_POINT ( 'NONE',  ( -27.28182215855319015, -24.57718421482303484, 4.330127018922217630 ) ) ;
#3177=AXIS2_PLACEMENT_3D ( 'NONE', #5182, #10943, #16770 ) ;
#3178=LINE ( 'NONE', #3099, #11292 ) ;
#3179=CARTESIAN_POINT ( 'NONE',  ( -4.526176995241833367, -78.67318889687062722, 8.660254037844408614 ) ) ;
#3180=ORIENTED_EDGE ( 'NONE', *, *, #8240, .T. ) ;
#3181=DIRECTION ( 'NONE',  ( -0.1566598588826321192, 0.9876526153536342445, 7.798540720466730171E-17 ) ) ;
#3183=AXIS2_PLACEMENT_3D ( 'NONE', #16892, #16989, #8345 ) ;
#3184=ORIENTED_EDGE ( 'NONE', *, *, #8240, .F. ) ;
#3185=DIRECTION ( 'NONE',  ( -0.1566598588826321747, 0.9876526153536343555, 0.000000000000000000 ) ) ;
#3186=DIRECTION ( 'NONE',  ( -0.9876526153536341335, -0.1566598588826327021, 0.000000000000000000 ) ) ;
#3189=EDGE_LOOP ( 'NONE', ( #9506, #18693, #12711, #10744 ) ) ;
#3190=CARTESIAN_POINT ( 'NONE',  ( -68.76323200340563346, -31.15689828789355786, 12.99038105676661736 ) ) ;
#3191=ORIENTED_EDGE ( 'NONE', *, *, #1172, .F. ) ;
#3192=CIRCLE ( 'NONE', #11953, 1.500000000000001332 ) ;
#3193=EDGE_CURVE ( 'NONE', #14599, #2583, #14384, .T. ) ;
#3194=ORIENTED_EDGE ( 'NONE', *, *, #12968, .T. ) ;
#3195=VERTEX_POINT ( 'NONE', #7193 ) ;
#3196=ORIENTED_EDGE ( 'NONE', *, *, #9202, .T. ) ;
#3198=CIRCLE ( 'NONE', #5352, 1.500000000000000444 ) ;
#3199=EDGE_LOOP ( 'NONE', ( #3658, #8523, #17690, #129 ) ) ;
#3202=DIRECTION ( 'NONE',  ( -0.1566598588826321192, 0.9876526153536342445, 7.798540720466731404E-17 ) ) ;
#3203=DIRECTION ( 'NONE',  ( -0.1566598588826321192, 0.9876526153536342445, 7.798540720466731404E-17 ) ) ;
#3205=CIRCLE ( 'NONE', #13799, 1.499999999999999556 ) ;
#3206=DIRECTION ( 'NONE',  ( -0.1566598588826321192, 0.9876526153536342445, 7.798540720466730171E-17 ) ) ;
#3207=CYLINDRICAL_SURFACE ( 'NONE', #1815, 1.500000000000001554 ) ;
#3208=DIRECTION ( 'NONE',  ( -0.1566598588826321192, 0.9876526153536342445, 7.798540720466731404E-17 ) ) ;
#3211=ORIENTED_EDGE ( 'NONE', *, *, #1319, .T. ) ;
#3214=DIRECTION ( 'NONE',  ( -0.1566598588826321192, 0.9876526153536342445, 7.798540720466730171E-17 ) ) ;
#3215=ORIENTED_EDGE ( 'NONE', *, *, #7887, .F. ) ;
#3216=EDGE_LOOP ( 'NONE', ( #16551, #503, #8590, #10451 ) ) ;
#3218=DIRECTION ( 'NONE',  ( -0.1566598588826321192, 0.9876526153536342445, 7.798540720466731404E-17 ) ) ;
#3219=ADVANCED_FACE ( 'NONE', ( #10289 ), #1672, .F. ) ;
#3221=FACE_BOUND ( 'NONE', #15340, .T. ) ;
#3222=EDGE_CURVE ( 'NONE', #11890, #16742, #829, .T. ) ;
#3223=DIRECTION ( 'NONE',  ( -0.9876526153536341335, -0.1566598588826327021, 0.000000000000000000 ) ) ;
#3224=ORIENTED_EDGE ( 'NONE', *, *, #16168, .F. ) ;
#3228=AXIS2_PLACEMENT_3D ( 'NONE', #4904, #9463, #7856 ) ;
#3229=VERTEX_POINT ( 'NONE', #4330 ) ;
#3232=CARTESIAN_POINT ( 'NONE',  ( -41.56315007100295844, -84.54793360496931598, -4.330127018922185655 ) ) ;
#3233=DIRECTION ( 'NONE',  ( -0.1566598588826321747, 0.9876526153536343555, 0.000000000000000000 ) ) ;
#3234=CARTESIAN_POINT ( 'NONE',  ( -41.56315007100295844, -84.54793360496931598, 4.330127018922213189 ) ) ;
#3235=DIRECTION ( 'NONE',  ( -0.1566598588826321192, 0.9876526153536342445, 7.798540720466730171E-17 ) ) ;
#3236=CARTESIAN_POINT ( 'NONE',  ( -12.46703292824873088, -22.22728633158356359, -4.330127018922181215 ) ) ;
#3237=ORIENTED_EDGE ( 'NONE', *, *, #15177, .T. ) ;
#3238=EDGE_LOOP ( 'NONE', ( #8742, #3638, #9483, #17486 ) ) ;
#3239=CARTESIAN_POINT ( 'NONE',  ( -47.81817376003895248, -22.77211831570752665, -21.65063509461098334 ) ) ;
#3240=DIRECTION ( 'NONE',  ( -0.1566598588826321192, 0.9876526153536342445, 7.798540720466730171E-17 ) ) ;
#3241=AXIS2_PLACEMENT_3D ( 'NONE', #13667, #16244, #3242 ) ;
#3242=DIRECTION ( 'NONE',  ( 0.000000000000000000, 0.000000000000000000, 1.000000000000000000 ) ) ;
#3245=ORIENTED_EDGE ( 'NONE', *, *, #15359, .F. ) ;
#3246=DIRECTION ( 'NONE',  ( -0.1566598588826321192, 0.9876526153536342445, 7.798540720466731404E-17 ) ) ;
#3247=AXIS2_PLACEMENT_3D ( 'NONE', #10957, #4801, #10592 ) ;
#3248=ADVANCED_FACE ( 'NONE', ( #17629 ), #1760, .F. ) ;
#3250=CIRCLE ( 'NONE', #15106, 1.499999999999999556 ) ;
#3251=DIRECTION ( 'NONE',  ( 0.000000000000000000, 0.000000000000000000, 1.000000000000000000 ) ) ;
#3252=DIRECTION ( 'NONE',  ( -0.1566598588826321747, 0.9876526153536343555, 0.000000000000000000 ) ) ;
#3254=AXIS2_PLACEMENT_3D ( 'NONE', #6643, #9769, #9566 ) ;
#3255=ORIENTED_EDGE ( 'NONE', *, *, #13564, .F. ) ;
#3256=CARTESIAN_POINT ( 'NONE',  ( -58.68235252892885256, -24.49537676341648762, 8.660254037844417496 ) ) ;
#3257=DIRECTION ( 'NONE',  ( -0.9876526153536336894, -0.1566598588826349503, 0.000000000000000000 ) ) ;
#3258=CARTESIAN_POINT ( 'NONE',  ( -42.09661138885763165, -26.92708209806250608, 12.99038105676661736 ) ) ;
#3259=VERTEX_POINT ( 'NONE', #13403 ) ;
#3260=EDGE_LOOP ( 'NONE', ( #16369, #2026 ) ) ;
#3261=DIRECTION ( 'NONE',  ( -0.1566598588826321747, 0.9876526153536343555, 0.000000000000000000 ) ) ;
#3263=VERTEX_POINT ( 'NONE', #11957 ) ;
#3264=CIRCLE ( 'NONE', #10820, 1.500000000000000888 ) ;
#3265=ORIENTED_EDGE ( 'NONE', *, *, #18344, .T. ) ;
#3266=DIRECTION ( 'NONE',  ( -0.1566598588826321192, 0.9876526153536342445, 7.798540720466731404E-17 ) ) ;
#3267=EDGE_CURVE ( 'NONE', #11861, #13426, #2628, .T. ) ;
#3270=FACE_OUTER_BOUND ( 'NONE', #15962, .T. ) ;
#3273=DIRECTION ( 'NONE',  ( -0.1566598588826321747, 0.9876526153536343555, 0.000000000000000000 ) ) ;
#3274=EDGE_CURVE ( 'NONE', #15309, #5835, #1140, .T. ) ;
#3275=DIRECTION ( 'NONE',  ( -0.9876526153536336894, -0.1566598588826349503, 0.000000000000000000 ) ) ;
#3276=AXIS2_PLACEMENT_3D ( 'NONE', #6252, #12089, #17937 ) ;
#3278=DIRECTION ( 'NONE',  ( -0.1566598588826321192, 0.9876526153536342445, 7.798540720466731404E-17 ) ) ;
#3279=CARTESIAN_POINT ( 'NONE',  ( -8.516422466834198346, -21.60064689605303911, 1.522258424776792809E-14 ) ) ;
#3281=CARTESIAN_POINT ( 'NONE',  ( 0.000000000000000000, 0.000000000000000000, 30.00000000000000000 ) ) ;
#3282=VERTEX_POINT ( 'NONE', #7828 ) ;
#3283=AXIS2_PLACEMENT_3D ( 'NONE', #3945, #14391, #5584 ) ;
#3286=VECTOR ( 'NONE', #3311, 1000.000000000000000 ) ;
#3287=VERTEX_POINT ( 'NONE', #7925 ) ;
#3288=ORIENTED_EDGE ( 'NONE', *, *, #833, .T. ) ;
#3289=FACE_OUTER_BOUND ( 'NONE', #16223, .T. ) ;
#3290=AXIS2_PLACEMENT_3D ( 'NONE', #6618, #9353, #13699 ) ;
#3291=CIRCLE ( 'NONE', #9687, 1.499999999999999556 ) ;
#3292=VECTOR ( 'NONE', #10736, 1000.000000000000000 ) ;
#3296=DIRECTION ( 'NONE',  ( -0.1566598588826321192, 0.9876526153536342445, 7.798540720466731404E-17 ) ) ;
#3297=AXIS2_PLACEMENT_3D ( 'NONE', #7847, #3903, #14854 ) ;
#3298=CIRCLE ( 'NONE', #13290, 1.500000000000000444 ) ;
#3299=ADVANCED_FACE ( 'NONE', ( #3633 ), #16754, .F. ) ;
#3300=CYLINDRICAL_SURFACE ( 'NONE', #6319, 1.500000000000001554 ) ;
#3301=DIRECTION ( 'NONE',  ( -0.1566598588826321192, 0.9876526153536342445, 7.798540720466731404E-17 ) ) ;
#3302=AXIS2_PLACEMENT_3D ( 'NONE', #6486, #13743, #10715 ) ;
#3303=DIRECTION ( 'NONE',  ( -0.1566598588826321192, 0.9876526153536342445, 7.798540720466730171E-17 ) ) ;
#3305=ORIENTED_EDGE ( 'NONE', *, *, #17292, .F. ) ;
#3306=AXIS2_PLACEMENT_3D ( 'NONE', #5358, #9889, #8002 ) ;
#3307=CARTESIAN_POINT ( 'NONE',  ( -15.71946376104596155, -17.68067290202200326, 1.908195823574487804E-14 ) ) ;
#3308=VERTEX_POINT ( 'NONE', #13870 ) ;
#3311=DIRECTION ( 'NONE',  ( -0.1566598588826321192, 0.9876526153536342445, 7.798540720466730171E-17 ) ) ;
#3312=ADVANCED_FACE ( 'NONE', ( #4396 ), #7264, .F. ) ;
#3313=VERTEX_POINT ( 'NONE', #3068 ) ;
#3315=VERTEX_POINT ( 'NONE', #6008 ) ;
#3316=AXIS2_PLACEMENT_3D ( 'NONE', #741, #11033, #16774 ) ;
#3317=VERTEX_POINT ( 'NONE', #17602 ) ;
#3318=DIRECTION ( 'NONE',  ( -0.1566598588826321192, 0.9876526153536342445, 7.798540720466730171E-17 ) ) ;
#3319=EDGE_LOOP ( 'NONE', ( #12347, #1645, #8615, #17813 ) ) ;
#3320=AXIS2_PLACEMENT_3D ( 'NONE', #9459, #10958, #1054 ) ;
#3321=FACE_BOUND ( 'NONE', #360, .T. ) ;
#3323=AXIS2_PLACEMENT_3D ( 'NONE', #2320, #12465, #6803 ) ;
#3324=ORIENTED_EDGE ( 'NONE', *, *, #14007, .T. ) ;
#3325=ORIENTED_EDGE ( 'NONE', *, *, #15865, .F. ) ;
#3327=AXIS2_PLACEMENT_3D ( 'NONE', #16452, #529, #8087 ) ;
#3328=EDGE_CURVE ( 'NONE', #4041, #15663, #8072, .T. ) ;
#3329=CARTESIAN_POINT ( 'NONE',  ( -69.54653129781877396, -26.21863521112543438, -4.330127018922180326 ) ) ;
#3331=CARTESIAN_POINT ( 'NONE',  ( -35.67686938905902849, -25.90879301532540779, -12.99038105676658006 ) ) ;
#3333=ADVANCED_FACE ( 'NONE', ( #16342 ), #6305, .F. ) ;
#3335=FACE_OUTER_BOUND ( 'NONE', #6010, .T. ) ;
#3336=ORIENTED_EDGE ( 'NONE', *, *, #2559, .T. ) ;
#3337=ORIENTED_EDGE ( 'NONE', *, *, #9952, .F. ) ;
#3338=DIRECTION ( 'NONE',  ( -0.1566598588826321192, 0.9876526153536342445, 7.798540720466730171E-17 ) ) ;
#3340=DIRECTION ( 'NONE',  ( 0.000000000000000000, 0.000000000000000000, 1.000000000000000000 ) ) ;
#3341=AXIS2_PLACEMENT_3D ( 'NONE', #18499, #12548, #932 ) ;
#3342=ORIENTED_EDGE ( 'NONE', *, *, #7989, .F. ) ;
#3343=ORIENTED_EDGE ( 'NONE', *, *, #8154, .F. ) ;
#3344=DIRECTION ( 'NONE',  ( -0.9876526153536344665, -0.1566598588826304539, 0.000000000000000000 ) ) ;
#3345=AXIS2_PLACEMENT_3D ( 'NONE', #7566, #17538, #8889 ) ;
#3347=EDGE_CURVE ( 'NONE', #8246, #18620, #6901, .T. ) ;
#3348=VECTOR ( 'NONE', #11570, 1000.000000000000000 ) ;
#3349=CARTESIAN_POINT ( 'NONE',  ( -7.818242838216901802, -16.42739403096095074, 17.32050807568881012 ) ) ;
#3351=ORIENTED_EDGE ( 'NONE', *, *, #5236, .T. ) ;
#3352=ADVANCED_FACE ( 'NONE', ( #3335 ), #12505, .F. ) ;
#3353=EDGE_CURVE ( 'NONE', #15259, #1477, #9887, .T. ) ;
#3354=DIRECTION ( 'NONE',  ( -0.9876526153536341335, -0.1566598588826327021, 0.000000000000000000 ) ) ;
#3356=VECTOR ( 'NONE', #5869, 1000.000000000000000 ) ;
#3358=DIRECTION ( 'NONE',  ( -0.9876526153536336894, -0.1566598588826349503, 0.000000000000000000 ) ) ;
#3359=VERTEX_POINT ( 'NONE', #3236 ) ;
#3360=ORIENTED_EDGE ( 'NONE', *, *, #15572, .F. ) ;
#3361=FACE_OUTER_BOUND ( 'NONE', #2587, .T. ) ;
#3363=CIRCLE ( 'NONE', #18564, 1.499999999999999556 ) ;
#3364=VERTEX_POINT ( 'NONE', #9034 ) ;
#3366=DIRECTION ( 'NONE',  ( -0.9876526153536344665, -0.1566598588826304539, 0.000000000000000000 ) ) ;
#3367=AXIS2_PLACEMENT_3D ( 'NONE', #14884, #17386, #17468 ) ;
#3369=ORIENTED_EDGE ( 'NONE', *, *, #6000, .T. ) ;
#3370=CARTESIAN_POINT ( 'NONE',  ( -35.67686938905904270, -25.90879301532540779, -21.65063509461098334 ) ) ;
#3371=CARTESIAN_POINT ( 'NONE',  ( -9.464440072009985272, -79.45648819128378193, 17.32050807568880657 ) ) ;
#3372=CARTESIAN_POINT ( 'NONE',  ( -76.17062661855784711, -32.33184722951329348, 8.660254037844417496 ) ) ;
#3373=CARTESIAN_POINT ( 'NONE',  ( -3.044698072211382112, -78.43819910854666944, 8.660254037844408614 ) ) ;
#3374=CYLINDRICAL_SURFACE ( 'NONE', #18458, 1.500000000000001554 ) ;
#3375=CARTESIAN_POINT ( 'NONE',  ( -20.32861884089991023, -81.17974663899272514, 4.330127018922213189 ) ) ;
#3377=ORIENTED_EDGE ( 'NONE', *, *, #16026, .F. ) ;
#3378=EDGE_CURVE ( 'NONE', #18416, #16068, #325, .T. ) ;
#3379=CIRCLE ( 'NONE', #8259, 1.500000000000000000 ) ;
#3380=EDGE_CURVE ( 'NONE', #12090, #3317, #18738, .T. ) ;
#3381=CARTESIAN_POINT ( 'NONE',  ( -23.33121169713865584, -23.95054477929251036, 1.869203119972154228E-14 ) ) ;
#3383=EDGE_LOOP ( 'NONE', ( #13747, #12542 ) ) ;
#3384=LINE ( 'NONE', #11819, #1432 ) ;
#3385=CIRCLE ( 'NONE', #10019, 1.500000000000000888 ) ;
#3386=CYLINDRICAL_SURFACE ( 'NONE', #7042, 1.500000000000000888 ) ;
#3387=LINE ( 'NONE', #8910, #7965 ) ;
#3388=LINE ( 'NONE', #18242, #1544 ) ;
#3392=LINE ( 'NONE', #9198, #11128 ) ;
#3393=CARTESIAN_POINT ( 'NONE',  ( -67.07739975943471222, -25.82698556391886413, 17.32050807568881723 ) ) ;
#3394=DIRECTION ( 'NONE',  ( -0.1566598588826321192, 0.9876526153536342445, 7.798540720466730171E-17 ) ) ;
#3395=CARTESIAN_POINT ( 'NONE',  ( -44.03228160938703439, -84.93958325217590755, 1.424741226644455312E-14 ) ) ;
#3398=ORIENTED_EDGE ( 'NONE', *, *, #18359, .F. ) ;
#3399=AXIS2_PLACEMENT_3D ( 'NONE', #12884, #8824, #16023 ) ;
#3401=DIRECTION ( 'NONE',  ( -0.1566598588826321192, 0.9876526153536342445, 7.798540720466730171E-17 ) ) ;
#3402=LINE ( 'NONE', #16136, #18791 ) ;
#3403=ADVANCED_FACE ( 'NONE', ( #16897 ), #6751, .F. ) ;
#3404=ORIENTED_EDGE ( 'NONE', *, *, #2406, .T. ) ;
#3405=ORIENTED_EDGE ( 'NONE', *, *, #2081, .F. ) ;
#3407=ORIENTED_EDGE ( 'NONE', *, *, #13160, .F. ) ;
#3408=DIRECTION ( 'NONE',  ( -0.1566598588826321192, 0.9876526153536342445, 7.798540720466731404E-17 ) ) ;
#3409=EDGE_CURVE ( 'NONE', #12681, #1415, #13291, .T. ) ;
#3410=ORIENTED_EDGE ( 'NONE', *, *, #3122, .F. ) ;
#3411=FACE_BOUND ( 'NONE', #14343, .T. ) ;
#3412=ORIENTED_EDGE ( 'NONE', *, *, #15297, .T. ) ;
#3414=CYLINDRICAL_SURFACE ( 'NONE', #14310, 1.500000000000001554 ) ;
#3415=EDGE_LOOP ( 'NONE', ( #4201, #12118, #18417, #14824 ) ) ;
#3417=ORIENTED_EDGE ( 'NONE', *, *, #8627, .F. ) ;
#3418=CARTESIAN_POINT ( 'NONE',  ( -38.92930022185625205, -21.36217958576385456, 8.660254037844417496 ) ) ;
#3419=ORIENTED_EDGE ( 'NONE', *, *, #13997, .F. ) ;
#3421=DIRECTION ( 'NONE',  ( -0.9876526153536341335, -0.1566598588826327021, 0.000000000000000000 ) ) ;
#3422=CARTESIAN_POINT ( 'NONE',  ( -71.02801022084922522, -26.45362499944938861, 21.65063509461102242 ) ) ;
#3423=DIRECTION ( 'NONE',  ( -0.1566598588826321747, 0.9876526153536343555, 0.000000000000000000 ) ) ;
#3425=VERTEX_POINT ( 'NONE', #7804 ) ;
#3426=EDGE_LOOP ( 'NONE', ( #14987, #10223 ) ) ;
#3428=CYLINDRICAL_SURFACE ( 'NONE', #16355, 1.500000000000001554 ) ;
#3431=ORIENTED_EDGE ( 'NONE', *, *, #12952, .T. ) ;
#3433=ORIENTED_EDGE ( 'NONE', *, *, #3792, .T. ) ;
#3436=CYLINDRICAL_SURFACE ( 'NONE', #5441, 1.500000000000001554 ) ;
#3437=CARTESIAN_POINT ( 'NONE',  ( -21.64537945316773460, -18.62063205531779531, -12.99038105676658006 ) ) ;
#3440=VERTEX_POINT ( 'NONE', #10449 ) ;
#3441=CYLINDRICAL_SURFACE ( 'NONE', #8641, 1.500000000000001554 ) ;
#3443=EDGE_LOOP ( 'NONE', ( #7347, #604, #4068, #11841 ) ) ;
#3444=CARTESIAN_POINT ( 'NONE',  ( -61.84966369593024638, -30.06027927571514624, 4.330127018922217630 ) ) ;
#3446=ORIENTED_EDGE ( 'NONE', *, *, #13764, .F. ) ;
#3447=ORIENTED_EDGE ( 'NONE', *, *, #4114, .F. ) ;
#3448=EDGE_CURVE ( 'NONE', #12256, #14889, #11267, .T. ) ;
#3449=EDGE_CURVE ( 'NONE', #18006, #1662, #7044, .T. ) ;
#3450=EDGE_CURVE ( 'NONE', #898, #4657, #5602, .T. ) ;
#3451=AXIS2_PLACEMENT_3D ( 'NONE', #9482, #2184, #6556 ) ;
#3452=CARTESIAN_POINT ( 'NONE',  ( -61.31620237807555895, -87.68113078262194904, -4.330127018922185655 ) ) ;
#3453=EDGE_CURVE ( 'NONE', #14006, #14647, #218, .T. ) ;
#3454=DIRECTION ( 'NONE',  ( -0.1566598588826321747, 0.9876526153536343555, 0.000000000000000000 ) ) ;
#3455=ADVANCED_FACE ( 'NONE', ( #5084 ), #9360, .F. ) ;
#3458=DIRECTION ( 'NONE',  ( -0.9876526153536341335, -0.1566598588826327021, 0.000000000000000000 ) ) ;
#3461=CARTESIAN_POINT ( 'NONE',  ( -20.86208015875457988, -23.55889513208593655, -21.65063509461098334 ) ) ;
#3462=CARTESIAN_POINT ( 'NONE',  ( -23.12685837619818940, -18.85562184364174598, 12.99038105676661736 ) ) ;
#3463=DIRECTION ( 'NONE',  ( -0.9876526153536336894, -0.1566598588826349503, 0.000000000000000000 ) ) ;
#3464=FACE_OUTER_BOUND ( 'NONE', #11568, .T. ) ;
#3465=AXIS2_PLACEMENT_3D ( 'NONE', #4100, #11216, #9525 ) ;
#3466=DIRECTION ( 'NONE',  ( -0.1566598588826321192, 0.9876526153536342445, 7.798540720466730171E-17 ) ) ;
#3467=DIRECTION ( 'NONE',  ( 0.000000000000000000, 0.000000000000000000, 1.000000000000000000 ) ) ;
#3468=VERTEX_POINT ( 'NONE', #847 ) ;
#3469=CARTESIAN_POINT ( 'NONE',  ( -75.18297400320422241, -32.17518737063066681, -12.99038105676658006 ) ) ;
#3470=VERTEX_POINT ( 'NONE', #12382 ) ;
#3471=ORIENTED_EDGE ( 'NONE', *, *, #16638, .T. ) ;
#3472=ADVANCED_FACE ( 'NONE', ( #6354 ), #10595, .F. ) ;
#3473=VERTEX_POINT ( 'NONE', #18022 ) ;
#3474=CARTESIAN_POINT ( 'NONE',  ( -21.81009776393036503, -81.41473642731669713, 12.99038105676661203 ) ) ;
#3475=ADVANCED_FACE ( 'NONE', ( #16482 ), #9552, .F. ) ;
#3476=CARTESIAN_POINT ( 'NONE',  ( -35.14340807120436239, -83.52964452223220349, -12.99038105676658539 ) ) ;
#3477=CIRCLE ( 'NONE', #5929, 1.500000000000000888 ) ;
#3479=CARTESIAN_POINT ( 'NONE',  ( 5.350349158294472218, -77.10659030804430358, 17.32050807568880657 ) ) ;
#3480=DIRECTION ( 'NONE',  ( -0.9876526153536336894, -0.1566598588826349503, 0.000000000000000000 ) ) ;
#3481=EDGE_CURVE ( 'NONE', #311, #14160, #11996, .T. ) ;
#3482=EDGE_CURVE ( 'NONE', #7247, #7443, #11423, .T. ) ;
#3483=DIRECTION ( 'NONE',  ( -0.1566598588826321192, 0.9876526153536342445, 7.798540720466730171E-17 ) ) ;
#3484=DIRECTION ( 'NONE',  ( 0.000000000000000000, 0.000000000000000000, 1.000000000000000000 ) ) ;
#3485=ORIENTED_EDGE ( 'NONE', *, *, #10745, .F. ) ;
#3486=DIRECTION ( 'NONE',  ( -0.9876526153536336894, -0.1566598588826349503, 0.000000000000000000 ) ) ;
#3487=ORIENTED_EDGE ( 'NONE', *, *, #17924, .F. ) ;
#3488=FACE_BOUND ( 'NONE', #2050, .T. ) ;
#3489=SURFACE_STYLE_USAGE ( .BOTH. , #16499 ) ;
#3491=CARTESIAN_POINT ( 'NONE',  ( -58.88670584986932965, -29.59029969906724844, -21.65063509461098334 ) ) ;
#3493=AXIS2_PLACEMENT_3D ( 'NONE', #12500, #5312, #12581 ) ;
#3494=VERTEX_POINT ( 'NONE', #2823 ) ;
#3497=DIRECTION ( 'NONE',  ( -0.9876526153536336894, -0.1566598588826350336, 0.000000000000000000 ) ) ;
#3498=FACE_BOUND ( 'NONE', #6231, .T. ) ;
#3499=AXIS2_PLACEMENT_3D ( 'NONE', #17963, #4742, #9119 ) ;
#3500=DIRECTION ( 'NONE',  ( -0.1566598588826321747, 0.9876526153536343555, 0.000000000000000000 ) ) ;
#3501=VERTEX_POINT ( 'NONE', #12563 ) ;
#3502=EDGE_CURVE ( 'NONE', #9820, #17699, #18451, .T. ) ;
#3503=AXIS2_PLACEMENT_3D ( 'NONE', #5196, #3743, #9547 ) ;
#3504=EDGE_CURVE ( 'NONE', #1028, #5886, #2043, .T. ) ;
#3505=CARTESIAN_POINT ( 'NONE',  ( -50.49165861936349131, -28.25869089856488614, -21.65063509461098334 ) ) ;
#3507=CARTESIAN_POINT ( 'NONE',  ( 0.5768043922889515285, -15.09578523045857601, 8.660254037844412167 ) ) ;
#3508=DIRECTION ( 'NONE',  ( 0.000000000000000000, 0.000000000000000000, 1.000000000000000000 ) ) ;
#3511=ORIENTED_EDGE ( 'NONE', *, *, #17053, .T. ) ;
#3512=ORIENTED_EDGE ( 'NONE', *, *, #9056, .T. ) ;
#3514=CIRCLE ( 'NONE', #513, 1.500000000000000444 ) ;
#3515=LINE ( 'NONE', #14725, #16581 ) ;
#3516=EDGE_LOOP ( 'NONE', ( #17717, #16519, #12790, #7153 ) ) ;
#3518=CIRCLE ( 'NONE', #18723, 1.500000000000001332 ) ;
#3520=VERTEX_POINT ( 'NONE', #11247 ) ;
#3521=DIRECTION ( 'NONE',  ( 0.9876526153536342445, 0.1566598588826321470, 6.424890667364402638E-17 ) ) ;
#3522=CIRCLE ( 'NONE', #14135, 1.500000000000000888 ) ;
#3523=DIRECTION ( 'NONE',  ( -0.9876526153536341335, -0.1566598588826327021, 0.000000000000000000 ) ) ;
#3524=VECTOR ( 'NONE', #10270, 1000.000000000000000 ) ;
#3526=DIRECTION ( 'NONE',  ( -0.1566598588826321192, 0.9876526153536342445, 7.798540720466731404E-17 ) ) ;
#3527=DIRECTION ( 'NONE',  ( -0.9876526153536341335, -0.1566598588826327021, 0.000000000000000000 ) ) ;
#3528=EDGE_CURVE ( 'NONE', #9211, #17125, #2338, .T. ) ;
#3529=CARTESIAN_POINT ( 'NONE',  ( -51.43967622453925514, -86.11453219379563961, 12.99038105676661203 ) ) ;
#3531=ORIENTED_EDGE ( 'NONE', *, *, #708, .T. ) ;
#3532=CIRCLE ( 'NONE', #9608, 1.500000000000001332 ) ;
#3533=DIRECTION ( 'NONE',  ( -0.1566598588826321747, 0.9876526153536343555, 0.000000000000000000 ) ) ;
#3534=DIRECTION ( 'NONE',  ( 0.000000000000000000, 0.000000000000000000, 1.000000000000000000 ) ) ;
#3535=CARTESIAN_POINT ( 'NONE',  ( -6.830590222863280658, -16.27073417207831696, -21.65063509461097979 ) ) ;
#3538=FACE_OUTER_BOUND ( 'NONE', #16194, .T. ) ;
#3539=ORIENTED_EDGE ( 'NONE', *, *, #7966, .F. ) ;
#3540=EDGE_CURVE ( 'NONE', #10934, #11092, #11051, .T. ) ;
#3541=CARTESIAN_POINT ( 'NONE',  ( -21.81009776393036503, -81.41473642731669713, 12.99038105676661203 ) ) ;
#3542=ORIENTED_EDGE ( 'NONE', *, *, #10944, .T. ) ;
#3544=DIRECTION ( 'NONE',  ( -0.1566598588826321192, 0.9876526153536342445, 7.798540720466731404E-17 ) ) ;
#3545=AXIS2_PLACEMENT_3D ( 'NONE', #9200, #7774, #12201 ) ;
#3546=CARTESIAN_POINT ( 'NONE',  ( -37.44782129882580080, -21.12718979743991099, 8.660254037844417496 ) ) ;
#3548=LINE ( 'NONE', #3737, #1346 ) ;
#3549=ORIENTED_EDGE ( 'NONE', *, *, #6813, .F. ) ;
#3550=DIRECTION ( 'NONE',  ( -0.1566598588826321192, 0.9876526153536342445, 7.798540720466730171E-17 ) ) ;
#3551=CARTESIAN_POINT ( 'NONE',  ( -55.22556837519114481, -23.94706725732728003, 17.32050807568881723 ) ) ;
#3552=CIRCLE ( 'NONE', #2669, 1.500000000000001332 ) ;
#3553=CARTESIAN_POINT ( 'NONE',  ( -11.97320662057189899, -22.14895640214223960, 1.887572821959364500E-14 ) ) ;
#3554=AXIS2_PLACEMENT_3D ( 'NONE', #11191, #9312, #11093 ) ;
#3555=FACE_OUTER_BOUND ( 'NONE', #8307, .T. ) ;
#3556=EDGE_CURVE ( 'NONE', #11687, #4660, #15055, .T. ) ;
#3557=AXIS2_PLACEMENT_3D ( 'NONE', #4916, #6548, #18039 ) ;
#3559=CIRCLE ( 'NONE', #9325, 1.500000000000000888 ) ;
#3560=DIRECTION ( 'NONE',  ( -0.9876526153536341335, -0.1566598588826327021, 0.000000000000000000 ) ) ;
#3562=CARTESIAN_POINT ( 'NONE',  ( -41.39843176024034221, -21.75382923297042481, -12.99038105676658006 ) ) ;
#3563=VERTEX_POINT ( 'NONE', #15430 ) ;
#3564=EDGE_CURVE ( 'NONE', #1595, #2455, #2451, .T. ) ;
#3565=CARTESIAN_POINT ( 'NONE',  ( -4.526176995241833367, -78.67318889687062722, 1.424741226644455312E-14 ) ) ;
#3567=ORIENTED_EDGE ( 'NONE', *, *, #4933, .F. ) ;
#3568=AXIS2_PLACEMENT_3D ( 'NONE', #15277, #6774, #3886 ) ;
#3569=LINE ( 'NONE', #13712, #4281 ) ;
#3570=AXIS2_PLACEMENT_3D ( 'NONE', #16568, #9077, #841 ) ;
#3574=FACE_OUTER_BOUND ( 'NONE', #6085, .T. ) ;
#3575=DIRECTION ( 'NONE',  ( -0.1566598588826321192, 0.9876526153536342445, 7.798540720466730171E-17 ) ) ;
#3576=ORIENTED_EDGE ( 'NONE', *, *, #9854, .F. ) ;
#3577=CARTESIAN_POINT ( 'NONE',  ( -28.06512145296634486, -19.63892113805490780, 12.99038105676661736 ) ) ;
#3578=EDGE_CURVE ( 'NONE', #3908, #16065, #6299, .T. ) ;
#3580=CIRCLE ( 'NONE', #6632, 1.499999999999999556 ) ;
#3582=CARTESIAN_POINT ( 'NONE',  ( -29.21749237908258223, -82.58968536893641499, -8.660254037844385522 ) ) ;
#3583=DIRECTION ( 'NONE',  ( -0.1566598588826321192, 0.9876526153536342445, 7.798540720466731404E-17 ) ) ;
#3584=CARTESIAN_POINT ( 'NONE',  ( -25.10216360690543524, -19.16894156140700289, -21.65063509461098334 ) ) ;
#3585=VECTOR ( 'NONE', #3130, 1000.000000000000000 ) ;
#3586=VECTOR ( 'NONE', #14652, 1000.000000000000000 ) ;
#3587=FACE_OUTER_BOUND ( 'NONE', #16613, .T. ) ;
#3588=CIRCLE ( 'NONE', #14205, 1.500000000000000888 ) ;
#3591=VERTEX_POINT ( 'NONE', #3943 ) ;
#3592=EDGE_LOOP ( 'NONE', ( #8832, #3938 ) ) ;
#3594=FACE_BOUND ( 'NONE', #188, .T. ) ;
#3595=VECTOR ( 'NONE', #15570, 1000.000000000000000 ) ;
#3596=CARTESIAN_POINT ( 'NONE',  ( -69.54653129781877396, -26.21863521112542728, -21.65063509461098334 ) ) ;
#3597=AXIS2_PLACEMENT_3D ( 'NONE', #11931, #9218, #7801 ) ;
#3598=ORIENTED_EDGE ( 'NONE', *, *, #13598, .T. ) ;
#3599=CIRCLE ( 'NONE', #17283, 1.500000000000000444 ) ;
#3600=AXIS2_PLACEMENT_3D ( 'NONE', #772, #5225, #2269 ) ;
#3602=VERTEX_POINT ( 'NONE', #12766 ) ;
#3603=LINE ( 'NONE', #9413, #11476 ) ;
#3604=CIRCLE ( 'NONE', #5762, 1.500000000000001332 ) ;
#3605=DIRECTION ( 'NONE',  ( -0.1566598588826321192, 0.9876526153536342445, 7.798540720466730171E-17 ) ) ;
#3606=ORIENTED_EDGE ( 'NONE', *, *, #11384, .T. ) ;
#3607=ORIENTED_EDGE ( 'NONE', *, *, #9925, .T. ) ;
#3608=CARTESIAN_POINT ( 'NONE',  ( -29.75095369693726610, -24.96883386202961574, 17.32050807568881723 ) ) ;
#3609=AXIS2_PLACEMENT_3D ( 'NONE', #7340, #16395, #3560 ) ;
#3610=EDGE_CURVE ( 'NONE', #9493, #18706, #3154, .T. ) ;
#3611=DIRECTION ( 'NONE',  ( 0.000000000000000000, 0.000000000000000000, 1.000000000000000000 ) ) ;
#3612=ORIENTED_EDGE ( 'NONE', *, *, #2540, .F. ) ;
#3615=EDGE_CURVE ( 'NONE', #3470, #13701, #17508, .T. ) ;
#3617=CARTESIAN_POINT ( 'NONE',  ( -6.047290928450125946, -21.20899724884646531, 21.65063509461101177 ) ) ;
#3618=LINE ( 'NONE', #8293, #12365 ) ;
#3619=EDGE_CURVE ( 'NONE', #11326, #3894, #1170, .T. ) ;
#3620=DIRECTION ( 'NONE',  ( -0.1566598588826321192, 0.9876526153536342445, 7.798540720466730171E-17 ) ) ;
#3621=CIRCLE ( 'NONE', #7004, 1.499999999999999556 ) ;
#3623=CARTESIAN_POINT ( 'NONE',  ( -6.047290928450125946, -21.20899724884646531, -4.330127018922184767 ) ) ;
#3625=EDGE_LOOP ( 'NONE', ( #5272, #13445, #10394, #10220 ) ) ;
#3626=AXIS2_PLACEMENT_3D ( 'NONE', #14421, #4178, #2940 ) ;
#3627=DIRECTION ( 'NONE',  ( -0.1566598588826321192, 0.9876526153536342445, 7.798540720466731404E-17 ) ) ;
#3628=AXIS2_PLACEMENT_3D ( 'NONE', #3791, #14043, #15375 ) ;
#3629=PLANE ( 'NONE',  #8081 ) ;
#3630=EDGE_LOOP ( 'NONE', ( #14623, #14621 ) ) ;
#3632=DIRECTION ( 'NONE',  ( -0.1566598588826321192, 0.9876526153536342445, 7.798540720466731404E-17 ) ) ;
#3633=FACE_OUTER_BOUND ( 'NONE', #4984, .T. ) ;
#3634=ORIENTED_EDGE ( 'NONE', *, *, #2033, .T. ) ;
#3635=VERTEX_POINT ( 'NONE', #58 ) ;
#3636=DIRECTION ( 'NONE',  ( 0.000000000000000000, 0.000000000000000000, 1.000000000000000000 ) ) ;
#3638=ORIENTED_EDGE ( 'NONE', *, *, #14918, .F. ) ;
#3639=VECTOR ( 'NONE', #12366, 1000.000000000000000 ) ;
#3640=EDGE_LOOP ( 'NONE', ( #15065, #6815 ) ) ;
#3641=VERTEX_POINT ( 'NONE', #7439 ) ;
#3642=CIRCLE ( 'NONE', #321, 1.499999999999999556 ) ;
#3643=ORIENTED_EDGE ( 'NONE', *, *, #5698, .T. ) ;
#3645=EDGE_CURVE ( 'NONE', #16215, #5645, #1157, .T. ) ;
#3646=DIRECTION ( 'NONE',  ( -0.1566598588826321192, 0.9876526153536342445, 7.798540720466730171E-17 ) ) ;
#3647=DIRECTION ( 'NONE',  ( -0.9876526153536336894, -0.1566598588826349503, 0.000000000000000000 ) ) ;
#3648=VECTOR ( 'NONE', #18073, 1000.000000000000000 ) ;
#3649=CARTESIAN_POINT ( 'NONE',  ( -68.72359699322777260, -88.85607972424168111, 1.424741226644455312E-14 ) ) ;
#3650=DIRECTION ( 'NONE',  ( -0.1566598588826321192, 0.9876526153536342445, 7.798540720466730171E-17 ) ) ;
#3653=EDGE_CURVE ( 'NONE', #10352, #4467, #15875, .T. ) ;
#3655=FACE_OUTER_BOUND ( 'NONE', #6658, .T. ) ;
#3656=FACE_BOUND ( 'NONE', #10064, .T. ) ;
#3657=DIRECTION ( 'NONE',  ( -0.1566598588826321192, 0.9876526153536342445, 7.798540720466730171E-17 ) ) ;
#3658=ORIENTED_EDGE ( 'NONE', *, *, #17731, .F. ) ;
#3659=CIRCLE ( 'NONE', #7916, 1.500000000000000888 ) ;
#3660=LINE ( 'NONE', #11048, #9401 ) ;
#3661=ORIENTED_EDGE ( 'NONE', *, *, #10209, .T. ) ;
#3664=DIRECTION ( 'NONE',  ( 0.000000000000000000, 0.000000000000000000, 1.000000000000000000 ) ) ;
#3665=VERTEX_POINT ( 'NONE', #13200 ) ;
#3666=ORIENTED_EDGE ( 'NONE', *, *, #5090, .F. ) ;
#3667=AXIS2_PLACEMENT_3D ( 'NONE', #12424, #11184, #10992 ) ;
#3668=EDGE_CURVE ( 'NONE', #18393, #730, #1744, .T. ) ;
#3670=ORIENTED_EDGE ( 'NONE', *, *, #3481, .T. ) ;
#3672=CARTESIAN_POINT ( 'NONE',  ( -34.97868976044173195, -20.73554015023333719, 21.65063509461101887 ) ) ;
#3673=CARTESIAN_POINT ( 'NONE',  ( -42.09661138885763876, -26.92708209806250608, -12.99038105676658006 ) ) ;
#3675=DIRECTION ( 'NONE',  ( 0.000000000000000000, 0.000000000000000000, 1.000000000000000000 ) ) ;
#3676=EDGE_CURVE ( 'NONE', #6916, #11814, #17610, .T. ) ;
#3678=CARTESIAN_POINT ( 'NONE',  ( -10.45209268736360997, -79.61314805016640150, -12.99038105676658539 ) ) ;
#3679=VERTEX_POINT ( 'NONE', #8863 ) ;
#3681=FACE_BOUND ( 'NONE', #6284, .T. ) ;
#3682=CIRCLE ( 'NONE', #3367, 1.500000000000001332 ) ;
#3683=DIRECTION ( 'NONE',  ( -0.1566598588826321192, 0.9876526153536342445, 7.798540720466730171E-17 ) ) ;
#3684=CARTESIAN_POINT ( 'NONE',  ( -20.16390053013728334, -18.38564226699385529, 4.330127018922218518 ) ) ;
#3685=DIRECTION ( 'NONE',  ( -0.1566598588826321192, 0.9876526153536342445, 7.798540720466730171E-17 ) ) ;
#3688=EDGE_LOOP ( 'NONE', ( #2858, #18740 ) ) ;
#3689=ORIENTED_EDGE ( 'NONE', *, *, #1480, .F. ) ;
#3691=FACE_BOUND ( 'NONE', #9396, .T. ) ;
#3692=EDGE_CURVE ( 'NONE', #11647, #1436, #5046, .T. ) ;
#3693=EDGE_CURVE ( 'NONE', #3520, #9109, #17414, .T. ) ;
#3694=EDGE_CURVE ( 'NONE', #344, #7608, #18113, .T. ) ;
#3696=EDGE_CURVE ( 'NONE', #16742, #11890, #1730, .T. ) ;
#3699=CARTESIAN_POINT ( 'NONE',  ( -80.30645961545690170, -27.92535762103354458, 92.77853496600735639 ) ) ;
#3700=FACE_BOUND ( 'NONE', #425, .T. ) ;
#3703=DIRECTION ( 'NONE',  ( -0.1566598588826321192, 0.9876526153536342445, 7.798540720466730171E-17 ) ) ;
#3704=CARTESIAN_POINT ( 'NONE',  ( -60.36818477289977380, -29.82528948739119556, 21.65063509461101887 ) ) ;
#3706=ORIENTED_EDGE ( 'NONE', *, *, #1080, .T. ) ;
#3708=EDGE_LOOP ( 'NONE', ( #2297, #18656 ) ) ;
#3709=CYLINDRICAL_SURFACE ( 'NONE', #16272, 1.500000000000001554 ) ;
#3710=ORIENTED_EDGE ( 'NONE', *, *, #16731, .T. ) ;
#3711=EDGE_LOOP ( 'NONE', ( #9095, #9230 ) ) ;
#3712=ORIENTED_EDGE ( 'NONE', *, *, #4114, .T. ) ;
#3714=CIRCLE ( 'NONE', #6170, 139.0000000000000000 ) ;
#3715=CARTESIAN_POINT ( 'NONE',  ( -47.03487446562577645, -27.71038139247565368, 21.65063509461101887 ) ) ;
#3716=EDGE_CURVE ( 'NONE', #11172, #12170, #17981, .T. ) ;
#3717=DIRECTION ( 'NONE',  ( -0.9876526153536336894, -0.1566598588826349503, 0.000000000000000000 ) ) ;
#3718=DIRECTION ( 'NONE',  ( -0.9876526153536341335, -0.1566598588826327021, 0.000000000000000000 ) ) ;
#3719=EDGE_CURVE ( 'NONE', #1188, #8364, #15093, .T. ) ;
#3720=VECTOR ( 'NONE', #13608, 1000.000000000000000 ) ;
#3721=DIRECTION ( 'NONE',  ( -0.9876526153536336894, -0.1566598588826350336, 0.000000000000000000 ) ) ;
#3722=CARTESIAN_POINT ( 'NONE',  ( -16.70711637639958269, -17.83733276090463704, 21.65063509461101532 ) ) ;
#3723=CARTESIAN_POINT ( 'NONE',  ( -23.33121169713865584, -23.95054477929251036, 8.660254037844417496 ) ) ;
#3725=ORIENTED_EDGE ( 'NONE', *, *, #6440, .F. ) ;
#3726=EDGE_LOOP ( 'NONE', ( #17084, #17441, #17181, #12468 ) ) ;
#3728=CARTESIAN_POINT ( 'NONE',  ( -58.68235252892885256, -24.49537676341649117, 17.32050807568882078 ) ) ;
#3729=ORIENTED_EDGE ( 'NONE', *, *, #10659, .F. ) ;
#3730=CARTESIAN_POINT ( 'NONE',  ( -47.81817376003892406, -22.77211831570754086, 12.99038105676661736 ) ) ;
#3731=VERTEX_POINT ( 'NONE', #18067 ) ;
#3732=EDGE_LOOP ( 'NONE', ( #18641, #6323 ) ) ;
#3733=CARTESIAN_POINT ( 'NONE',  ( -59.83472345504510770, -87.44614099429799126, 4.330127018922213189 ) ) ;
#3734=FACE_OUTER_BOUND ( 'NONE', #871, .T. ) ;
#3735=CARTESIAN_POINT ( 'NONE',  ( 1.360103686702108128, -20.03404830722672259, -17.32050807568878170 ) ) ;
#3736=DIRECTION ( 'NONE',  ( 0.000000000000000000, 0.000000000000000000, 1.000000000000000000 ) ) ;
#3737=CARTESIAN_POINT ( 'NONE',  ( -50.45202360918564466, -85.95787233491300583, -17.32050807568878525 ) ) ;
#3738=DIRECTION ( 'NONE',  ( -0.1566598588826321192, 0.9876526153536342445, 7.798540720466730171E-17 ) ) ;
#3739=( NAMED_UNIT ( * ) PLANE_ANGLE_UNIT ( ) SI_UNIT ( $, .RADIAN. ) );
#3740=ADVANCED_FACE ( 'NONE', ( #14914 ), #3428, .F. ) ;
#3742=EDGE_LOOP ( 'NONE', ( #2805, #17397 ) ) ;
#3743=DIRECTION ( 'NONE',  ( -0.1566598588826321192, 0.9876526153536342445, 7.798540720466730171E-17 ) ) ;
#3745=CYLINDRICAL_SURFACE ( 'NONE', #10609, 1.500000000000000666 ) ;
#3746=ADVANCED_FACE ( 'NONE', ( #1935 ), #7720, .F. ) ;
#3747=DIRECTION ( 'NONE',  ( -0.1566598588826321192, 0.9876526153536342445, 7.798540720466730171E-17 ) ) ;
#3749=ORIENTED_EDGE ( 'NONE', *, *, #12586, .F. ) ;
#3750=DIRECTION ( 'NONE',  ( -0.9876526153536336894, -0.1566598588826349503, 0.000000000000000000 ) ) ;
#3752=ORIENTED_EDGE ( 'NONE', *, *, #15016, .T. ) ;
#3753=EDGE_LOOP ( 'NONE', ( #2627, #3140, #11646, #8492 ) ) ;
#3754=CARTESIAN_POINT ( 'NONE',  ( 55.85952145814821534, 6.938893903907228378E-15, -24.99999999999999289 ) ) ;
#3755=ORIENTED_EDGE ( 'NONE', *, *, #4446, .T. ) ;
#3756=CARTESIAN_POINT ( 'NONE',  ( -26.58364252993588650, -19.40393134973095357, -4.330127018922180326 ) ) ;
#3759=LINE ( 'NONE', #12576, #17335 ) ;
#3760=DIRECTION ( 'NONE',  ( 0.000000000000000000, 0.000000000000000000, 1.000000000000000000 ) ) ;
#3761=DIRECTION ( 'NONE',  ( -0.1566598588826326743, -0.9876526153536341335, 0.000000000000000000 ) ) ;
#3763=ORIENTED_EDGE ( 'NONE', *, *, #2432, .F. ) ;
#3764=CARTESIAN_POINT ( 'NONE',  ( -2.057045456857756971, -78.28153924966404986, 21.65063509461100821 ) ) ;
#3765=DIRECTION ( 'NONE',  ( -0.1566598588826321192, 0.9876526153536342445, 7.798540720466730171E-17 ) ) ;
#3766=EDGE_LOOP ( 'NONE', ( #8570, #391 ) ) ;
#3767=FACE_BOUND ( 'NONE', #10947, .T. ) ;
#3768=CARTESIAN_POINT ( 'NONE',  ( -5.842937607509656850, -16.11407431319567962, 17.32050807568881012 ) ) ;
#3770=EDGE_CURVE ( 'NONE', #7505, #139, #10809, .T. ) ;
#3773=ORIENTED_EDGE ( 'NONE', *, *, #13251, .T. ) ;
#3776=ORIENTED_EDGE ( 'NONE', *, *, #11014, .F. ) ;
#3777=DIRECTION ( 'NONE',  ( -0.9876526153536336894, -0.1566598588826349503, 0.000000000000000000 ) ) ;
#3778=FACE_BOUND ( 'NONE', #15963, .T. ) ;
#3779=CARTESIAN_POINT ( 'NONE',  ( -65.26681283949008616, -88.30777021815246997, -17.32050807568878525 ) ) ;
#3780=AXIS2_PLACEMENT_3D ( 'NONE', #16211, #3203, #13526 ) ;
#3781=DIRECTION ( 'NONE',  ( -0.9876526153536336894, -0.1566598588826349503, 0.000000000000000000 ) ) ;
#3783=ORIENTED_EDGE ( 'NONE', *, *, #1166, .T. ) ;
#3784=AXIS2_PLACEMENT_3D ( 'NONE', #17823, #14857, #657 ) ;
#3785=CARTESIAN_POINT ( 'NONE',  ( -69.25705831108246002, -31.23522821733487476, -17.32050807568878170 ) ) ;
#3786=DIRECTION ( 'NONE',  ( -0.9876526153536341335, -0.1566598588826327021, 0.000000000000000000 ) ) ;
#3788=EDGE_LOOP ( 'NONE', ( #12762, #5999, #4570, #11309 ) ) ;
#3789=DIRECTION ( 'NONE',  ( -0.9876526153536336894, -0.1566598588826349503, 0.000000000000000000 ) ) ;
#3790=ADVANCED_FACE ( 'NONE', ( #11555 ), #3207, .F. ) ;
#3791=CARTESIAN_POINT ( 'NONE',  ( -38.92930022185625205, -21.36217958576384746, -8.660254037844380193 ) ) ;
#3792=EDGE_CURVE ( 'NONE', #18229, #1028, #7333, .T. ) ;
#3793=DIRECTION ( 'NONE',  ( -0.1566598588826321192, 0.9876526153536342445, 7.798540720466730171E-17 ) ) ;
#3794=VERTEX_POINT ( 'NONE', #2179 ) ;
#3795=VERTEX_POINT ( 'NONE', #18247 ) ;
#3796=FACE_OUTER_BOUND ( 'NONE', #15562, .T. ) ;
#3797=ORIENTED_EDGE ( 'NONE', *, *, #8887, .F. ) ;
#3798=CARTESIAN_POINT ( 'NONE',  ( -38.92930022185625205, -21.36217958576385456, 8.660254037844417496 ) ) ;
#3800=FACE_BOUND ( 'NONE', #12522, .T. ) ;
#3801=CARTESIAN_POINT ( 'NONE',  ( -19.34096622554629263, -81.02308678011010556, 17.32050807568881368 ) ) ;
#3802=LINE ( 'NONE', #18377, #7555 ) ;
#3804=AXIS2_PLACEMENT_3D ( 'NONE', #14685, #1704, #13247 ) ;
#3805=CARTESIAN_POINT ( 'NONE',  ( -47.98289207080156871, -85.56622268770642847, -4.330127018922185655 ) ) ;
#3806=LINE ( 'NONE', #12455, #3815 ) ;
#3807=ORIENTED_EDGE ( 'NONE', *, *, #2766, .F. ) ;
#3808=CARTESIAN_POINT ( 'NONE',  ( -23.33121169713865584, -23.95054477929251036, -8.660254037844380193 ) ) ;
#3810=ADVANCED_FACE ( 'NONE', ( #5219 ), #1901, .F. ) ;
#3811=EDGE_LOOP ( 'NONE', ( #6923, #2569, #17630, #1572 ) ) ;
#3814=CARTESIAN_POINT ( 'NONE',  ( -28.26947477390680774, -24.73384407370567217, -17.32050807568878170 ) ) ;
#3815=VECTOR ( 'NONE', #12623, 1000.000000000000000 ) ;
#3816=ORIENTED_EDGE ( 'NONE', *, *, #4057, .F. ) ;
#3817=CIRCLE ( 'NONE', #16884, 1.499999999999999556 ) ;
#3818=EDGE_CURVE ( 'NONE', #13180, #3665, #10582, .T. ) ;
#3819=CIRCLE ( 'NONE', #18435, 1.500000000000000888 ) ;
#3820=ORIENTED_EDGE ( 'NONE', *, *, #3504, .T. ) ;
#3821=DIRECTION ( 'NONE',  ( -0.1566598588826321192, 0.9876526153536342445, 7.798540720466730171E-17 ) ) ;
#3822=EDGE_CURVE ( 'NONE', #9967, #1267, #5463, .T. ) ;
#3823=CIRCLE ( 'NONE', #13813, 1.500000000000000888 ) ;
#3824=DIRECTION ( 'NONE',  ( -0.1566598588826321747, 0.9876526153536343555, 0.000000000000000000 ) ) ;
#3825=DIRECTION ( 'NONE',  ( -0.1566598588826321747, 0.9876526153536343555, 0.000000000000000000 ) ) ;
#3826=ORIENTED_EDGE ( 'NONE', *, *, #15472, .T. ) ;
#3827=DIRECTION ( 'NONE',  ( 0.000000000000000000, 0.000000000000000000, 1.000000000000000000 ) ) ;
#3828=DIRECTION ( 'NONE',  ( -0.1566598588826321747, 0.9876526153536343555, 0.000000000000000000 ) ) ;
#3829=AXIS2_PLACEMENT_3D ( 'NONE', #12912, #5839, #4306 ) ;
#3831=CARTESIAN_POINT ( 'NONE',  ( -49.79347899074618056, -23.08543803347280132, -4.330127018922180326 ) ) ;
#3832=PRESENTATION_STYLE_ASSIGNMENT (( #16865 ) ) ;
#3834=ORIENTED_EDGE ( 'NONE', *, *, #8638, .F. ) ;
#3835=CARTESIAN_POINT ( 'NONE',  ( -22.34355908178503114, -23.79388492040988012, -12.99038105676658006 ) ) ;
#3836=AXIS2_PLACEMENT_3D ( 'NONE', #17698, #13386, #12037 ) ;
#3837=CARTESIAN_POINT ( 'NONE',  ( -27.73601345605213098, -82.35469558061247142, -8.660254037844385522 ) ) ;
#3840=CARTESIAN_POINT ( 'NONE',  ( -73.49714175923330117, -26.84527464665595176, -17.32050807568878170 ) ) ;
#3841=LINE ( 'NONE', #9655, #2706 ) ;
#3844=ORIENTED_EDGE ( 'NONE', *, *, #6220, .F. ) ;
#3849=VERTEX_POINT ( 'NONE', #14879 ) ;
#3850=EDGE_CURVE ( 'NONE', #12551, #2681, #2721, .T. ) ;
#3851=LINE ( 'NONE', #15156, #12443 ) ;
#3852=EDGE_CURVE ( 'NONE', #12162, #1839, #928, .T. ) ;
#3853=CIRCLE ( 'NONE', #5998, 1.500000000000000888 ) ;
#3854=DIRECTION ( 'NONE',  ( -0.1566598588826321192, 0.9876526153536342445, 7.798540720466731404E-17 ) ) ;
#3855=DIRECTION ( 'NONE',  ( -0.1566598588826321192, 0.9876526153536342445, 7.798540720466731404E-17 ) ) ;
#3856=DIRECTION ( 'NONE',  ( -0.1566598588826321192, 0.9876526153536342445, 7.798540720466730171E-17 ) ) ;
#3857=CIRCLE ( 'NONE', #8432, 1.500000000000000888 ) ;
#3858=CYLINDRICAL_SURFACE ( 'NONE', #16978, 1.500000000000000666 ) ;
#3859=CARTESIAN_POINT ( 'NONE',  ( -19.34096622554629263, -81.02308678011010556, 8.660254037844412167 ) ) ;
#3860=CARTESIAN_POINT ( 'NONE',  ( -5.513829610595458064, -78.82984875575324679, -21.65063509461098690 ) ) ;
#3862=CARTESIAN_POINT ( 'NONE',  ( -6.995308533625909320, -79.06483854407720457, -12.99038105676658539 ) ) ;
#3863=DIRECTION ( 'NONE',  ( -0.1566598588826321747, 0.9876526153536343555, 0.000000000000000000 ) ) ;
#3864=VERTEX_POINT ( 'NONE', #3393 ) ;
#3865=CARTESIAN_POINT ( 'NONE',  ( -28.26947477390680774, -24.73384407370567217, 1.869203119972154228E-14 ) ) ;
#3866=EDGE_LOOP ( 'NONE', ( #8102, #11142 ) ) ;
#3867=LINE ( 'NONE', #8060, #10761 ) ;
#3869=AXIS2_PLACEMENT_3D ( 'NONE', #6572, #9503, #16820 ) ;
#3870=FACE_BOUND ( 'NONE', #1085, .T. ) ;
#3873=AXIS2_PLACEMENT_3D ( 'NONE', #8173, #994, #6765 ) ;
#3875=CARTESIAN_POINT ( 'NONE',  ( -25.76070822534488869, -82.04137586284721806, 8.660254037844412167 ) ) ;
#3876=EDGE_CURVE ( 'NONE', #12785, #12633, #6616, .T. ) ;
#3877=AXIS2_PLACEMENT_3D ( 'NONE', #11321, #11240, #9546 ) ;
#3882=DIRECTION ( 'NONE',  ( -0.1566598588826321192, 0.9876526153536342445, 7.798540720466731404E-17 ) ) ;
#3883=LINE ( 'NONE', #17104, #1489 ) ;
#3884=DIRECTION ( 'NONE',  ( 0.000000000000000000, 0.000000000000000000, 1.000000000000000000 ) ) ;
#3885=ORIENTED_EDGE ( 'NONE', *, *, #2261, .T. ) ;
#3886=DIRECTION ( 'NONE',  ( -0.9876526153536341335, -0.1566598588826327021, 0.000000000000000000 ) ) ;
#3888=ORIENTED_EDGE ( 'NONE', *, *, #1904, .F. ) ;
#3889=ORIENTED_EDGE ( 'NONE', *, *, #6388, .T. ) ;
#3890=DIRECTION ( 'NONE',  ( -0.1566598588826321192, 0.9876526153536342445, 7.798540720466730171E-17 ) ) ;
#3894=VERTEX_POINT ( 'NONE', #2440 ) ;
#3895=EDGE_CURVE ( 'NONE', #16215, #2189, #939, .T. ) ;
#3896=CIRCLE ( 'NONE', #12685, 1.500000000000000000 ) ;
#3897=AXIS2_PLACEMENT_3D ( 'NONE', #5898, #17199, #14618 ) ;
#3898=FACE_OUTER_BOUND ( 'NONE', #9715, .T. ) ;
#3899=EDGE_CURVE ( 'NONE', #1264, #10247, #15441, .T. ) ;
#3902=EDGE_CURVE ( 'NONE', #7759, #139, #10286, .T. ) ;
#3903=DIRECTION ( 'NONE',  ( -0.1566598588826321192, 0.9876526153536342445, 7.798540720466731404E-17 ) ) ;
#3904=VECTOR ( 'NONE', #856, 1000.000000000000000 ) ;
#3905=CYLINDRICAL_SURFACE ( 'NONE', #10272, 1.500000000000000888 ) ;
#3906=CIRCLE ( 'NONE', #6372, 1.500000000000000888 ) ;
#3907=DIRECTION ( 'NONE',  ( 0.000000000000000000, 0.000000000000000000, 1.000000000000000000 ) ) ;
#3908=VERTEX_POINT ( 'NONE', #15801 ) ;
#3909=DIRECTION ( 'NONE',  ( -0.1566598588826321747, 0.9876526153536343555, 0.000000000000000000 ) ) ;
#3910=DIRECTION ( 'NONE',  ( -0.1566598588826321192, 0.9876526153536342445, 7.798540720466730171E-17 ) ) ;
#3911=AXIS2_PLACEMENT_3D ( 'NONE', #16364, #12158, #3354 ) ;
#3914=FACE_BOUND ( 'NONE', #14625, .T. ) ;
#3915=CARTESIAN_POINT ( 'NONE',  ( -2.096680467035594297, -20.58235781331593017, -17.32050807568878170 ) ) ;
#3916=ORIENTED_EDGE ( 'NONE', *, *, #8270, .F. ) ;
#3917=VERTEX_POINT ( 'NONE', #12927 ) ;
#3918=DIRECTION ( 'NONE',  ( -0.1566598588826321747, 0.9876526153536343555, 0.000000000000000000 ) ) ;
#3920=ORIENTED_EDGE ( 'NONE', *, *, #12842, .T. ) ;
#3921=DIRECTION ( 'NONE',  ( 0.000000000000000000, 0.000000000000000000, 1.000000000000000000 ) ) ;
#3922=AXIS2_PLACEMENT_3D ( 'NONE', #7381, #10297, #13135 ) ;
#3923=EDGE_CURVE ( 'NONE', #14148, #17176, #6071, .T. ) ;
#3924=CIRCLE ( 'NONE', #11192, 1.500000000000000888 ) ;
#3925=DIRECTION ( 'NONE',  ( 0.000000000000000000, 0.000000000000000000, 1.000000000000000000 ) ) ;
#3926=EDGE_CURVE ( 'NONE', #10692, #9818, #15739, .T. ) ;
#3927=VERTEX_POINT ( 'NONE', #3931 ) ;
#3928=AXIS2_PLACEMENT_3D ( 'NONE', #18459, #13840, #16618 ) ;
#3929=EDGE_CURVE ( 'NONE', #7929, #6801, #5095, .T. ) ;
#3931=CARTESIAN_POINT ( 'NONE',  ( -70.04035760549561473, -26.29696514056674772, 1.908195823574487804E-14 ) ) ;
#3932=ADVANCED_FACE ( 'NONE', ( #14665 ), #3173, .F. ) ;
#3934=CIRCLE ( 'NONE', #16992, 1.500000000000000444 ) ;
#3935=DIRECTION ( 'NONE',  ( -0.1566598588826321192, 0.9876526153536342445, 7.798540720466730171E-17 ) ) ;
#3937=FACE_OUTER_BOUND ( 'NONE', #2169, .T. ) ;
#3938=ORIENTED_EDGE ( 'NONE', *, *, #1214, .T. ) ;
#3939=CARTESIAN_POINT ( 'NONE',  ( -65.26681283949008616, -88.30777021815248418, 17.32050807568881368 ) ) ;
#3940=AXIS2_PLACEMENT_3D ( 'NONE', #11869, #5850, #7643 ) ;
#3941=CYLINDRICAL_SURFACE ( 'NONE', #7791, 1.500000000000001554 ) ;
#3942=CARTESIAN_POINT ( 'NONE',  ( -11.93357161039406300, -79.84813783849037350, 4.330127018922213189 ) ) ;
#3943=CARTESIAN_POINT ( 'NONE',  ( -34.97868976044173195, -20.73554015023332298, -12.99038105676658006 ) ) ;
#3944=ORIENTED_EDGE ( 'NONE', *, *, #1956, .F. ) ;
#3945=CARTESIAN_POINT ( 'NONE',  ( -21.81009776393036503, -81.41473642731669713, 21.65063509461101532 ) ) ;
#3948=AXIS2_PLACEMENT_3D ( 'NONE', #18597, #15587, #9741 ) ;
#3949=DIRECTION ( 'NONE',  ( 0.000000000000000000, 0.000000000000000000, 1.000000000000000000 ) ) ;
#3950=DIRECTION ( 'NONE',  ( -0.9876526153536336894, -0.1566598588826349503, 0.000000000000000000 ) ) ;
#3951=ADVANCED_FACE ( 'NONE', ( #6149 ), #831, .F. ) ;
#3952=ORIENTED_EDGE ( 'NONE', *, *, #10858, .T. ) ;
#3953=AXIS2_PLACEMENT_3D ( 'NONE', #14667, #17923, #6341 ) ;
#3954=LINE ( 'NONE', #9767, #17994 ) ;
#3955=DIRECTION ( 'NONE',  ( -0.9876526153536341335, -0.1566598588826327021, 0.000000000000000000 ) ) ;
#3957=DIRECTION ( 'NONE',  ( -0.9876526153536336894, -0.1566598588826350336, 0.000000000000000000 ) ) ;
#3958=AXIS2_PLACEMENT_3D ( 'NONE', #6974, #13097, #15766 ) ;
#3960=EDGE_LOOP ( 'NONE', ( #2107, #7180 ) ) ;
#3961=FACE_OUTER_BOUND ( 'NONE', #10938, .T. ) ;
#3962=EDGE_CURVE ( 'NONE', #5781, #10329, #4541, .T. ) ;
#3964=ADVANCED_FACE ( 'NONE', ( #8143 ), #5303, .F. ) ;
#3965=FACE_OUTER_BOUND ( 'NONE', #11098, .T. ) ;
#3967=AXIS2_PLACEMENT_3D ( 'NONE', #1146, #9926, #1335 ) ;
#3968=AXIS2_PLACEMENT_3D ( 'NONE', #3418, #2106, #7894 ) ;
#3969=ORIENTED_EDGE ( 'NONE', *, *, #5996, .F. ) ;
#3970=CARTESIAN_POINT ( 'NONE',  ( -48.02252708097939404, -27.86704125135830523, 8.660254037844417496 ) ) ;
#3971=VERTEX_POINT ( 'NONE', #12287 ) ;
#3972=ORIENTED_EDGE ( 'NONE', *, *, #16312, .F. ) ;
#3974=CIRCLE ( 'NONE', #13966, 1.499999999999999556 ) ;
#3977=FACE_BOUND ( 'NONE', #18521, .T. ) ;
#3978=DIRECTION ( 'NONE',  ( -0.1566598588826321192, 0.9876526153536342445, 7.798540720466730171E-17 ) ) ;
#3979=CIRCLE ( 'NONE', #10651, 1.500000000000000888 ) ;
#3980=CARTESIAN_POINT ( 'NONE',  ( -25.10216360690543524, -19.16894156140701000, -4.330127018922180326 ) ) ;
#3981=EDGE_CURVE ( 'NONE', #1864, #9740, #5131, .T. ) ;
#3982=AXIS2_PLACEMENT_3D ( 'NONE', #7370, #7185, #6027 ) ;
#3983=CARTESIAN_POINT ( 'NONE',  ( -66.08974714408108753, -25.67032570503621258, -21.65063509461097979 ) ) ;
#3984=DIRECTION ( 'NONE',  ( -0.1566598588826321192, 0.9876526153536342445, 7.798540720466730171E-17 ) ) ;
#3985=DIRECTION ( 'NONE',  ( -0.9876526153536341335, -0.1566598588826327021, 0.000000000000000000 ) ) ;
#3989=VERTEX_POINT ( 'NONE', #10835 ) ;
#3990=ORIENTED_EDGE ( 'NONE', *, *, #7662, .T. ) ;
#3992=DIRECTION ( 'NONE',  ( -0.9876526153536341335, -0.1566598588826327021, 0.000000000000000000 ) ) ;
#3994=ORIENTED_EDGE ( 'NONE', *, *, #17207, .T. ) ;
#3996=ORIENTED_EDGE ( 'NONE', *, *, #9746, .T. ) ;
#3998=EDGE_CURVE ( 'NONE', #18092, #13174, #12065, .T. ) ;
#3999=DIRECTION ( 'NONE',  ( -0.9876526153536341335, -0.1566598588826327021, 0.000000000000000000 ) ) ;
#4000=ORIENTED_EDGE ( 'NONE', *, *, #8473, .T. ) ;
#4002=DIRECTION ( 'NONE',  ( -0.1566598588826321192, 0.9876526153536342445, 7.798540720466730171E-17 ) ) ;
#4004=CYLINDRICAL_SURFACE ( 'NONE', #6049, 1.500000000000001554 ) ;
#4005=CARTESIAN_POINT ( 'NONE',  ( -75.96627329761737712, -27.23692429386254688, 21.65063509461102242 ) ) ;
#4006=DIRECTION ( 'NONE',  ( -0.1566598588826321192, 0.9876526153536342445, 7.798540720466731404E-17 ) ) ;
#4007=CARTESIAN_POINT ( 'NONE',  ( -46.54104815794895700, -27.63205146303435100, 1.887572821959364500E-14 ) ) ;
#4008=ORIENTED_EDGE ( 'NONE', *, *, #145, .T. ) ;
#4009=ORIENTED_EDGE ( 'NONE', *, *, #484, .F. ) ;
#4010=CIRCLE ( 'NONE', #10373, 1.500000000000000000 ) ;
#4011=FACE_BOUND ( 'NONE', #7147, .T. ) ;
#4012=CARTESIAN_POINT ( 'NONE',  ( -65.26681283949008616, -88.30777021815246997, -8.660254037844385522 ) ) ;
#4014=ORIENTED_EDGE ( 'NONE', *, *, #7861, .F. ) ;
#4015=ORIENTED_EDGE ( 'NONE', *, *, #2195, .F. ) ;
#4016=DIRECTION ( 'NONE',  ( -0.1566598588826321192, 0.9876526153536342445, 7.798540720466730171E-17 ) ) ;
#4017=ORIENTED_EDGE ( 'NONE', *, *, #13225, .F. ) ;
#4018=CARTESIAN_POINT ( 'NONE',  ( 8.807133312032172867, -76.55828080195509244, 8.660254037844406838 ) ) ;
#4019=EDGE_CURVE ( 'NONE', #2560, #14180, #12740, .T. ) ;
#4020=DIRECTION ( 'NONE',  ( 0.000000000000000000, 0.000000000000000000, 1.000000000000000000 ) ) ;
#4021=ORIENTED_EDGE ( 'NONE', *, *, #13424, .T. ) ;
#4022=DIRECTION ( 'NONE',  ( -0.9876526153536341335, -0.1566598588826327021, 0.000000000000000000 ) ) ;
#4025=LINE ( 'NONE', #9826, #13983 ) ;
#4026=DIRECTION ( 'NONE',  ( -0.1566598588826321192, 0.9876526153536342445, 7.798540720466730171E-17 ) ) ;
#4028=EDGE_CURVE ( 'NONE', #3313, #17816, #1741, .T. ) ;
#4030=CARTESIAN_POINT ( 'NONE',  ( -23.33121169713865584, -23.95054477929251036, 8.660254037844417496 ) ) ;
#4032=ORIENTED_EDGE ( 'NONE', *, *, #6709, .F. ) ;
#4033=EDGE_LOOP ( 'NONE', ( #13267, #3342 ) ) ;
#4035=FACE_OUTER_BOUND ( 'NONE', #1789, .T. ) ;
#4037=EDGE_LOOP ( 'NONE', ( #17040, #8717, #14369, #33 ) ) ;
#4041=VERTEX_POINT ( 'NONE', #5030 ) ;
#4043=VERTEX_POINT ( 'NONE', #8076 ) ;
#4044=LINE ( 'NONE', #11339, #8531 ) ;
#4046=CARTESIAN_POINT ( 'NONE',  ( -23.12685837619818940, -18.85562184364174598, 4.330127018922218518 ) ) ;
#4047=CARTESIAN_POINT ( 'NONE',  ( -20.86208015875457988, -23.55889513208593655, -21.65063509461098334 ) ) ;
#4049=CYLINDRICAL_SURFACE ( 'NONE', #9045, 1.500000000000001554 ) ;
#4051=FACE_BOUND ( 'NONE', #12098, .T. ) ;
#4053=VECTOR ( 'NONE', #14886, 1000.000000000000000 ) ;
#4054=LINE ( 'NONE', #6840, #16648 ) ;
#4055=EDGE_LOOP ( 'NONE', ( #6042, #10786 ) ) ;
#4056=ADVANCED_FACE ( 'NONE', ( #18276 ), #10999, .F. ) ;
#4057=EDGE_CURVE ( 'NONE', #14743, #12954, #8778, .T. ) ;
#4058=VERTEX_POINT ( 'NONE', #2388 ) ;
#4059=CYLINDRICAL_SURFACE ( 'NONE', #9053, 1.500000000000001554 ) ;
#4060=ORIENTED_EDGE ( 'NONE', *, *, #3528, .T. ) ;
#4061=ORIENTED_EDGE ( 'NONE', *, *, #16832, .T. ) ;
#4062=LINE ( 'NONE', #15548, #12899 ) ;
#4063=EDGE_CURVE ( 'NONE', #6818, #13999, #4246, .T. ) ;
#4064=EDGE_CURVE ( 'NONE', #14647, #14006, #7892, .T. ) ;
#4065=FACE_BOUND ( 'NONE', #4543, .T. ) ;
#4066=ADVANCED_FACE ( 'NONE', ( #16879 ), #5206, .F. ) ;
#4068=ORIENTED_EDGE ( 'NONE', *, *, #12819, .T. ) ;
#4069=DIRECTION ( 'NONE',  ( -0.9876526153536336894, -0.1566598588826349503, 0.000000000000000000 ) ) ;
#4070=FACE_OUTER_BOUND ( 'NONE', #11082, .T. ) ;
#4071=EDGE_LOOP ( 'NONE', ( #7725, #18637, #16808, #10084 ) ) ;
#4072=VERTEX_POINT ( 'NONE', #13625 ) ;
#4074=DIRECTION ( 'NONE',  ( -0.1566598588826321192, 0.9876526153536342445, 7.798540720466731404E-17 ) ) ;
#4075=FACE_OUTER_BOUND ( 'NONE', #11055, .T. ) ;
#4076=DIRECTION ( 'NONE',  ( -0.000000000000000000, -0.000000000000000000, -1.000000000000000000 ) ) ;
#4077=AXIS2_PLACEMENT_3D ( 'NONE', #5553, #2600, #8384 ) ;
#4079=ORIENTED_EDGE ( 'NONE', *, *, #15226, .F. ) ;
#4082=VERTEX_POINT ( 'NONE', #12281 ) ;
#4083=ORIENTED_EDGE ( 'NONE', *, *, #11826, .T. ) ;
#4084=FACE_BOUND ( 'NONE', #5231, .T. ) ;
#4085=ADVANCED_FACE ( 'NONE', ( #6453 ), #18233, .F. ) ;
#4086=CARTESIAN_POINT ( 'NONE',  ( -57.69469991357524208, -24.33871690453385028, -4.330127018922180326 ) ) ;
#4087=EDGE_CURVE ( 'NONE', #4380, #12710, #2739, .T. ) ;
#4090=CARTESIAN_POINT ( 'NONE',  ( -43.04462899403340970, -84.78292339329327376, 4.330127018922213189 ) ) ;
#4092=EDGE_CURVE ( 'NONE', #18200, #6686, #11794, .T. ) ;
#4093=CIRCLE ( 'NONE', #5625, 1.500000000000000888 ) ;
#4094=DIRECTION ( 'NONE',  ( -0.9876526153536336894, -0.1566598588826349503, 0.000000000000000000 ) ) ;
#4098=ORIENTED_EDGE ( 'NONE', *, *, #3716, .T. ) ;
#4099=CARTESIAN_POINT ( 'NONE',  ( 7.819480696678551723, -76.71494066083772623, -12.99038105676658894 ) ) ;
#4100=CARTESIAN_POINT ( 'NONE',  ( -46.33669483700847280, -22.53712852738359729, 21.65063509461102242 ) ) ;
#4101=VERTEX_POINT ( 'NONE', #7738 ) ;
#4102=VERTEX_POINT ( 'NONE', #9634 ) ;
#4103=FACE_BOUND ( 'NONE', #17791, .T. ) ;
#4105=CIRCLE ( 'NONE', #5933, 1.500000000000000444 ) ;
#4107=VECTOR ( 'NONE', #14588, 1000.000000000000000 ) ;
#4108=EDGE_LOOP ( 'NONE', ( #17122, #7204 ) ) ;
#4109=FACE_OUTER_BOUND ( 'NONE', #15467, .T. ) ;
#4110=CARTESIAN_POINT ( 'NONE',  ( -4.361458684479201153, -15.87908452487173427, 1.561251128379126385E-14 ) ) ;
#4112=DIRECTION ( 'NONE',  ( -0.9876526153536336894, -0.1566598588826349503, 0.000000000000000000 ) ) ;
#4114=EDGE_CURVE ( 'NONE', #5804, #7971, #7933, .T. ) ;
#4115=CARTESIAN_POINT ( 'NONE',  ( -53.90880776292333820, -86.50618184100221697, 1.424741226644455312E-14 ) ) ;
#4116=FACE_OUTER_BOUND ( 'NONE', #5413, .T. ) ;
#4117=LINE ( 'NONE', #5286, #14508 ) ;
#4118=ORIENTED_EDGE ( 'NONE', *, *, #1350, .F. ) ;
#4119=DIRECTION ( 'NONE',  ( -0.1566598588826321192, 0.9876526153536342445, 7.798540720466730171E-17 ) ) ;
#4120=ORIENTED_EDGE ( 'NONE', *, *, #12728, .T. ) ;
#4121=ADVANCED_FACE ( 'NONE', ( #16952 ), #6603, .F. ) ;
#4122=CARTESIAN_POINT ( 'NONE',  ( -15.92381708198643153, -22.77559583767277473, 4.330127018922217630 ) ) ;
#4123=CARTESIAN_POINT ( 'NONE',  ( -38.10636591726525069, -83.99962409888011905, 4.330127018922213189 ) ) ;
#4125=ORIENTED_EDGE ( 'NONE', *, *, #16207, .F. ) ;
#4127=EDGE_CURVE ( 'NONE', #10862, #9895, #1035, .T. ) ;
#4129=CARTESIAN_POINT ( 'NONE',  ( -68.55887868246516348, -26.06197535224280770, 17.32050807568882078 ) ) ;
#4130=VERTEX_POINT ( 'NONE', #8110 ) ;
#4133=CYLINDRICAL_SURFACE ( 'NONE', #15433, 1.500000000000001554 ) ;
#4134=CARTESIAN_POINT ( 'NONE',  ( -56.91140061916208737, -29.27697998130198442, -12.99038105676658006 ) ) ;
#4137=EDGE_CURVE ( 'NONE', #8368, #10816, #7300, .T. ) ;
#4142=VERTEX_POINT ( 'NONE', #644 ) ;
#4143=FACE_OUTER_BOUND ( 'NONE', #12077, .T. ) ;
#4145=AXIS2_PLACEMENT_3D ( 'NONE', #4804, #13793, #4901 ) ;
#4146=ADVANCED_FACE ( 'NONE', ( #15026 ), #2426, .F. ) ;
#4147=ADVANCED_FACE ( 'NONE', ( #18091 ), #734, .F. ) ;
#4148=CARTESIAN_POINT ( 'NONE',  ( -15.92381708198643153, -22.77559583767277473, -4.330127018922181215 ) ) ;
#4150=EDGE_CURVE ( 'NONE', #6385, #11472, #7585, .T. ) ;
#4151=FACE_OUTER_BOUND ( 'NONE', #13087, .T. ) ;
#4155=VERTEX_POINT ( 'NONE', #16766 ) ;
#4156=AXIS2_PLACEMENT_3D ( 'NONE', #5650, #11404, #13201 ) ;
#4157=ORIENTED_EDGE ( 'NONE', *, *, #16208, .T. ) ;
#4158=CARTESIAN_POINT ( 'NONE',  ( -32.22008523532134205, -25.36048350923618955, 12.99038105676661736 ) ) ;
#4159=ORIENTED_EDGE ( 'NONE', *, *, #8007, .T. ) ;
#4160=VERTEX_POINT ( 'NONE', #3730 ) ;
#4161=VERTEX_POINT ( 'NONE', #8595 ) ;
#4162=ORIENTED_EDGE ( 'NONE', *, *, #5404, .T. ) ;
#4163=DIRECTION ( 'NONE',  ( 0.000000000000000000, 0.000000000000000000, 1.000000000000000000 ) ) ;
#4164=VECTOR ( 'NONE', #460, 1000.000000000000000 ) ;
#4165=DIRECTION ( 'NONE',  ( 1.000000000000000000, 0.000000000000000000, 0.000000000000000000 ) ) ;
#4166=CIRCLE ( 'NONE', #1798, 1.499999999999999556 ) ;
#4169=ORIENTED_EDGE ( 'NONE', *, *, #11281, .T. ) ;
#4172=CIRCLE ( 'NONE', #12624, 1.500000000000000444 ) ;
#4174=CARTESIAN_POINT ( 'NONE',  ( -19.17624791478365864, -18.22898240811121795, 8.660254037844417496 ) ) ;
#4175=EDGE_LOOP ( 'NONE', ( #5383, #13978 ) ) ;
#4176=ORIENTED_EDGE ( 'NONE', *, *, #5589, .F. ) ;
#4177=ORIENTED_EDGE ( 'NONE', *, *, #5915, .T. ) ;
#4178=DIRECTION ( 'NONE',  ( -0.1566598588826321747, 0.9876526153536343555, 0.000000000000000000 ) ) ;
#4179=DIRECTION ( 'NONE',  ( -0.1566598588826321192, 0.9876526153536342445, 7.798540720466730171E-17 ) ) ;
#4180=AXIS2_PLACEMENT_3D ( 'NONE', #5843, #6998, #8759 ) ;
#4181=CARTESIAN_POINT ( 'NONE',  ( -17.69476899175320739, -17.99399261978727438, 8.660254037844417496 ) ) ;
#4182=CIRCLE ( 'NONE', #5079, 20.00000000000001066 ) ;
#4184=AXIS2_PLACEMENT_3D ( 'NONE', #3234, #12226, #2203 ) ;
#4185=ORIENTED_EDGE ( 'NONE', *, *, #6942, .T. ) ;
#4187=ORIENTED_EDGE ( 'NONE', *, *, #15526, .T. ) ;
#4188=ORIENTED_EDGE ( 'NONE', *, *, #1246, .T. ) ;
#4189=DIRECTION ( 'NONE',  ( 1.000000000000000000, 0.000000000000000000, 0.000000000000000000 ) ) ;
#4190=ORIENTED_EDGE ( 'NONE', *, *, #13028, .T. ) ;
#4191=DIRECTION ( 'NONE',  ( -0.1566598588826321192, 0.9876526153536342445, 7.798540720466730171E-17 ) ) ;
#4192=AXIS2_PLACEMENT_3D ( 'NONE', #7334, #2666, #7140 ) ;
#4193=DIRECTION ( 'NONE',  ( -0.000000000000000000, -0.000000000000000000, -1.000000000000000000 ) ) ;
#4194=DIRECTION ( 'NONE',  ( -0.1566598588826321192, 0.9876526153536342445, 7.798540720466730171E-17 ) ) ;
#4195=AXIS2_PLACEMENT_3D ( 'NONE', #4148, #2646, #6937 ) ;
#4196=AXIS2_PLACEMENT_3D ( 'NONE', #1638, #15934, #8565 ) ;
#4197=LINE ( 'NONE', #17214, #15685 ) ;
#4198=CARTESIAN_POINT ( 'NONE',  ( -58.68235252892886678, -24.49537676341648407, 1.908195823574487804E-14 ) ) ;
#4200=FACE_OUTER_BOUND ( 'NONE', #13986, .T. ) ;
#4201=ORIENTED_EDGE ( 'NONE', *, *, #1480, .T. ) ;
#4202=LINE ( 'NONE', #2798, #18071 ) ;
#4203=CARTESIAN_POINT ( 'NONE',  ( -33.00338452973448966, -20.42222043246805896, -4.330127018922180326 ) ) ;
#4204=ADVANCED_FACE ( 'NONE', ( #10090 ), #8393, .F. ) ;
#4206=ORIENTED_EDGE ( 'NONE', *, *, #8271, .F. ) ;
#4208=VERTEX_POINT ( 'NONE', #17231 ) ;
#4211=DIRECTION ( 'NONE',  ( -0.1566598588826321192, 0.9876526153536342445, 7.798540720466731404E-17 ) ) ;
#4212=AXIS2_PLACEMENT_3D ( 'NONE', #17989, #10371, #8951 ) ;
#4213=CIRCLE ( 'NONE', #1799, 1.500000000000000888 ) ;
#4214=CIRCLE ( 'NONE', #16332, 1.499999999999999556 ) ;
#4217=CARTESIAN_POINT ( 'NONE',  ( -25.26688191766807279, -81.96304593340587985, -21.65063509461098690 ) ) ;
#4218=CIRCLE ( 'NONE', #287, 1.500000000000000888 ) ;
#4220=VECTOR ( 'NONE', #15086, 1000.000000000000000 ) ;
#4221=DIRECTION ( 'NONE',  ( -0.9876526153536341335, -0.1566598588826327021, 0.000000000000000000 ) ) ;
#4222=CARTESIAN_POINT ( 'NONE',  ( -69.25705831108246002, -31.23522821733487476, -8.660254037844380193 ) ) ;
#4224=EDGE_LOOP ( 'NONE', ( #3666, #13144 ) ) ;
#4225=CIRCLE ( 'NONE', #9701, 1.500000000000001332 ) ;
#4227=CARTESIAN_POINT ( 'NONE',  ( -59.83472345504510770, -87.44614099429797704, -21.65063509461098690 ) ) ;
#4229=LINE ( 'NONE', #8779, #12300 ) ;
#4230=CARTESIAN_POINT ( 'NONE',  ( -55.42992169613163611, -29.04199019297804085, -21.65063509461098334 ) ) ;
#4232=ORIENTED_EDGE ( 'NONE', *, *, #15098, .F. ) ;
#4233=VERTEX_POINT ( 'NONE', #17332 ) ;
#4234=DIRECTION ( 'NONE',  ( -0.1566598588826321747, 0.9876526153536343555, 0.000000000000000000 ) ) ;
#4236=DIRECTION ( 'NONE',  ( -0.1566598588826321192, 0.9876526153536342445, 7.798540720466731404E-17 ) ) ;
#4239=ORIENTED_EDGE ( 'NONE', *, *, #10939, .F. ) ;
#4240=EDGE_LOOP ( 'NONE', ( #13373, #1217 ) ) ;
#4241=EDGE_CURVE ( 'NONE', #14450, #7294, #18538, .T. ) ;
#4242=CARTESIAN_POINT ( 'NONE',  ( -17.40529600501688279, -23.01058562599671831, 12.99038105676661381 ) ) ;
#4244=ORIENTED_EDGE ( 'NONE', *, *, #13023, .F. ) ;
#4245=VECTOR ( 'NONE', #14138, 1000.000000000000000 ) ;
#4246=CIRCLE ( 'NONE', #8508, 1.500000000000000888 ) ;
#4247=DIRECTION ( 'NONE',  ( -0.1566598588826321192, 0.9876526153536342445, 7.798540720466730171E-17 ) ) ;
#4248=ADVANCED_FACE ( 'NONE', ( #1308 ), #14457, .F. ) ;
#4249=DIRECTION ( 'NONE',  ( 0.000000000000000000, 0.000000000000000000, 1.000000000000000000 ) ) ;
#4251=CARTESIAN_POINT ( 'NONE',  ( -67.57122606711153878, -25.90531549336015971, -21.65063509461098334 ) ) ;
#4252=DIRECTION ( 'NONE',  ( -0.9876526153536336894, -0.1566598588826349503, 0.000000000000000000 ) ) ;
#4253=ORIENTED_EDGE ( 'NONE', *, *, #10939, .T. ) ;
#4254=CIRCLE ( 'NONE', #13336, 1.500000000000000444 ) ;
#4257=CARTESIAN_POINT ( 'NONE',  ( -29.21749237908258223, -82.58968536893642920, 17.32050807568881368 ) ) ;
#4258=FACE_BOUND ( 'NONE', #10149, .T. ) ;
#4259=CYLINDRICAL_SURFACE ( 'NONE', #1006, 1.500000000000001554 ) ;
#4260=CIRCLE ( 'NONE', #1842, 1.500000000000000000 ) ;
#4261=CARTESIAN_POINT ( 'NONE',  ( -20.86208015875458344, -23.55889513208593655, 12.99038105676661736 ) ) ;
#4262=DIRECTION ( 'NONE',  ( -0.1566598588826321192, 0.9876526153536342445, 7.798540720466730171E-17 ) ) ;
#4263=ORIENTED_EDGE ( 'NONE', *, *, #5442, .F. ) ;
#4265=FACE_OUTER_BOUND ( 'NONE', #2447, .T. ) ;
#4267=ORIENTED_EDGE ( 'NONE', *, *, #11314, .F. ) ;
#4268=EDGE_LOOP ( 'NONE', ( #2639, #8226 ) ) ;
#4269=CARTESIAN_POINT ( 'NONE',  ( -10.78120068427780964, -16.89737360760884144, -17.32050807568878170 ) ) ;
#4271=CIRCLE ( 'NONE', #9648, 1.500000000000001332 ) ;
#4272=FACE_BOUND ( 'NONE', #9666, .T. ) ;
#4273=EDGE_CURVE ( 'NONE', #12329, #886, #2704, .T. ) ;
#4274=DIRECTION ( 'NONE',  ( 0.000000000000000000, 0.000000000000000000, 1.000000000000000000 ) ) ;
#4275=AXIS2_PLACEMENT_3D ( 'NONE', #14532, #11650, #14253 ) ;
#4276=DIRECTION ( 'NONE',  ( 1.000000000000000000, 0.000000000000000000, 0.000000000000000000 ) ) ;
#4277=EDGE_LOOP ( 'NONE', ( #9126, #1921, #3542, #12695 ) ) ;
#4280=VERTEX_POINT ( 'NONE', #285 ) ;
#4281=VECTOR ( 'NONE', #9561, 1000.000000000000000 ) ;
#4282=AXIS2_PLACEMENT_3D ( 'NONE', #11392, #17215, #6397 ) ;
#4284=CYLINDRICAL_SURFACE ( 'NONE', #9987, 1.500000000000000888 ) ;
#4285=EDGE_CURVE ( 'NONE', #9461, #7705, #15151, .T. ) ;
#4286=DIRECTION ( 'NONE',  ( 0.000000000000000000, 0.000000000000000000, 1.000000000000000000 ) ) ;
#4287=CIRCLE ( 'NONE', #14285, 1.500000000000000444 ) ;
#4289=EDGE_LOOP ( 'NONE', ( #7155, #3052 ) ) ;
#4290=VERTEX_POINT ( 'NONE', #17842 ) ;
#4291=EDGE_LOOP ( 'NONE', ( #12304, #12229, #16969, #10131 ) ) ;
#4292=CARTESIAN_POINT ( 'NONE',  ( -16.87183468716221313, -80.63143713290352821, -4.330127018922185655 ) ) ;
#4293=EDGE_CURVE ( 'NONE', #15166, #18004, #7010, .T. ) ;
#4294=EDGE_CURVE ( 'NONE', #12874, #10229, #13927, .T. ) ;
#4295=ORIENTED_EDGE ( 'NONE', *, *, #12442, .T. ) ;
#4296=FACE_BOUND ( 'NONE', #13349, .T. ) ;
#4297=EDGE_CURVE ( 'NONE', #16444, #4718, #2754, .T. ) ;
#4298=DIRECTION ( 'NONE',  ( -0.1566598588826321747, 0.9876526153536343555, 0.000000000000000000 ) ) ;
#4299=ORIENTED_EDGE ( 'NONE', *, *, #10177, .F. ) ;
#4300=DIRECTION ( 'NONE',  ( -0.1566598588826321192, 0.9876526153536342445, 7.798540720466730171E-17 ) ) ;
#4301=DIRECTION ( 'NONE',  ( 1.000000000000000000, 0.000000000000000000, -0.000000000000000000 ) ) ;
#4302=CIRCLE ( 'NONE', #14888, 1.499999999999999556 ) ;
#4303=DIRECTION ( 'NONE',  ( 0.000000000000000000, 0.000000000000000000, 1.000000000000000000 ) ) ;
#4305=CARTESIAN_POINT ( 'NONE',  ( 1.893565004556770903, -77.65489981413351472, 1.096166233436304165E-14 ) ) ;
#4306=DIRECTION ( 'NONE',  ( 0.000000000000000000, 0.000000000000000000, 1.000000000000000000 ) ) ;
#4307=AXIS2_PLACEMENT_3D ( 'NONE', #4829, #18044, #9389 ) ;
#4309=ORIENTED_EDGE ( 'NONE', *, *, #1871, .F. ) ;
#4310=VERTEX_POINT ( 'NONE', #15244 ) ;
#4311=CARTESIAN_POINT ( 'NONE',  ( -71.02801022084922522, -26.45362499944937440, -12.99038105676658006 ) ) ;
#4312=DIRECTION ( 'NONE',  ( -0.9876526153536341335, -0.1566598588826327576, 0.000000000000000000 ) ) ;
#4314=EDGE_CURVE ( 'NONE', #6912, #5315, #9405, .T. ) ;
#4315=ADVANCED_FACE ( 'NONE', ( #7866 ), #6462, .F. ) ;
#4316=CIRCLE ( 'NONE', #14615, 1.500000000000000000 ) ;
#4317=ORIENTED_EDGE ( 'NONE', *, *, #6276, .T. ) ;
#4318=ORIENTED_EDGE ( 'NONE', *, *, #4629, .F. ) ;
#4319=CARTESIAN_POINT ( 'NONE',  ( -63.78533391645962780, -88.07278042982854060, 17.32050807568881368 ) ) ;
#4321=EDGE_CURVE ( 'NONE', #7992, #7156, #3388, .T. ) ;
#4322=CYLINDRICAL_SURFACE ( 'NONE', #17916, 1.500000000000001554 ) ;
#4323=CARTESIAN_POINT ( 'NONE',  ( -18.39294862037050393, -23.16724548487935564, 1.869203119972154228E-14 ) ) ;
#4324=CARTESIAN_POINT ( 'NONE',  ( -66.78792677269838407, -30.84357857012830095, -4.330127018922181215 ) ) ;
#4325=ORIENTED_EDGE ( 'NONE', *, *, #16497, .F. ) ;
#4326=AXIS2_PLACEMENT_3D ( 'NONE', #10608, #16209, #17747 ) ;
#4327=DIRECTION ( 'NONE',  ( -0.9876526153536336894, -0.1566598588826349503, 0.000000000000000000 ) ) ;
#4329=DIRECTION ( 'NONE',  ( -0.9876526153536336894, -0.1566598588826349503, 0.000000000000000000 ) ) ;
#4330=CARTESIAN_POINT ( 'NONE',  ( -53.94844277310117064, -28.80700040465408662, 4.330127018922217630 ) ) ;
#4331=DIRECTION ( 'NONE',  ( 0.000000000000000000, 0.000000000000000000, 1.000000000000000000 ) ) ;
#4332=DIRECTION ( 'NONE',  ( -0.9876526153536341335, -0.1566598588826327021, 0.000000000000000000 ) ) ;
#4334=ORIENTED_EDGE ( 'NONE', *, *, #11593, .F. ) ;
#4335=ORIENTED_EDGE ( 'NONE', *, *, #11679, .F. ) ;
#4336=CARTESIAN_POINT ( 'NONE',  ( -66.25446545484369665, -88.46443007703510375, -21.65063509461098690 ) ) ;
#4337=ORIENTED_EDGE ( 'NONE', *, *, #3578, .T. ) ;
#4340=EDGE_CURVE ( 'NONE', #12777, #11183, #13325, .T. ) ;
#4343=EDGE_CURVE ( 'NONE', #6457, #2469, #16587, .T. ) ;
#4344=CYLINDRICAL_SURFACE ( 'NONE', #16775, 1.500000000000001554 ) ;
#4345=ORIENTED_EDGE ( 'NONE', *, *, #10580, .F. ) ;
#4346=FACE_OUTER_BOUND ( 'NONE', #13527, .T. ) ;
#4347=DIRECTION ( 'NONE',  ( -0.1566598588826321192, 0.9876526153536342445, 7.798540720466730171E-17 ) ) ;
#4348=ADVANCED_FACE ( 'NONE', ( #10873 ), #16696, .F. ) ;
#4349=CARTESIAN_POINT ( 'NONE',  ( -24.31886431249228053, -24.10720463817513703, -4.330127018922181215 ) ) ;
#4350=ORIENTED_EDGE ( 'NONE', *, *, #1649, .T. ) ;
#4352=DIRECTION ( 'NONE',  ( -0.1566598588826321192, 0.9876526153536342445, 7.798540720466730171E-17 ) ) ;
#4353=AXIS2_PLACEMENT_3D ( 'NONE', #8401, #8507, #2529 ) ;
#4354=EDGE_LOOP ( 'NONE', ( #12014, #17117 ) ) ;
#4355=ORIENTED_EDGE ( 'NONE', *, *, #15048, .F. ) ;
#4356=ORIENTED_EDGE ( 'NONE', *, *, #12590, .T. ) ;
#4357=ORIENTED_EDGE ( 'NONE', *, *, #15152, .T. ) ;
#4358=DIRECTION ( 'NONE',  ( -0.9876526153536341335, -0.1566598588826327021, 0.000000000000000000 ) ) ;
#4359=VERTEX_POINT ( 'NONE', #9276 ) ;
#4360=DIRECTION ( 'NONE',  ( -0.9876526153536336894, -0.1566598588826349503, 0.000000000000000000 ) ) ;
#4361=ORIENTED_EDGE ( 'NONE', *, *, #18102, .F. ) ;
#4364=CARTESIAN_POINT ( 'NONE',  ( -51.27495791377663181, -23.32042782179674489, -4.330127018922180326 ) ) ;
#4365=DIRECTION ( 'NONE',  ( -0.1566598588826321192, 0.9876526153536342445, 7.798540720466731404E-17 ) ) ;
#4366=ORIENTED_EDGE ( 'NONE', *, *, #9124, .T. ) ;
#4367=EDGE_CURVE ( 'NONE', #12785, #3795, #3934, .T. ) ;
#4369=EDGE_LOOP ( 'NONE', ( #7507, #5555 ) ) ;
#4371=DIRECTION ( 'NONE',  ( 0.000000000000000000, 0.000000000000000000, 1.000000000000000000 ) ) ;
#4372=FACE_OUTER_BOUND ( 'NONE', #18179, .T. ) ;
#4373=CARTESIAN_POINT ( 'NONE',  ( -21.64537945316773460, -18.62063205531779175, -21.65063509461097979 ) ) ;
#4375=FACE_BOUND ( 'NONE', #16095, .T. ) ;
#4376=CARTESIAN_POINT ( 'NONE',  ( -8.516422466834198346, -21.60064689605303911, 17.32050807568881012 ) ) ;
#4377=ORIENTED_EDGE ( 'NONE', *, *, #15869, .T. ) ;
#4378=EDGE_LOOP ( 'NONE', ( #9533, #10 ) ) ;
#4379=VERTEX_POINT ( 'NONE', #4615 ) ;
#4380=VERTEX_POINT ( 'NONE', #11703 ) ;
#4382=VERTEX_POINT ( 'NONE', #3009 ) ;
#4383=VECTOR ( 'NONE', #5984, 1000.000000000000000 ) ;
#4384=FACE_BOUND ( 'NONE', #4033, .T. ) ;
#4386=DIRECTION ( 'NONE',  ( 0.000000000000000000, 0.000000000000000000, 1.000000000000000000 ) ) ;
#4388=ADVANCED_FACE ( 'NONE', ( #6055 ), #13332, .F. ) ;
#4392=DIRECTION ( 'NONE',  ( -0.1566598588826321192, 0.9876526153536342445, 7.798540720466731404E-17 ) ) ;
#4393=EDGE_CURVE ( 'NONE', #15929, #18110, #7595, .T. ) ;
#4394=DIRECTION ( 'NONE',  ( -0.1566598588826321192, 0.9876526153536342445, 7.798540720466731404E-17 ) ) ;
#4396=FACE_OUTER_BOUND ( 'NONE', #1097, .T. ) ;
#4398=VERTEX_POINT ( 'NONE', #18605 ) ;
#4400=VERTEX_POINT ( 'NONE', #8509 ) ;
#4401=DIRECTION ( 'NONE',  ( -0.1566598588826321747, 0.9876526153536343555, 0.000000000000000000 ) ) ;
#4402=DIRECTION ( 'NONE',  ( 0.000000000000000000, 0.000000000000000000, 1.000000000000000000 ) ) ;
#4404=DIRECTION ( 'NONE',  ( -0.9876526153536336894, -0.1566598588826349503, 0.000000000000000000 ) ) ;
#4406=DIRECTION ( 'NONE',  ( -0.9876526153536336894, -0.1566598588826349503, 0.000000000000000000 ) ) ;
#4408=ADVANCED_FACE ( 'NONE', ( #1129 ), #12646, .T. ) ;
#4409=VECTOR ( 'NONE', #18457, 1000.000000000000000 ) ;
#4412=CARTESIAN_POINT ( 'NONE',  ( -31.68662391746666884, -82.98133501614299234, -12.99038105676658539 ) ) ;
#4414=EDGE_LOOP ( 'NONE', ( #7322, #6758 ) ) ;
#4415=EDGE_LOOP ( 'NONE', ( #12895, #501, #15641, #9969 ) ) ;
#4418=DIRECTION ( 'NONE',  ( -0.9876526153536341335, -0.1566598588826327021, 0.000000000000000000 ) ) ;
#4420=ORIENTED_EDGE ( 'NONE', *, *, #4028, .F. ) ;
#4424=DIRECTION ( 'NONE',  ( 0.000000000000000000, 0.000000000000000000, 1.000000000000000000 ) ) ;
#4425=CARTESIAN_POINT ( 'NONE',  ( -49.95819730150881099, -85.87954240547166762, -21.65063509461098690 ) ) ;
#4426=CIRCLE ( 'NONE', #11670, 1.499999999999999556 ) ;
#4427=CARTESIAN_POINT ( 'NONE',  ( -15.88418207180859021, -80.47477727402089442, -8.660254037844385522 ) ) ;
#4428=LINE ( 'NONE', #15828, #2360 ) ;
#4429=CARTESIAN_POINT ( 'NONE',  ( -56.21322099054479082, -24.10372711620989605, -21.65063509461097979 ) ) ;
#4430=ORIENTED_EDGE ( 'NONE', *, *, #1045, .T. ) ;
#4431=CARTESIAN_POINT ( 'NONE',  ( 1.893565004556770903, -77.65489981413351472, -8.660254037844385522 ) ) ;
#4432=AXIS2_PLACEMENT_3D ( 'NONE', #14024, #9772, #9938 ) ;
#4433=CARTESIAN_POINT ( 'NONE',  ( -13.41505053342451426, -80.08312762681433128, -4.330127018922185655 ) ) ;
#4436=VERTEX_POINT ( 'NONE', #7369 ) ;
#4437=EDGE_CURVE ( 'NONE', #15703, #17521, #4260, .T. ) ;
#4440=LINE ( 'NONE', #3024, #11684 ) ;
#4441=AXIS2_PLACEMENT_3D ( 'NONE', #725, #16651, #6508 ) ;
#4442=ORIENTED_EDGE ( 'NONE', *, *, #12055, .F. ) ;
#4443=CIRCLE ( 'NONE', #2028, 1.500000000000000888 ) ;
#4444=ORIENTED_EDGE ( 'NONE', *, *, #5295, .T. ) ;
#4445=DIRECTION ( 'NONE',  ( -0.1566598588826321192, 0.9876526153536342445, 7.798540720466730171E-17 ) ) ;
#4446=EDGE_CURVE ( 'NONE', #10913, #2476, #17311, .T. ) ;
#4447=AXIS2_PLACEMENT_3D ( 'NONE', #3735, #3825, #4890 ) ;
#4448=FACE_BOUND ( 'NONE', #2249, .T. ) ;
#4449=ORIENTED_EDGE ( 'NONE', *, *, #10314, .T. ) ;
#4450=CARTESIAN_POINT ( 'NONE',  ( -42.87991068327077926, -21.98881902129437549, -4.330127018922180326 ) ) ;
#4454=FACE_BOUND ( 'NONE', #5287, .T. ) ;
#4455=AXIS2_PLACEMENT_3D ( 'NONE', #2180, #3208, #9104 ) ;
#4458=LINE ( 'NONE', #1278, #13621 ) ;
#4459=LINE ( 'NONE', #9182, #8788 ) ;
#4460=CYLINDRICAL_SURFACE ( 'NONE', #4196, 1.500000000000000666 ) ;
#4461=AXIS2_PLACEMENT_3D ( 'NONE', #7220, #16682, #10684 ) ;
#4462=CYLINDRICAL_SURFACE ( 'NONE', #8748, 1.500000000000001554 ) ;
#4463=VERTEX_POINT ( 'NONE', #11677 ) ;
#4464=EDGE_LOOP ( 'NONE', ( #18502, #1164, #4687, #10917 ) ) ;
#4467=VERTEX_POINT ( 'NONE', #5931 ) ;
#4468=CARTESIAN_POINT ( 'NONE',  ( -12.75650591498505371, -17.21069332537411256, 1.926565525561698076E-14 ) ) ;
#4469=EDGE_CURVE ( 'NONE', #10372, #12073, #153, .T. ) ;
#4470=ORIENTED_EDGE ( 'NONE', *, *, #16230, .T. ) ;
#4471=FACE_BOUND ( 'NONE', #6433, .T. ) ;
#4475=CIRCLE ( 'NONE', #15942, 1.500000000000000888 ) ;
#4476=EDGE_LOOP ( 'NONE', ( #17899, #1840, #16199, #5121 ) ) ;
#4477=AXIS2_PLACEMENT_3D ( 'NONE', #228, #3338, #3152 ) ;
#4478=FACE_BOUND ( 'NONE', #17233, .T. ) ;
#4479=CIRCLE ( 'NONE', #557, 1.499999999999999556 ) ;
#4480=VECTOR ( 'NONE', #6702, 1000.000000000000000 ) ;
#4481=CARTESIAN_POINT ( 'NONE',  ( -29.05277406831996245, -19.79558099693754158, 17.32050807568882078 ) ) ;
#4483=DIRECTION ( 'NONE',  ( -0.1566598588826321747, 0.9876526153536343555, 0.000000000000000000 ) ) ;
#4485=CARTESIAN_POINT ( 'NONE',  ( -81.73462711737164454, 33.01666666666666572, 30.00000000000000000 ) ) ;
#4488=VERTEX_POINT ( 'NONE', #68 ) ;
#4489=EDGE_LOOP ( 'NONE', ( #15605, #13376, #4659, #17869 ) ) ;
#4490=DIRECTION ( 'NONE',  ( -0.9876526153536341335, -0.1566598588826327021, 0.000000000000000000 ) ) ;
#4491=DIRECTION ( 'NONE',  ( -0.1566598588826321192, 0.9876526153536342445, 7.798540720466730171E-17 ) ) ;
#4493=EDGE_CURVE ( 'NONE', #13102, #17604, #15719, .T. ) ;
#4495=ORIENTED_EDGE ( 'NONE', *, *, #6919, .F. ) ;
#4496=DIRECTION ( 'NONE',  ( -0.000000000000000000, -0.000000000000000000, -1.000000000000000000 ) ) ;
#4497=EDGE_LOOP ( 'NONE', ( #6515, #13015 ) ) ;
#4499=ADVANCED_FACE ( 'NONE', ( #15802 ), #6026, .F. ) ;
#4501=DIRECTION ( 'NONE',  ( 0.000000000000000000, 0.000000000000000000, 1.000000000000000000 ) ) ;
#4503=CARTESIAN_POINT ( 'NONE',  ( -54.73174206751433957, -23.86873732788595248, -21.65063509461098334 ) ) ;
#4504=CIRCLE ( 'NONE', #6954, 1.500000000000000888 ) ;
#4505=CARTESIAN_POINT ( 'NONE',  ( -43.86756329862440396, -22.14547888017701638, 17.32050807568882078 ) ) ;
#4506=DIRECTION ( 'NONE',  ( -0.1566598588826321192, 0.9876526153536342445, 7.798540720466730171E-17 ) ) ;
#4508=ORIENTED_EDGE ( 'NONE', *, *, #8569, .F. ) ;
#4510=AXIS2_PLACEMENT_3D ( 'NONE', #4873, #3252, #6321 ) ;
#4511=EDGE_LOOP ( 'NONE', ( #7483, #18589, #4964, #2663 ) ) ;
#4512=CARTESIAN_POINT ( 'NONE',  ( -55.42992169613163611, -29.04199019297804085, -21.65063509461098334 ) ) ;
#4513=ORIENTED_EDGE ( 'NONE', *, *, #16228, .T. ) ;
#4517=CIRCLE ( 'NONE', #7547, 1.500000000000000888 ) ;
#4518=CARTESIAN_POINT ( 'NONE',  ( -34.97868976044173195, -20.73554015023332653, -4.330127018922180326 ) ) ;
#4519=EDGE_LOOP ( 'NONE', ( #17371, #5776 ) ) ;
#4520=CIRCLE ( 'NONE', #18509, 1.499999999999999556 ) ;
#4521=CYLINDRICAL_SURFACE ( 'NONE', #13942, 1.500000000000001554 ) ;
#4522=DIRECTION ( 'NONE',  ( -0.1566598588826321747, 0.9876526153536343555, 0.000000000000000000 ) ) ;
#4523=CIRCLE ( 'NONE', #17270, 1.500000000000001332 ) ;
#4524=AXIS2_PLACEMENT_3D ( 'NONE', #2304, #15491, #18289 ) ;
#4525=CARTESIAN_POINT ( 'NONE',  ( -45.34904222165485521, -22.38046866850095640, 1.908195823574487804E-14 ) ) ;
#4528=ORIENTED_EDGE ( 'NONE', *, *, #149, .F. ) ;
#4529=DIRECTION ( 'NONE',  ( -0.1566598588826321192, 0.9876526153536342445, 7.798540720466730171E-17 ) ) ;
#4530=FACE_BOUND ( 'NONE', #4175, .T. ) ;
#4531=VECTOR ( 'NONE', #6232, 1000.000000000000000 ) ;
#4532=DIRECTION ( 'NONE',  ( -0.1566598588826321747, 0.9876526153536343555, 0.000000000000000000 ) ) ;
#4533=LINE ( 'NONE', #8005, #11464 ) ;
#4534=AXIS2_PLACEMENT_3D ( 'NONE', #14999, #4483, #13287 ) ;
#4535=CARTESIAN_POINT ( 'NONE',  ( -66.78792677269838407, -30.84357857012830095, -21.65063509461098334 ) ) ;
#4536=DIRECTION ( 'NONE',  ( -0.9876526153536341335, -0.1566598588826327021, 0.000000000000000000 ) ) ;
#4537=ORIENTED_EDGE ( 'NONE', *, *, #224, .T. ) ;
#4541=CIRCLE ( 'NONE', #6672, 1.500000000000001332 ) ;
#4542=EDGE_LOOP ( 'NONE', ( #11693, #8331, #12039, #7668 ) ) ;
#4543=EDGE_LOOP ( 'NONE', ( #17886, #4014 ) ) ;
#4545=DIRECTION ( 'NONE',  ( -0.1566598588826321192, 0.9876526153536342445, 7.798540720466730171E-17 ) ) ;
#4546=CIRCLE ( 'NONE', #18532, 1.500000000000000000 ) ;
#4547=DIRECTION ( 'NONE',  ( -0.9876526153536344665, -0.1566598588826304539, 0.000000000000000000 ) ) ;
#4548=AXIS2_PLACEMENT_3D ( 'NONE', #2777, #13423, #15044 ) ;
#4549=VERTEX_POINT ( 'NONE', #2978 ) ;
#4552=ADVANCED_FACE ( 'NONE', ( #15109 ), #6320, .T. ) ;
#4554=CIRCLE ( 'NONE', #17811, 1.500000000000000888 ) ;
#4555=ORIENTED_EDGE ( 'NONE', *, *, #1349, .F. ) ;
#4556=FACE_BOUND ( 'NONE', #13903, .T. ) ;
#4557=AXIS2_PLACEMENT_3D ( 'NONE', #13117, #3157, #11500 ) ;
#4559=EDGE_LOOP ( 'NONE', ( #6568, #5457 ) ) ;
#4560=CARTESIAN_POINT ( 'NONE',  ( -54.73174206751432536, -23.86873732788596314, 4.330127018922218518 ) ) ;
#4563=CARTESIAN_POINT ( 'NONE',  ( -68.72359699322777260, -88.85607972424169532, 8.660254037844412167 ) ) ;
#4564=ORIENTED_EDGE ( 'NONE', *, *, #9378, .F. ) ;
#4565=ORIENTED_EDGE ( 'NONE', *, *, #2752, .F. ) ;
#4566=ORIENTED_EDGE ( 'NONE', *, *, #19, .F. ) ;
#4568=FACE_BOUND ( 'NONE', #10941, .T. ) ;
#4569=CARTESIAN_POINT ( 'NONE',  ( -43.04462899403342391, -84.78292339329327376, -21.65063509461098690 ) ) ;
#4570=ORIENTED_EDGE ( 'NONE', *, *, #9491, .T. ) ;
#4571=LINE ( 'NONE', #17590, #3039 ) ;
#4572=EDGE_LOOP ( 'NONE', ( #6973, #5826, #13187, #15819 ) ) ;
#4575=VERTEX_POINT ( 'NONE', #7644 ) ;
#4576=DIRECTION ( 'NONE',  ( -0.1566598588826321192, 0.9876526153536342445, 7.798540720466730171E-17 ) ) ;
#4577=VECTOR ( 'NONE', #6642, 1000.000000000000000 ) ;
#4578=EDGE_CURVE ( 'NONE', #14627, #6069, #3007, .T. ) ;
#4579=DIRECTION ( 'NONE',  ( -0.1566598588826321192, 0.9876526153536342445, 7.798540720466731404E-17 ) ) ;
#4580=CARTESIAN_POINT ( 'NONE',  ( -61.15148406731293562, -24.88702641062306498, 4.330127018922218518 ) ) ;
#4581=VECTOR ( 'NONE', #4191, 1000.000000000000000 ) ;
#4583=DIRECTION ( 'NONE',  ( -0.9876526153536336894, -0.1566598588826349503, 0.000000000000000000 ) ) ;
#4585=ORIENTED_EDGE ( 'NONE', *, *, #2521, .T. ) ;
#4586=FACE_BOUND ( 'NONE', #17262, .T. ) ;
#4588=CARTESIAN_POINT ( 'NONE',  ( -6.995308533625909320, -79.06483854407720457, -21.65063509461098690 ) ) ;
#4589=CIRCLE ( 'NONE', #14578, 1.499999999999999556 ) ;
#4590=ORIENTED_EDGE ( 'NONE', *, *, #15913, .T. ) ;
#4591=CARTESIAN_POINT ( 'NONE',  ( 10.28861223506262412, -76.32329101363113466, 17.32050807568880657 ) ) ;
#4594=CIRCLE ( 'NONE', #5204, 1.500000000000000888 ) ;
#4595=DIRECTION ( 'NONE',  ( -0.1566598588826321192, 0.9876526153536342445, 7.798540720466731404E-17 ) ) ;
#4597=DIRECTION ( 'NONE',  ( -0.1566598588826321192, 0.9876526153536342445, 7.798540720466730171E-17 ) ) ;
#4598=AXIS2_PLACEMENT_3D ( 'NONE', #10700, #2750, #14216 ) ;
#4599=ADVANCED_FACE ( 'NONE', ( #6130 ), #3436, .F. ) ;
#4600=DIRECTION ( 'NONE',  ( -0.9876526153536336894, -0.1566598588826349503, 0.000000000000000000 ) ) ;
#4601=CARTESIAN_POINT ( 'NONE',  ( -75.96627329761737712, -27.23692429386254332, 12.99038105676661736 ) ) ;
#4602=EDGE_LOOP ( 'NONE', ( #494, #8655 ) ) ;
#4603=DIRECTION ( 'NONE',  ( -0.1566598588826321192, 0.9876526153536342445, 7.798540720466730171E-17 ) ) ;
#4604=ORIENTED_EDGE ( 'NONE', *, *, #6698, .F. ) ;
#4609=EDGE_CURVE ( 'NONE', #14, #730, #282, .T. ) ;
#4611=VERTEX_POINT ( 'NONE', #5048 ) ;
#4612=LINE ( 'NONE', #1869, #5971 ) ;
#4613=CARTESIAN_POINT ( 'NONE',  ( -6.047290928450125946, -21.20899724884646531, 12.99038105676661026 ) ) ;
#4614=CARTESIAN_POINT ( 'NONE',  ( -78.43540483600145308, -27.62857394106912423, 17.32050807568882078 ) ) ;
#4615=CARTESIAN_POINT ( 'NONE',  ( -21.84973277410820458, -23.71555499096855613, 1.887572821959364500E-14 ) ) ;
#4616=CARTESIAN_POINT ( 'NONE',  ( -6.007655918272284623, -78.90817868519457079, 8.660254037844408614 ) ) ;
#4618=DIRECTION ( 'NONE',  ( -0.9876526153536336894, -0.1566598588826349503, 0.000000000000000000 ) ) ;
#4620=VERTEX_POINT ( 'NONE', #10821 ) ;
#4621=DIRECTION ( 'NONE',  ( 0.000000000000000000, 0.000000000000000000, 1.000000000000000000 ) ) ;
#4622=EDGE_CURVE ( 'NONE', #227, #11803, #5757, .T. ) ;
#4623=CARTESIAN_POINT ( 'NONE',  ( 0.4120860815263194254, -77.88988960245745830, 8.660254037844408614 ) ) ;
#4624=CARTESIAN_POINT ( 'NONE',  ( -14.93616446663280328, -22.61893597879013740, -17.32050807568878170 ) ) ;
#4625=ORIENTED_EDGE ( 'NONE', *, *, #14894, .T. ) ;
#4629=EDGE_CURVE ( 'NONE', #10665, #15027, #9370, .T. ) ;
#4630=EDGE_LOOP ( 'NONE', ( #6779, #2547, #9147, #4827 ) ) ;
#4631=DIRECTION ( 'NONE',  ( -0.9876526153536341335, -0.1566598588826327021, 0.000000000000000000 ) ) ;
#4632=AXIS2_PLACEMENT_3D ( 'NONE', #11061, #9472, #12493 ) ;
#4633=EDGE_CURVE ( 'NONE', #8008, #15653, #6221, .T. ) ;
#4637=DIRECTION ( 'NONE',  ( -0.9876526153536336894, -0.1566598588826350336, 0.000000000000000000 ) ) ;
#4638=CARTESIAN_POINT ( 'NONE',  ( -44.07191661956488105, -27.24040181582776299, -4.330127018922181215 ) ) ;
#4639=CYLINDRICAL_SURFACE ( 'NONE', #7371, 1.500000000000001554 ) ;
#4640=AXIS2_PLACEMENT_3D ( 'NONE', #17725, #548, #10676 ) ;
#4641=LINE ( 'NONE', #11909, #253 ) ;
#4643=EDGE_LOOP ( 'NONE', ( #10514, #16463 ) ) ;
#4644=EDGE_CURVE ( 'NONE', #8469, #5396, #16641, .T. ) ;
#4645=ADVANCED_FACE ( 'NONE', ( #17033 ), #5258, .F. ) ;
#4646=EDGE_LOOP ( 'NONE', ( #4355, #8636 ) ) ;
#4647=CARTESIAN_POINT ( 'NONE',  ( -23.33121169713865584, -23.95054477929251036, -17.32050807568878170 ) ) ;
#4648=DIRECTION ( 'NONE',  ( 0.000000000000000000, 0.000000000000000000, 1.000000000000000000 ) ) ;
#4649=EDGE_CURVE ( 'NONE', #9397, #7505, #18185, .T. ) ;
#4650=VERTEX_POINT ( 'NONE', #2221 ) ;
#4651=EDGE_CURVE ( 'NONE', #8287, #14949, #1229, .T. ) ;
#4652=EDGE_LOOP ( 'NONE', ( #12016, #11274, #8, #15733 ) ) ;
#4653=ORIENTED_EDGE ( 'NONE', *, *, #15865, .T. ) ;
#4654=FACE_OUTER_BOUND ( 'NONE', #4714, .T. ) ;
#4655=FACE_BOUND ( 'NONE', #8658, .T. ) ;
#4656=DIRECTION ( 'NONE',  ( -0.1566598588826321192, 0.9876526153536342445, 7.798540720466731404E-17 ) ) ;
#4657=VERTEX_POINT ( 'NONE', #16746 ) ;
#4658=DIRECTION ( 'NONE',  ( -0.9876526153536336894, -0.1566598588826349503, 0.000000000000000000 ) ) ;
#4659=ORIENTED_EDGE ( 'NONE', *, *, #8346, .T. ) ;
#4660=VERTEX_POINT ( 'NONE', #15290 ) ;
#4661=ORIENTED_EDGE ( 'NONE', *, *, #3453, .F. ) ;
#4662=DIRECTION ( 'NONE',  ( -0.1566598588826321192, 0.9876526153536342445, 7.798540720466731404E-17 ) ) ;
#4663=DIRECTION ( 'NONE',  ( -0.1566598588826321192, 0.9876526153536342445, 7.798540720466730171E-17 ) ) ;
#4664=DIRECTION ( 'NONE',  ( -0.9876526153536341335, -0.1566598588826327021, 0.000000000000000000 ) ) ;
#4665=CARTESIAN_POINT ( 'NONE',  ( -66.29410046502155751, -30.76524864068697696, 17.32050807568881723 ) ) ;
#4666=DIRECTION ( 'NONE',  ( -0.9876526153536336894, -0.1566598588826349503, 0.000000000000000000 ) ) ;
#4667=ORIENTED_EDGE ( 'NONE', *, *, #10531, .T. ) ;
#4668=CARTESIAN_POINT ( 'NONE',  ( -22.79775037928398618, -81.57139628619931671, 8.660254037844412167 ) ) ;
#4669=AXIS2_PLACEMENT_3D ( 'NONE', #11417, #17146, #9833 ) ;
#4670=CARTESIAN_POINT ( 'NONE',  ( -67.73594437787414790, -88.69941986535904732, -21.65063509461098690 ) ) ;
#4671=EDGE_CURVE ( 'NONE', #10521, #1565, #12375, .T. ) ;
#4672=DIRECTION ( 'NONE',  ( -0.9876526153536336894, -0.1566598588826349503, 0.000000000000000000 ) ) ;
#4673=EDGE_CURVE ( 'NONE', #9895, #5011, #4214, .T. ) ;
#4674=EDGE_LOOP ( 'NONE', ( #5819, #12508, #1748, #15482 ) ) ;
#4676=DIRECTION ( 'NONE',  ( -0.9876526153536336894, -0.1566598588826349503, 0.000000000000000000 ) ) ;
#4677=EDGE_CURVE ( 'NONE', #9448, #10913, #8198, .T. ) ;
#4679=AXIS2_PLACEMENT_3D ( 'NONE', #10831, #3632, #638 ) ;
#4680=DIRECTION ( 'NONE',  ( 0.000000000000000000, 0.000000000000000000, 1.000000000000000000 ) ) ;
#4683=DIRECTION ( 'NONE',  ( -0.9876526153536336894, -0.1566598588826350336, 0.000000000000000000 ) ) ;
#4684=CARTESIAN_POINT ( 'NONE',  ( -25.80034323552273179, -24.34219442649909126, -12.99038105676658006 ) ) ;
#4687=ORIENTED_EDGE ( 'NONE', *, *, #15847, .T. ) ;
#4688=DIRECTION ( 'NONE',  ( -0.1566598588826321747, 0.9876526153536343555, 0.000000000000000000 ) ) ;
#4689=ORIENTED_EDGE ( 'NONE', *, *, #1191, .T. ) ;
#4690=EDGE_LOOP ( 'NONE', ( #14029, #408, #5920, #8744 ) ) ;
#4692=CARTESIAN_POINT ( 'NONE',  ( -45.55339554259532520, -27.47539160415171722, 4.330127018922217630 ) ) ;
#4693=CIRCLE ( 'NONE', #17445, 1.500000000000000888 ) ;
#4694=ORIENTED_EDGE ( 'NONE', *, *, #1223, .F. ) ;
#4696=DIRECTION ( 'NONE',  ( -0.1566598588826321192, 0.9876526153536342445, 7.798540720466730171E-17 ) ) ;
#4698=CARTESIAN_POINT ( 'NONE',  ( -81.73462711737164454, 33.01666666666666572, -35.00000000000000000 ) ) ;
#4699=VECTOR ( 'NONE', #6717, 1000.000000000000000 ) ;
#4701=ORIENTED_EDGE ( 'NONE', *, *, #9726, .F. ) ;
#4704=ADVANCED_FACE ( 'NONE', ( #2466 ), #2645, .F. ) ;
#4705=LINE ( 'NONE', #15139, #2074 ) ;
#4706=CIRCLE ( 'NONE', #15310, 1.499999999999999556 ) ;
#4707=ORIENTED_EDGE ( 'NONE', *, *, #8121, .T. ) ;
#4708=DIRECTION ( 'NONE',  ( -0.9876526153536336894, -0.1566598588826349503, 0.000000000000000000 ) ) ;
#4709=FACE_BOUND ( 'NONE', #18685, .T. ) ;
#4710=LINE ( 'NONE', #7478, #14762 ) ;
#4711=DIRECTION ( 'NONE',  ( -0.1566598588826321192, 0.9876526153536342445, 7.798540720466730171E-17 ) ) ;
#4712=ORIENTED_EDGE ( 'NONE', *, *, #12537, .T. ) ;
#4713=ORIENTED_EDGE ( 'NONE', *, *, #1558, .T. ) ;
#4714=EDGE_LOOP ( 'NONE', ( #11329, #6235, #15047, #17467 ) ) ;
#4715=CARTESIAN_POINT ( 'NONE',  ( -38.92930022185625205, -21.36217958576385811, 17.32050807568882078 ) ) ;
#4716=AXIS2_PLACEMENT_3D ( 'NONE', #4927, #13546, #1644 ) ;
#4717=EDGE_LOOP ( 'NONE', ( #11922, #16464, #4169, #8212 ) ) ;
#4718=VERTEX_POINT ( 'NONE', #7038 ) ;
#4719=CARTESIAN_POINT ( 'NONE',  ( -32.67427653282027933, -83.13799487502562613, 8.660254037844412167 ) ) ;
#4721=CARTESIAN_POINT ( 'NONE',  ( -38.10636591726525069, -83.99962409888011905, 12.99038105676661203 ) ) ;
#4722=EDGE_LOOP ( 'NONE', ( #13567, #12736, #6734, #8957 ) ) ;
#4725=DIRECTION ( 'NONE',  ( -0.1566598588826321192, 0.9876526153536342445, 7.798540720466731404E-17 ) ) ;
#4726=EDGE_CURVE ( 'NONE', #9991, #17961, #14416, .T. ) ;
#4728=DIRECTION ( 'NONE',  ( -0.9876526153536344665, -0.1566598588826304539, 0.000000000000000000 ) ) ;
#4730=LINE ( 'NONE', #17846, #887 ) ;
#4731=DIRECTION ( 'NONE',  ( -0.1566598588826321747, 0.9876526153536343555, 0.000000000000000000 ) ) ;
#4732=EDGE_LOOP ( 'NONE', ( #10994, #18364, #1318, #7024 ) ) ;
#4733=ORIENTED_EDGE ( 'NONE', *, *, #8809, .F. ) ;
#4734=CARTESIAN_POINT ( 'NONE',  ( -66.08974714408108753, -25.67032570503622324, 4.330127018922218518 ) ) ;
#4735=AXIS2_PLACEMENT_3D ( 'NONE', #6701, #10931, #3907 ) ;
#4736=AXIS2_PLACEMENT_3D ( 'NONE', #182, #7484, #7678 ) ;
#4737=CARTESIAN_POINT ( 'NONE',  ( -46.33669483700848701, -22.53712852738358308, -12.99038105676658006 ) ) ;
#4738=AXIS2_PLACEMENT_3D ( 'NONE', #14848, #3266, #13326 ) ;
#4739=ORIENTED_EDGE ( 'NONE', *, *, #6850, .T. ) ;
#4741=VERTEX_POINT ( 'NONE', #5985 ) ;
#4742=DIRECTION ( 'NONE',  ( -0.1566598588826321192, 0.9876526153536342445, 7.798540720466730171E-17 ) ) ;
#4744=EDGE_CURVE ( 'NONE', #15183, #8278, #10570, .T. ) ;
#4745=AXIS2_PLACEMENT_3D ( 'NONE', #9639, #2434, #544 ) ;
#4747=EDGE_LOOP ( 'NONE', ( #17109, #4783 ) ) ;
#4748=FACE_BOUND ( 'NONE', #1438, .T. ) ;
#4749=EDGE_CURVE ( 'NONE', #3169, #450, #4817, .T. ) ;
#4751=ORIENTED_EDGE ( 'NONE', *, *, #17417, .F. ) ;
#4752=ORIENTED_EDGE ( 'NONE', *, *, #1192, .F. ) ;
#4754=VERTEX_POINT ( 'NONE', #15846 ) ;
#4756=FACE_BOUND ( 'NONE', #566, .T. ) ;
#4757=VECTOR ( 'NONE', #330, 1000.000000000000000 ) ;
#4758=FACE_OUTER_BOUND ( 'NONE', #8170, .T. ) ;
#4760=DIRECTION ( 'NONE',  ( -0.1566598588826321747, 0.9876526153536343555, 0.000000000000000000 ) ) ;
#4761=CARTESIAN_POINT ( 'NONE',  ( -19.38060123572412863, -23.32390534376198232, -21.65063509461098334 ) ) ;
#4762=CYLINDRICAL_SURFACE ( 'NONE', #12869, 1.500000000000001554 ) ;
#4763=DIRECTION ( 'NONE',  ( -0.1566598588826321192, 0.9876526153536342445, 7.798540720466730171E-17 ) ) ;
#4765=ORIENTED_EDGE ( 'NONE', *, *, #13971, .T. ) ;
#4766=CARTESIAN_POINT ( 'NONE',  ( 3.231158466157542541, -19.73726462726228803, 30.00000000000000000 ) ) ;
#4767=DIRECTION ( 'NONE',  ( -0.1566598588826321192, 0.9876526153536342445, 7.798540720466730171E-17 ) ) ;
#4769=EDGE_LOOP ( 'NONE', ( #2821, #14933, #10668, #15763 ) ) ;
#4770=ORIENTED_EDGE ( 'NONE', *, *, #16258, .T. ) ;
#4771=CARTESIAN_POINT ( 'NONE',  ( -63.82496892663748156, -30.37359899348040315, 12.99038105676661736 ) ) ;
#4772=CIRCLE ( 'NONE', #17821, 1.499999999999999556 ) ;
#4773=FACE_BOUND ( 'NONE', #639, .T. ) ;
#4775=CIRCLE ( 'NONE', #9638, 1.500000000000000888 ) ;
#4776=DIRECTION ( 'NONE',  ( -0.9876526153536336894, -0.1566598588826349503, 0.000000000000000000 ) ) ;
#4777=EDGE_CURVE ( 'NONE', #959, #2096, #17873, .T. ) ;
#4778=ORIENTED_EDGE ( 'NONE', *, *, #7970, .T. ) ;
#4779=ADVANCED_FACE ( 'NONE', ( #119 ), #14525, .F. ) ;
#4781=CYLINDRICAL_SURFACE ( 'NONE', #9585, 1.500000000000000666 ) ;
#4782=FACE_OUTER_BOUND ( 'NONE', #16015, .T. ) ;
#4783=ORIENTED_EDGE ( 'NONE', *, *, #5339, .F. ) ;
#4784=ORIENTED_EDGE ( 'NONE', *, *, #12442, .F. ) ;
#4785=CARTESIAN_POINT ( 'NONE',  ( -35.67686938905904270, -25.90879301532540779, -21.65063509461098334 ) ) ;
#4789=ORIENTED_EDGE ( 'NONE', *, *, #14726, .F. ) ;
#4790=DIRECTION ( 'NONE',  ( 0.000000000000000000, 0.000000000000000000, 1.000000000000000000 ) ) ;
#4791=VECTOR ( 'NONE', #7597, 1000.000000000000000 ) ;
#4792=DIRECTION ( 'NONE',  ( -0.1566598588826321192, 0.9876526153536342445, 7.798540720466730171E-17 ) ) ;
#4793=DIRECTION ( 'NONE',  ( 0.000000000000000000, 0.000000000000000000, 1.000000000000000000 ) ) ;
#4794=CIRCLE ( 'NONE', #15400, 1.500000000000000888 ) ;
#4796=CARTESIAN_POINT ( 'NONE',  ( -17.85948730251583783, -80.78809699178614778, -17.32050807568878525 ) ) ;
#4799=AXIS2_PLACEMENT_3D ( 'NONE', #5388, #12276, #2165 ) ;
#4800=FACE_OUTER_BOUND ( 'NONE', #8513, .T. ) ;
#4801=DIRECTION ( 'NONE',  ( -0.1566598588826321192, 0.9876526153536342445, 7.798540720466730171E-17 ) ) ;
#4804=CARTESIAN_POINT ( 'NONE',  ( 7.819480696678551723, -76.71494066083772623, 4.330127018922207860 ) ) ;
#4805=CYLINDRICAL_SURFACE ( 'NONE', #1502, 1.500000000000001554 ) ;
#4806=ORIENTED_EDGE ( 'NONE', *, *, #601, .F. ) ;
#4807=AXIS2_PLACEMENT_3D ( 'NONE', #13274, #10435, #3223 ) ;
#4808=DIRECTION ( 'NONE',  ( -0.1566598588826321747, 0.9876526153536343555, 0.000000000000000000 ) ) ;
#4809=AXIS2_PLACEMENT_3D ( 'NONE', #5803, #11540, #4358 ) ;
#4810=VERTEX_POINT ( 'NONE', #17472 ) ;
#4812=ORIENTED_EDGE ( 'NONE', *, *, #2086, .T. ) ;
#4813=CARTESIAN_POINT ( 'NONE',  ( -34.15575545585073058, -83.37298466334958391, 8.660254037844412167 ) ) ;
#4814=AXIS2_PLACEMENT_3D ( 'NONE', #2619, #2444, #8229 ) ;
#4816=AXIS2_PLACEMENT_3D ( 'NONE', #13681, #7479, #12344 ) ;
#4817=CIRCLE ( 'NONE', #15124, 1.500000000000000444 ) ;
#4818=LINE ( 'NONE', #17564, #9449 ) ;
#4819=EDGE_LOOP ( 'NONE', ( #714, #9485 ) ) ;
#4820=CARTESIAN_POINT ( 'NONE',  ( -52.26261052913027072, -23.47708768067937868, -8.660254037844380193 ) ) ;
#4821=DIRECTION ( 'NONE',  ( 0.000000000000000000, 0.000000000000000000, 1.000000000000000000 ) ) ;
#4822=DIRECTION ( 'NONE',  ( 1.000000000000000000, 0.000000000000000000, 0.000000000000000000 ) ) ;
#4823=DIRECTION ( 'NONE',  ( 0.000000000000000000, 0.000000000000000000, 1.000000000000000000 ) ) ;
#4824=CIRCLE ( 'NONE', #16980, 1.500000000000000888 ) ;
#4825=DIRECTION ( 'NONE',  ( -0.9876526153536341335, -0.1566598588826327021, 0.000000000000000000 ) ) ;
#4826=DIRECTION ( 'NONE',  ( -0.1566598588826321192, 0.9876526153536342445, 7.798540720466731404E-17 ) ) ;
#4827=ORIENTED_EDGE ( 'NONE', *, *, #3079, .T. ) ;
#4828=CIRCLE ( 'NONE', #2718, 1.500000000000000444 ) ;
#4829=CARTESIAN_POINT ( 'NONE',  ( -20.86208015875458344, -23.55889513208593655, 21.65063509461101177 ) ) ;
#4830=VERTEX_POINT ( 'NONE', #4181 ) ;
#4831=ADVANCED_FACE ( 'NONE', ( #1365 ), #9965, .F. ) ;
#4832=CARTESIAN_POINT ( 'NONE',  ( -52.96079015774756016, -28.65034054577145994, 1.869203119972154228E-14 ) ) ;
#4835=ADVANCED_FACE ( 'NONE', ( #30 ), #4460, .F. ) ;
#4837=AXIS2_PLACEMENT_3D ( 'NONE', #9345, #6810, #1042 ) ;
#4838=ORIENTED_EDGE ( 'NONE', *, *, #14687, .T. ) ;
#4839=DIRECTION ( 'NONE',  ( -0.9876526153536336894, -0.1566598588826349503, 0.000000000000000000 ) ) ;
#4840=ORIENTED_EDGE ( 'NONE', *, *, #3895, .F. ) ;
#4841=CIRCLE ( 'NONE', #17293, 1.499999999999999556 ) ;
#4842=FACE_BOUND ( 'NONE', #13068, .T. ) ;
#4844=EDGE_LOOP ( 'NONE', ( #15254, #1407 ) ) ;
#4846=AXIS2_PLACEMENT_3D ( 'NONE', #6368, #2177, #15058 ) ;
#4847=EDGE_LOOP ( 'NONE', ( #11935, #177, #16663, #3020 ) ) ;
#4848=EDGE_LOOP ( 'NONE', ( #6680, #3325 ) ) ;
#4850=AXIS2_PLACEMENT_3D ( 'NONE', #3801, #12049, #16534 ) ;
#4851=CARTESIAN_POINT ( 'NONE',  ( -88.14047854185180597, 6.938893903907228378E-15, 30.00000000000000000 ) ) ;
#4853=DIRECTION ( 'NONE',  ( -0.9876526153536341335, -0.1566598588826327021, 0.000000000000000000 ) ) ;
#4854=CARTESIAN_POINT ( 'NONE',  ( -5.349111299832828514, -16.03574438375436984, 4.330127018922214965 ) ) ;
#4855=LINE ( 'NONE', #11860, #2277 ) ;
#4858=ORIENTED_EDGE ( 'NONE', *, *, #17861, .F. ) ;
#4859=ORIENTED_EDGE ( 'NONE', *, *, #960, .F. ) ;
#4861=EDGE_CURVE ( 'NONE', #1457, #1168, #2942, .T. ) ;
#4862=EDGE_CURVE ( 'NONE', #491, #15907, #5736, .T. ) ;
#4865=EDGE_LOOP ( 'NONE', ( #15914, #16088 ) ) ;
#4866=DIRECTION ( 'NONE',  ( -0.1566598588826321192, 0.9876526153536342445, 7.798540720466730171E-17 ) ) ;
#4867=EDGE_CURVE ( 'NONE', #18009, #9527, #5603, .T. ) ;
#4869=EDGE_LOOP ( 'NONE', ( #3151, #7094 ) ) ;
#4872=DIRECTION ( 'NONE',  ( -1.000000000000000000, 0.000000000000000000, 0.000000000000000000 ) ) ;
#4873=CARTESIAN_POINT ( 'NONE',  ( -50.49165861936347000, -28.25869089856487903, 21.65063509461101887 ) ) ;
#4874=CIRCLE ( 'NONE', #974, 1.500000000000000444 ) ;
#4876=DIRECTION ( 'NONE',  ( -0.1566598588826321192, 0.9876526153536342445, 7.798540720466731404E-17 ) ) ;
#4877=AXIS2_PLACEMENT_3D ( 'NONE', #17266, #11523, #7209 ) ;
#4878=AXIS2_PLACEMENT_3D ( 'NONE', #15267, #5328, #6956 ) ;
#4879=DIRECTION ( 'NONE',  ( -0.1566598588826321192, 0.9876526153536342445, 7.798540720466730171E-17 ) ) ;
#4881=ORIENTED_EDGE ( 'NONE', *, *, #17949, .F. ) ;
#4882=EDGE_LOOP ( 'NONE', ( #9630, #5173, #15590, #4420 ) ) ;
#4883=DIRECTION ( 'NONE',  ( -0.1566598588826321192, 0.9876526153536342445, 7.798540720466730171E-17 ) ) ;
#4885=ORIENTED_EDGE ( 'NONE', *, *, #13124, .F. ) ;
#4886=EDGE_CURVE ( 'NONE', #10150, #9162, #12048, .T. ) ;
#4890=DIRECTION ( 'NONE',  ( -0.9876526153536341335, -0.1566598588826327576, 0.000000000000000000 ) ) ;
#4892=CYLINDRICAL_SURFACE ( 'NONE', #16708, 1.500000000000001554 ) ;
#4893=CARTESIAN_POINT ( 'NONE',  ( -41.39843176024032800, -21.75382923297043547, 12.99038105676661736 ) ) ;
#4894=LINE ( 'NONE', #10678, #9444 ) ;
#4895=CYLINDRICAL_SURFACE ( 'NONE', #6005, 1.500000000000001554 ) ;
#4897=CYLINDRICAL_SURFACE ( 'NONE', #15022, 1.500000000000001554 ) ;
#4898=DIRECTION ( 'NONE',  ( 0.000000000000000000, 0.000000000000000000, 1.000000000000000000 ) ) ;
#4899=ORIENTED_EDGE ( 'NONE', *, *, #5885, .F. ) ;
#4900=DIRECTION ( 'NONE',  ( -0.1566598588826321192, 0.9876526153536342445, 7.798540720466730171E-17 ) ) ;
#4901=DIRECTION ( 'NONE',  ( -0.9876526153536336894, -0.1566598588826350336, 0.000000000000000000 ) ) ;
#4902=CARTESIAN_POINT ( 'NONE',  ( -14.23798483801550674, -17.44568311369805969, 1.908195823574487804E-14 ) ) ;
#4903=ORIENTED_EDGE ( 'NONE', *, *, #3125, .T. ) ;
#4904=CARTESIAN_POINT ( 'NONE',  ( 0.4120860815263194254, -77.88988960245745830, 8.660254037844408614 ) ) ;
#4905=ORIENTED_EDGE ( 'NONE', *, *, #4241, .F. ) ;
#4906=EDGE_CURVE ( 'NONE', #14051, #3263, #892, .T. ) ;
#4908=CIRCLE ( 'NONE', #8562, 1.500000000000000888 ) ;
#4909=EDGE_CURVE ( 'NONE', #16874, #9493, #8145, .T. ) ;
#4910=CYLINDRICAL_SURFACE ( 'NONE', #15192, 1.500000000000001554 ) ;
#4911=ORIENTED_EDGE ( 'NONE', *, *, #1108, .F. ) ;
#4912=EDGE_CURVE ( 'NONE', #15608, #6427, #2383, .T. ) ;
#4913=DIRECTION ( 'NONE',  ( -0.9876526153536336894, -0.1566598588826349503, 0.000000000000000000 ) ) ;
#4916=CARTESIAN_POINT ( 'NONE',  ( -62.83731631128386397, -30.21693913459777647, -8.660254037844380193 ) ) ;
#4917=CARTESIAN_POINT ( 'NONE',  ( -40.61513246582717329, -26.69209230973856251, -4.330127018922181215 ) ) ;
#4918=CYLINDRICAL_SURFACE ( 'NONE', #7233, 1.500000000000001554 ) ;
#4919=ORIENTED_EDGE ( 'NONE', *, *, #444, .T. ) ;
#4921=CIRCLE ( 'NONE', #16146, 1.500000000000001332 ) ;
#4922=LINE ( 'NONE', #14978, #4383 ) ;
#4923=FACE_OUTER_BOUND ( 'NONE', #469, .T. ) ;
#4924=ORIENTED_EDGE ( 'NONE', *, *, #8809, .T. ) ;
#4925=EDGE_LOOP ( 'NONE', ( #4334, #12632, #10246, #2343 ) ) ;
#4926=VERTEX_POINT ( 'NONE', #7481 ) ;
#4927=CARTESIAN_POINT ( 'NONE',  ( -51.43967622453926936, -86.11453219379563961, -4.330127018922185655 ) ) ;
#4928=FACE_BOUND ( 'NONE', #17182, .T. ) ;
#4929=VECTOR ( 'NONE', #9928, 1000.000000000000000 ) ;
#4930=EDGE_CURVE ( 'NONE', #12097, #16672, #15406, .T. ) ;
#4931=DIRECTION ( 'NONE',  ( -0.9876526153536336894, -0.1566598588826349503, 0.000000000000000000 ) ) ;
#4932=CARTESIAN_POINT ( 'NONE',  ( -75.18297400320422241, -32.17518737063066681, -4.330127018922181215 ) ) ;
#4933=EDGE_CURVE ( 'NONE', #10907, #8900, #13346, .T. ) ;
#4935=CARTESIAN_POINT ( 'NONE',  ( -64.77298653181324539, -88.22944028871116018, -4.330127018922185655 ) ) ;
#4937=CARTESIAN_POINT ( 'NONE',  ( -84.16561914167408531, 33.59999999999999432, 30.00000000000000000 ) ) ;
#4939=EDGE_LOOP ( 'NONE', ( #17204, #16241 ) ) ;
#4940=DIRECTION ( 'NONE',  ( -0.9876526153536341335, -0.1566598588826327021, 0.000000000000000000 ) ) ;
#4942=ORIENTED_EDGE ( 'NONE', *, *, #8587, .T. ) ;
#4945=CARTESIAN_POINT ( 'NONE',  ( -32.67427653282027933, -83.13799487502562613, 1.443110928631665584E-14 ) ) ;
#4946=DIRECTION ( 'NONE',  ( -0.1566598588826321192, 0.9876526153536342445, 7.798540720466730171E-17 ) ) ;
#4947=ORIENTED_EDGE ( 'NONE', *, *, #7098, .T. ) ;
#4949=DIRECTION ( 'NONE',  ( -0.9876526153536336894, -0.1566598588826349503, 0.000000000000000000 ) ) ;
#4951=DIRECTION ( 'NONE',  ( -0.1566598588826321747, 0.9876526153536343555, 0.000000000000000000 ) ) ;
#4953=ADVANCED_FACE ( 'NONE', ( #6355 ), #7676, .F. ) ;
#4956=DIRECTION ( 'NONE',  ( -0.9876526153536341335, -0.1566598588826327021, 0.000000000000000000 ) ) ;
#4957=CARTESIAN_POINT ( 'NONE',  ( -68.55887868246516348, -26.06197535224279704, -8.660254037844380193 ) ) ;
#4960=VERTEX_POINT ( 'NONE', #7754 ) ;
#4961=CYLINDRICAL_SURFACE ( 'NONE', #15159, 1.500000000000001554 ) ;
#4962=ORIENTED_EDGE ( 'NONE', *, *, #6335, .T. ) ;
#4963=CARTESIAN_POINT ( 'NONE',  ( 11.77009115809307715, -76.08830122530719109, 17.32050807568880657 ) ) ;
#4964=ORIENTED_EDGE ( 'NONE', *, *, #1647, .T. ) ;
#4965=EDGE_CURVE ( 'NONE', #9953, #2455, #11452, .T. ) ;
#4967=DIRECTION ( 'NONE',  ( -0.9876526153536341335, -0.1566598588826327576, 0.000000000000000000 ) ) ;
#4968=EDGE_CURVE ( 'NONE', #62, #3665, #1696, .T. ) ;
#4970=DIRECTION ( 'NONE',  ( -0.1566598588826321192, 0.9876526153536342445, 7.798540720466731404E-17 ) ) ;
#4971=CARTESIAN_POINT ( 'NONE',  ( -5.349111299832828514, -16.03574438375436984, 12.99038105676661026 ) ) ;
#4972=DIRECTION ( 'NONE',  ( -0.9876526153536336894, -0.1566598588826349503, 0.000000000000000000 ) ) ;
#4973=FACE_OUTER_BOUND ( 'NONE', #9022, .T. ) ;
#4975=LINE ( 'NONE', #2159, #14190 ) ;
#4976=FACE_OUTER_BOUND ( 'NONE', #12617, .T. ) ;
#4977=DIRECTION ( 'NONE',  ( -0.1566598588826321192, 0.9876526153536342445, 7.798540720466731404E-17 ) ) ;
#4978=VERTEX_POINT ( 'NONE', #10400 ) ;
#4979=LINE ( 'NONE', #14952, #10594 ) ;
#4981=CARTESIAN_POINT ( 'NONE',  ( 1.360103686702108128, -20.03404830722672259, 8.660254037844412167 ) ) ;
#4982=EDGE_LOOP ( 'NONE', ( #7342, #3670 ) ) ;
#4983=CARTESIAN_POINT ( 'NONE',  ( -19.17624791478365864, -18.22898240811121440, -8.660254037844380193 ) ) ;
#4984=EDGE_LOOP ( 'NONE', ( #11825, #15237, #1387, #11714 ) ) ;
#4985=ORIENTED_EDGE ( 'NONE', *, *, #17809, .T. ) ;
#4987=DIRECTION ( 'NONE',  ( -0.9876526153536341335, -0.1566598588826327021, 0.000000000000000000 ) ) ;
#4988=EDGE_LOOP ( 'NONE', ( #54, #14843 ) ) ;
#4989=DIRECTION ( 'NONE',  ( -0.9876526153536341335, -0.1566598588826327021, 0.000000000000000000 ) ) ;
#4990=AXIS2_PLACEMENT_3D ( 'NONE', #16732, #2386, #9504 ) ;
#4992=DIRECTION ( 'NONE',  ( -0.1566598588826321192, 0.9876526153536342445, 7.798540720466730171E-17 ) ) ;
#4993=CYLINDRICAL_SURFACE ( 'NONE', #12746, 1.500000000000001554 ) ;
#4994=DIRECTION ( 'NONE',  ( -0.9876526153536341335, -0.1566598588826327021, 0.000000000000000000 ) ) ;
#4995=DIRECTION ( 'NONE',  ( -0.9876526153536336894, -0.1566598588826349503, 0.000000000000000000 ) ) ;
#4996=VERTEX_POINT ( 'NONE', #1786 ) ;
#4997=CARTESIAN_POINT ( 'NONE',  ( -10.98555400521827963, -21.99229654325962002, -4.330127018922181215 ) ) ;
#4998=VERTEX_POINT ( 'NONE', #11896 ) ;
#4999=ADVANCED_FACE ( 'NONE', ( #465 ), #4805, .F. ) ;
#5000=ADVANCED_FACE ( 'NONE', ( #10491 ), #16285, .F. ) ;
#5001=CARTESIAN_POINT ( 'NONE',  ( -71.72618984946653597, -31.62687786454144856, 21.65063509461101887 ) ) ;
#5003=AXIS2_PLACEMENT_3D ( 'NONE', #16912, #13943, #2576 ) ;
#5004=DIRECTION ( 'NONE',  ( -0.9876526153536341335, -0.1566598588826327576, 0.000000000000000000 ) ) ;
#5006=FACE_BOUND ( 'NONE', #6253, .T. ) ;
#5010=EDGE_LOOP ( 'NONE', ( #5235, #13979, #10166, #10428 ) ) ;
#5011=VERTEX_POINT ( 'NONE', #664 ) ;
#5012=ORIENTED_EDGE ( 'NONE', *, *, #10660, .T. ) ;
#5013=CARTESIAN_POINT ( 'NONE',  ( -26.78799585087635649, -24.49885428538171794, 8.660254037844417496 ) ) ;
#5014=ORIENTED_EDGE ( 'NONE', *, *, #7525, .F. ) ;
#5015=FACE_BOUND ( 'NONE', #18674, .T. ) ;
#5016=ORIENTED_EDGE ( 'NONE', *, *, #3125, .F. ) ;
#5017=CARTESIAN_POINT ( 'NONE',  ( -36.46016868347218320, -20.97052993855727365, 4.330127018922218518 ) ) ;
#5019=AXIS2_PLACEMENT_3D ( 'NONE', #4505, #73, #17344 ) ;
#5020=FACE_BOUND ( 'NONE', #511, .T. ) ;
#5021=CARTESIAN_POINT ( 'NONE',  ( -16.87183468716221313, -80.63143713290352821, -21.65063509461098690 ) ) ;
#5022=ORIENTED_EDGE ( 'NONE', *, *, #13522, .F. ) ;
#5023=CARTESIAN_POINT ( 'NONE',  ( 6.831828081324923474, -76.87160051972034580, 17.32050807568880657 ) ) ;
#5026=ORIENTED_EDGE ( 'NONE', *, *, #11038, .F. ) ;
#5027=CARTESIAN_POINT ( 'NONE',  ( -73.49714175923330117, -26.84527464665595531, -8.660254037844380193 ) ) ;
#5029=ADVANCED_FACE ( 'NONE', ( #13514 ), #13425, .F. ) ;
#5030=CARTESIAN_POINT ( 'NONE',  ( -66.78792677269838407, -30.84357857012830095, -12.99038105676658006 ) ) ;
#5031=ORIENTED_EDGE ( 'NONE', *, *, #1119, .T. ) ;
#5032=CARTESIAN_POINT ( 'NONE',  ( -14.40270314877813895, -80.23978748569695085, 1.424741226644455312E-14 ) ) ;
#5033=CARTESIAN_POINT ( 'NONE',  ( 0.3724510713484785462, -20.19070816610934926, -21.65063509461098334 ) ) ;
#5034=EDGE_LOOP ( 'NONE', ( #6830, #5867, #11121, #17385 ) ) ;
#5035=DIRECTION ( 'NONE',  ( 0.000000000000000000, 0.000000000000000000, 1.000000000000000000 ) ) ;
#5036=ORIENTED_EDGE ( 'NONE', *, *, #362, .T. ) ;
#5038=ORIENTED_EDGE ( 'NONE', *, *, #653, .F. ) ;
#5039=FACE_OUTER_BOUND ( 'NONE', #12305, .T. ) ;
#5040=EDGE_CURVE ( 'NONE', #18006, #3093, #1782, .T. ) ;
#5041=AXIS2_PLACEMENT_3D ( 'NONE', #7584, #13072, #16399 ) ;
#5042=DIRECTION ( 'NONE',  ( -0.1566598588826321192, 0.9876526153536342445, 7.798540720466730171E-17 ) ) ;
#5043=EDGE_LOOP ( 'NONE', ( #6788, #14911 ) ) ;
#5045=FACE_BOUND ( 'NONE', #4819, .T. ) ;
#5046=CIRCLE ( 'NONE', #7492, 1.500000000000001332 ) ;
#5047=CARTESIAN_POINT ( 'NONE',  ( -30.73860631229088369, -25.12549372091224598, 4.330127018922217630 ) ) ;
#5048=CARTESIAN_POINT ( 'NONE',  ( -79.24244631363546887, 32.81909429640987952, -30.00000000000000000 ) ) ;
#5049=DIRECTION ( 'NONE',  ( -0.1566598588826321192, 0.9876526153536342445, 7.798540720466730171E-17 ) ) ;
#5051=CARTESIAN_POINT ( 'NONE',  ( -18.18859529943003750, -18.07232254922858417, 21.65063509461101177 ) ) ;
#5052=DIRECTION ( 'NONE',  ( -0.1566598588826321192, 0.9876526153536342445, 7.798540720466730171E-17 ) ) ;
#5056=CARTESIAN_POINT ( 'NONE',  ( -38.10636591726527911, -83.99962409888010484, -21.65063509461098690 ) ) ;
#5057=CARTESIAN_POINT ( 'NONE',  ( -15.92381708198643153, -22.77559583767277473, 21.65063509461101177 ) ) ;
#5059=VERTEX_POINT ( 'NONE', #5292 ) ;
#5061=EDGE_CURVE ( 'NONE', #9479, #18003, #3841, .T. ) ;
#5062=ORIENTED_EDGE ( 'NONE', *, *, #6970, .F. ) ;
#5063=ORIENTED_EDGE ( 'NONE', *, *, #7474, .F. ) ;
#5064=ORIENTED_EDGE ( 'NONE', *, *, #13666, .T. ) ;
#5065=ADVANCED_FACE ( 'NONE', ( #1056 ), #18421, .F. ) ;
#5066=CYLINDRICAL_SURFACE ( 'NONE', #6022, 1.500000000000001554 ) ;
#5067=CYLINDRICAL_SURFACE ( 'NONE', #12906, 1.500000000000001554 ) ;
#5069=ORIENTED_EDGE ( 'NONE', *, *, #2307, .F. ) ;
#5070=DIRECTION ( 'NONE',  ( -0.9876526153536336894, -0.1566598588826349503, 0.000000000000000000 ) ) ;
#5073=CARTESIAN_POINT ( 'NONE',  ( -32.22008523532134205, -25.36048350923618955, 4.330127018922217630 ) ) ;
#5075=DIRECTION ( 'NONE',  ( -0.9876526153536341335, -0.1566598588826327021, 0.000000000000000000 ) ) ;
#5078=CARTESIAN_POINT ( 'NONE',  ( -41.56315007100294423, -84.54793360496931598, 12.99038105676661203 ) ) ;
#5079=AXIS2_PLACEMENT_3D ( 'NONE', #14440, #18754, #1294 ) ;
#5080=CARTESIAN_POINT ( 'NONE',  ( -68.72359699322777260, -88.85607972424168111, -8.660254037844385522 ) ) ;
#5081=ORIENTED_EDGE ( 'NONE', *, *, #1319, .F. ) ;
#5083=EDGE_CURVE ( 'NONE', #6519, #9513, #9949, .T. ) ;
#5084=FACE_OUTER_BOUND ( 'NONE', #4717, .T. ) ;
#5085=CARTESIAN_POINT ( 'NONE',  ( -16.70711637639958269, -17.83733276090463704, 12.99038105676661381 ) ) ;
#5086=ORIENTED_EDGE ( 'NONE', *, *, #11457, .F. ) ;
#5088=EDGE_CURVE ( 'NONE', #3468, #14246, #16640, .T. ) ;
#5089=DIRECTION ( 'NONE',  ( -0.9876526153536341335, -0.1566598588826327021, 0.000000000000000000 ) ) ;
#5090=EDGE_CURVE ( 'NONE', #8278, #15183, #591, .T. ) ;
#5091=ORIENTED_EDGE ( 'NONE', *, *, #10771, .T. ) ;
#5093=LINE ( 'NONE', #10867, #3904 ) ;
#5095=LINE ( 'NONE', #8038, #296 ) ;
#5097=DIRECTION ( 'NONE',  ( 1.000000000000000000, 0.000000000000000000, 0.000000000000000000 ) ) ;
#5098=ORIENTED_EDGE ( 'NONE', *, *, #6813, .T. ) ;
#5099=CIRCLE ( 'NONE', #8737, 1.500000000000001332 ) ;
#5100=LINE ( 'NONE', #8042, #9467 ) ;
#5102=DIRECTION ( 'NONE',  ( -0.1566598588826321192, 0.9876526153536342445, 7.798540720466730171E-17 ) ) ;
#5104=DIRECTION ( 'NONE',  ( -0.1566598588826321192, 0.9876526153536342445, 7.798540720466731404E-17 ) ) ;
#5105=CARTESIAN_POINT ( 'NONE',  ( -68.76323200340561925, -31.15689828789355786, -21.65063509461098334 ) ) ;
#5106=CARTESIAN_POINT ( 'NONE',  ( -78.43540483600145308, -27.62857394106912423, 17.32050807568882078 ) ) ;
#5107=CARTESIAN_POINT ( 'NONE',  ( -42.87991068327079347, -21.98881902129436838, -21.65063509461098334 ) ) ;
#5108=VERTEX_POINT ( 'NONE', #15146 ) ;
#5109=CIRCLE ( 'NONE', #9363, 1.500000000000000444 ) ;
#5110=LINE ( 'NONE', #585, #7648 ) ;
#5111=DIRECTION ( 'NONE',  ( -0.1566598588826321747, 0.9876526153536343555, 0.000000000000000000 ) ) ;
#5112=AXIS2_PLACEMENT_3D ( 'NONE', #14114, #5515, #11270 ) ;
#5113=AXIS2_PLACEMENT_3D ( 'NONE', #15886, #11778, #4600 ) ;
#5114=EDGE_CURVE ( 'NONE', #1113, #202, #2991, .T. ) ;
#5116=VECTOR ( 'NONE', #914, 1000.000000000000000 ) ;
#5119=ORIENTED_EDGE ( 'NONE', *, *, #13310, .F. ) ;
#5121=ORIENTED_EDGE ( 'NONE', *, *, #7378, .F. ) ;
#5122=CYLINDRICAL_SURFACE ( 'NONE', #16539, 1.500000000000001554 ) ;
#5123=EDGE_LOOP ( 'NONE', ( #15285, #4770, #3531, #17351 ) ) ;
#5124=FACE_BOUND ( 'NONE', #17158, .T. ) ;
#5125=EDGE_CURVE ( 'NONE', #1703, #8251, #13579, .T. ) ;
#5126=CIRCLE ( 'NONE', #3297, 1.500000000000001332 ) ;
#5127=AXIS2_PLACEMENT_3D ( 'NONE', #12925, #14286, #5471 ) ;
#5128=EDGE_CURVE ( 'NONE', #17749, #11803, #14388, .T. ) ;
#5129=AXIS2_PLACEMENT_3D ( 'NONE', #12225, #9502, #16515 ) ;
#5131=CIRCLE ( 'NONE', #18205, 2.500000000000002220 ) ;
#5133=DIRECTION ( 'NONE',  ( 0.000000000000000000, 0.000000000000000000, 1.000000000000000000 ) ) ;
#5135=CARTESIAN_POINT ( 'NONE',  ( -60.36818477289978091, -29.82528948739120267, -12.99038105676658006 ) ) ;
#5136=ORIENTED_EDGE ( 'NONE', *, *, #14044, .T. ) ;
#5137=FACE_OUTER_BOUND ( 'NONE', #13046, .T. ) ;
#5138=CARTESIAN_POINT ( 'NONE',  ( -71.72618984946653597, -31.62687786454144856, -21.65063509461098334 ) ) ;
#5140=CARTESIAN_POINT ( 'NONE',  ( -50.49165861936347710, -28.25869089856488614, -4.330127018922181215 ) ) ;
#5141=ORIENTED_EDGE ( 'NONE', *, *, #17517, .T. ) ;
#5142=ORIENTED_EDGE ( 'NONE', *, *, #10711, .T. ) ;
#5146=DIRECTION ( 'NONE',  ( 0.000000000000000000, 0.000000000000000000, 1.000000000000000000 ) ) ;
#5147=ORIENTED_EDGE ( 'NONE', *, *, #11792, .F. ) ;
#5148=VERTEX_POINT ( 'NONE', #8414 ) ;
#5149=CIRCLE ( 'NONE', #12405, 1.500000000000001332 ) ;
#5150=CARTESIAN_POINT ( 'NONE',  ( -18.39294862037050393, -23.16724548487935564, -8.660254037844380193 ) ) ;
#5151=ORIENTED_EDGE ( 'NONE', *, *, #6193, .F. ) ;
#5152=VERTEX_POINT ( 'NONE', #7113 ) ;
#5153=ORIENTED_EDGE ( 'NONE', *, *, #5243, .F. ) ;
#5155=ADVANCED_FACE ( 'NONE', ( #12941 ), #12656, .F. ) ;
#5156=DIRECTION ( 'NONE',  ( -0.9876526153536336894, -0.1566598588826349503, 0.000000000000000000 ) ) ;
#5157=CARTESIAN_POINT ( 'NONE',  ( 6.338001773648100468, -76.94993044916168401, 21.65063509461100821 ) ) ;
#5158=EDGE_CURVE ( 'NONE', #93, #4467, #15107, .T. ) ;
#5159=FACE_BOUND ( 'NONE', #1486, .T. ) ;
#5160=VECTOR ( 'NONE', #12833, 1000.000000000000000 ) ;
#5161=LINE ( 'NONE', #9519, #8195 ) ;
#5162=ADVANCED_FACE ( 'NONE', ( #13041 ), #2992, .F. ) ;
#5164=CARTESIAN_POINT ( 'NONE',  ( -62.83731631128386397, -30.21693913459777647, -8.660254037844380193 ) ) ;
#5167=CARTESIAN_POINT ( 'NONE',  ( 2.881217619910392269, -77.49823995525089515, -21.65063509461098690 ) ) ;
#5168=VECTOR ( 'NONE', #3159, 1000.000000000000000 ) ;
#5169=CARTESIAN_POINT ( 'NONE',  ( -38.92930022185625205, -21.36217958576383680, 1.214306433183764966E-14 ) ) ;
#5170=CARTESIAN_POINT ( 'NONE',  ( -15.39035576413176187, -80.39644734457957043, -4.330127018922185655 ) ) ;
#5171=AXIS2_PLACEMENT_3D ( 'NONE', #2811, #12838, #12923 ) ;
#5172=CYLINDRICAL_SURFACE ( 'NONE', #6520, 1.500000000000001554 ) ;
#5173=ORIENTED_EDGE ( 'NONE', *, *, #4933, .T. ) ;
#5174=EDGE_LOOP ( 'NONE', ( #7389, #2368 ) ) ;
#5175=DIRECTION ( 'NONE',  ( -0.1566598588826321192, 0.9876526153536342445, 7.798540720466730171E-17 ) ) ;
#5177=CIRCLE ( 'NONE', #10308, 1.500000000000000888 ) ;
#5178=CARTESIAN_POINT ( 'NONE',  ( -72.71384246482016067, -31.78353772342409300, -17.32050807568878170 ) ) ;
#5181=DIRECTION ( 'NONE',  ( -0.1566598588826321192, 0.9876526153536342445, 7.798540720466730171E-17 ) ) ;
#5182=CARTESIAN_POINT ( 'NONE',  ( -51.43967622453925514, -86.11453219379563961, 12.99038105676661203 ) ) ;
#5183=AXIS2_PLACEMENT_3D ( 'NONE', #5150, #9423, #3992 ) ;
#5184=CARTESIAN_POINT ( 'NONE',  ( -55.42992169613163611, -29.04199019297804085, -12.99038105676658006 ) ) ;
#5185=DIRECTION ( 'NONE',  ( -0.1566598588826321192, 0.9876526153536342445, 7.798540720466731404E-17 ) ) ;
#5186=AXIS2_PLACEMENT_3D ( 'NONE', #9044, #17986, #4676 ) ;
#5187=EDGE_LOOP ( 'NONE', ( #16418, #5453, #16871, #7830 ) ) ;
#5188=CYLINDRICAL_SURFACE ( 'NONE', #9410, 1.500000000000001554 ) ;
#5189=EDGE_CURVE ( 'NONE', #7443, #8527, #10273, .T. ) ;
#5190=LINE ( 'NONE', #11133, #16787 ) ;
#5192=CYLINDRICAL_SURFACE ( 'NONE', #14296, 1.500000000000001554 ) ;
#5193=CIRCLE ( 'NONE', #8224, 1.500000000000000000 ) ;
#5195=DIRECTION ( 'NONE',  ( -0.1566598588826321747, 0.9876526153536343555, 0.000000000000000000 ) ) ;
#5196=CARTESIAN_POINT ( 'NONE',  ( -26.74836084069850983, -82.19803572172985184, 4.330127018922213189 ) ) ;
#5197=ADVANCED_FACE ( 'NONE', ( #4035 ), #12767, .F. ) ;
#5198=CYLINDRICAL_SURFACE ( 'NONE', #3247, 1.500000000000000666 ) ;
#5200=CARTESIAN_POINT ( 'NONE',  ( -25.59598991458226536, -19.24727149084831623, -17.32050807568878170 ) ) ;
#5201=CARTESIAN_POINT ( 'NONE',  ( -68.72359699322777260, -88.85607972424169532, 17.32050807568881368 ) ) ;
#5202=CARTESIAN_POINT ( 'NONE',  ( -21.64537945316773460, -18.62063205531779175, -21.65063509461097979 ) ) ;
#5203=VERTEX_POINT ( 'NONE', #10105 ) ;
#5204=AXIS2_PLACEMENT_3D ( 'NONE', #18644, #5707, #17185 ) ;
#5205=DIRECTION ( 'NONE',  ( 0.000000000000000000, 0.000000000000000000, 1.000000000000000000 ) ) ;
#5206=CYLINDRICAL_SURFACE ( 'NONE', #25, 1.500000000000000666 ) ;
#5207=ORIENTED_EDGE ( 'NONE', *, *, #3058, .T. ) ;
#5210=DIRECTION ( 'NONE',  ( -0.1566598588826321747, 0.9876526153536343555, 0.000000000000000000 ) ) ;
#5211=CARTESIAN_POINT ( 'NONE',  ( -26.58364252993588650, -19.40393134973096068, 12.99038105676661736 ) ) ;
#5214=CARTESIAN_POINT ( 'NONE',  ( -67.77557938805200877, -31.00023842901093118, 17.32050807568881723 ) ) ;
#5215=CARTESIAN_POINT ( 'NONE',  ( -39.13365354279673625, -26.45710252141460828, -21.65063509461098334 ) ) ;
#5216=EDGE_CURVE ( 'NONE', #3364, #5781, #1503, .T. ) ;
#5217=EDGE_CURVE ( 'NONE', #9201, #15912, #4213, .T. ) ;
#5218=LINE ( 'NONE', #6645, #11724 ) ;
#5219=FACE_OUTER_BOUND ( 'NONE', #10013, .T. ) ;
#5220=DIRECTION ( 'NONE',  ( -0.1566598588826321192, 0.9876526153536342445, 7.798540720466730171E-17 ) ) ;
#5222=ORIENTED_EDGE ( 'NONE', *, *, #9229, .T. ) ;
#5223=EDGE_CURVE ( 'NONE', #11862, #3864, #2062, .T. ) ;
#5224=DIRECTION ( 'NONE',  ( 0.000000000000000000, 0.000000000000000000, 1.000000000000000000 ) ) ;
#5225=DIRECTION ( 'NONE',  ( -0.1566598588826321192, 0.9876526153536342445, 7.798540720466731404E-17 ) ) ;
#5226=CARTESIAN_POINT ( 'NONE',  ( -16.87183468716221313, -80.63143713290352821, 4.330127018922213189 ) ) ;
#5227=AXIS2_PLACEMENT_3D ( 'NONE', #15553, #8354, #5326 ) ;
#5228=ORIENTED_EDGE ( 'NONE', *, *, #11524, .T. ) ;
#5230=VERTEX_POINT ( 'NONE', #8522 ) ;
#5231=EDGE_LOOP ( 'NONE', ( #15894, #11648 ) ) ;
#5233=FACE_BOUND ( 'NONE', #3960, .T. ) ;
#5234=DIRECTION ( 'NONE',  ( -0.9876526153536341335, -0.1566598588826327021, 0.000000000000000000 ) ) ;
#5235=ORIENTED_EDGE ( 'NONE', *, *, #10858, .F. ) ;
#5236=EDGE_CURVE ( 'NONE', #7636, #17961, #14298, .T. ) ;
#5237=CIRCLE ( 'NONE', #9784, 1.500000000000000888 ) ;
#5238=ORIENTED_EDGE ( 'NONE', *, *, #14131, .T. ) ;
#5239=CARTESIAN_POINT ( 'NONE',  ( -63.62061560569701157, -25.27867605782963523, -17.32050807568878170 ) ) ;
#5240=ORIENTED_EDGE ( 'NONE', *, *, #4437, .F. ) ;
#5241=DIRECTION ( 'NONE',  ( -0.1566598588826321192, 0.9876526153536342445, 7.798540720466730171E-17 ) ) ;
#5242=DIRECTION ( 'NONE',  ( -0.1566598588826321192, 0.9876526153536342445, 7.798540720466730171E-17 ) ) ;
#5243=EDGE_CURVE ( 'NONE', #755, #1263, #11767, .T. ) ;
#5245=ORIENTED_EDGE ( 'NONE', *, *, #18253, .T. ) ;
#5246=FACE_OUTER_BOUND ( 'NONE', #12849, .T. ) ;
#5247=ORIENTED_EDGE ( 'NONE', *, *, #13225, .T. ) ;
#5248=FACE_OUTER_BOUND ( 'NONE', #15637, .T. ) ;
#5249=VERTEX_POINT ( 'NONE', #16805 ) ;
#5250=VERTEX_POINT ( 'NONE', #2473 ) ;
#5252=CIRCLE ( 'NONE', #14026, 1.500000000000000888 ) ;
#5253=FACE_OUTER_BOUND ( 'NONE', #5034, .T. ) ;
#5255=CARTESIAN_POINT ( 'NONE',  ( -0.9046745307415022808, -15.33077501878252136, -17.32050807568878170 ) ) ;
#5256=ORIENTED_EDGE ( 'NONE', *, *, #394, .T. ) ;
#5258=CYLINDRICAL_SURFACE ( 'NONE', #16659, 1.500000000000000888 ) ;
#5259=CARTESIAN_POINT ( 'NONE',  ( -3.044698072211382112, -78.43819910854666944, -17.32050807568878525 ) ) ;
#5263=DIRECTION ( 'NONE',  ( -0.1566598588826321747, 0.9876526153536343555, 0.000000000000000000 ) ) ;
#5264=EDGE_CURVE ( 'NONE', #14963, #13690, #17575, .T. ) ;
#5265=CYLINDRICAL_SURFACE ( 'NONE', #9028, 1.500000000000000666 ) ;
#5267=ORIENTED_EDGE ( 'NONE', *, *, #2782, .F. ) ;
#5269=ORIENTED_EDGE ( 'NONE', *, *, #10087, .F. ) ;
#5270=DIRECTION ( 'NONE',  ( -0.1566598588826321192, 0.9876526153536342445, 7.798540720466730171E-17 ) ) ;
#5271=VERTEX_POINT ( 'NONE', #5313 ) ;
#5272=ORIENTED_EDGE ( 'NONE', *, *, #18701, .F. ) ;
#5273=ORIENTED_EDGE ( 'NONE', *, *, #16069, .T. ) ;
#5275=DIRECTION ( 'NONE',  ( -0.1566598588826321192, 0.9876526153536342445, 7.798540720466730171E-17 ) ) ;
#5276=ORIENTED_EDGE ( 'NONE', *, *, #2289, .T. ) ;
#5277=CARTESIAN_POINT ( 'NONE',  ( -67.24211807019732134, -88.62108993591773753, -8.660254037844385522 ) ) ;
#5278=DIRECTION ( 'NONE',  ( -0.1566598588826321192, 0.9876526153536342445, 7.798540720466730171E-17 ) ) ;
#5280=VERTEX_POINT ( 'NONE', #8261 ) ;
#5281=CARTESIAN_POINT ( 'NONE',  ( -16.87183468716221313, -80.63143713290354242, 21.65063509461101532 ) ) ;
#5282=CARTESIAN_POINT ( 'NONE',  ( -1.109027851681966492, -20.42569795443330349, 21.65063509461101177 ) ) ;
#5283=DIRECTION ( 'NONE',  ( -0.9876526153536336894, -0.1566598588826349503, 0.000000000000000000 ) ) ;
#5285=ORIENTED_EDGE ( 'NONE', *, *, #12389, .F. ) ;
#5286=CARTESIAN_POINT ( 'NONE',  ( -20.32861884089991023, -81.17974663899272514, -4.330127018922185655 ) ) ;
#5287=EDGE_LOOP ( 'NONE', ( #593, #15852 ) ) ;
#5288=DIRECTION ( 'NONE',  ( -0.1566598588826321192, 0.9876526153536342445, 7.798540720466731404E-17 ) ) ;
#5289=FACE_OUTER_BOUND ( 'NONE', #13039, .T. ) ;
#5290=DIRECTION ( 'NONE',  ( -0.9876526153536336894, -0.1566598588826349503, 0.000000000000000000 ) ) ;
#5292=CARTESIAN_POINT ( 'NONE',  ( 3.231158466157545206, -19.73726462726228092, 30.00000000000000000 ) ) ;
#5293=ORIENTED_EDGE ( 'NONE', *, *, #15041, .F. ) ;
#5294=DIRECTION ( 'NONE',  ( -0.1566598588826321192, 0.9876526153536342445, 7.798540720466730171E-17 ) ) ;
#5295=EDGE_CURVE ( 'NONE', #1415, #2898, #6053, .T. ) ;
#5296=AXIS2_PLACEMENT_3D ( 'NONE', #9960, #15756, #2776 ) ;
#5297=ORIENTED_EDGE ( 'NONE', *, *, #3696, .T. ) ;
#5298=ORIENTED_EDGE ( 'NONE', *, *, #4886, .T. ) ;
#5299=EDGE_LOOP ( 'NONE', ( #2856, #14891 ) ) ;
#5300=DIRECTION ( 'NONE',  ( -0.1566598588826321192, 0.9876526153536342445, 7.798540720466731404E-17 ) ) ;
#5301=DIRECTION ( 'NONE',  ( 0.000000000000000000, 0.000000000000000000, 1.000000000000000000 ) ) ;
#5302=EDGE_CURVE ( 'NONE', #12897, #370, #8764, .T. ) ;
#5303=CYLINDRICAL_SURFACE ( 'NONE', #15136, 1.500000000000001554 ) ;
#5304=CYLINDRICAL_SURFACE ( 'NONE', #17373, 1.500000000000000666 ) ;
#5305=EDGE_CURVE ( 'NONE', #6856, #18075, #4523, .T. ) ;
#5307=CARTESIAN_POINT ( 'NONE',  ( -0.5755665338273089349, -78.04654946134009208, -12.99038105676658539 ) ) ;
#5308=DIRECTION ( 'NONE',  ( -0.1566598588826321747, 0.9876526153536343555, 0.000000000000000000 ) ) ;
#5309=DIRECTION ( 'NONE',  ( -0.1566598588826321192, 0.9876526153536342445, 7.798540720466730171E-17 ) ) ;
#5310=AXIS2_PLACEMENT_3D ( 'NONE', #4684, #10466, #13316 ) ;
#5312=DIRECTION ( 'NONE',  ( -0.1566598588826321192, 0.9876526153536342445, 7.798540720466730171E-17 ) ) ;
#5313=CARTESIAN_POINT ( 'NONE',  ( -61.35583738825339850, -29.98194934627382224, 17.32050807568881723 ) ) ;
#5315=VERTEX_POINT ( 'NONE', #15541 ) ;
#5317=CARTESIAN_POINT ( 'NONE',  ( -41.39843176024032800, -21.75382923297043902, 21.65063509461102242 ) ) ;
#5319=ORIENTED_EDGE ( 'NONE', *, *, #18794, .F. ) ;
#5320=ORIENTED_EDGE ( 'NONE', *, *, #18052, .F. ) ;
#5321=CARTESIAN_POINT ( 'NONE',  ( -17.69476899175320739, -17.99399261978726727, -17.32050807568878170 ) ) ;
#5322=EDGE_CURVE ( 'NONE', #11461, #5108, #16920, .T. ) ;
#5323=FACE_BOUND ( 'NONE', #18165, .T. ) ;
#5325=CARTESIAN_POINT ( 'NONE',  ( 10.28861223506262412, -76.32329101363113466, -17.32050807568878525 ) ) ;
#5326=DIRECTION ( 'NONE',  ( -0.9876526153536336894, -0.1566598588826350336, 0.000000000000000000 ) ) ;
#5327=ORIENTED_EDGE ( 'NONE', *, *, #5083, .F. ) ;
#5328=DIRECTION ( 'NONE',  ( -0.1566598588826321192, 0.9876526153536342445, 7.798540720466731404E-17 ) ) ;
#5329=LINE ( 'NONE', #1362, #14099 ) ;
#5330=DIRECTION ( 'NONE',  ( -0.9876526153536336894, -0.1566598588826349503, 0.000000000000000000 ) ) ;
#5331=VECTOR ( 'NONE', #15348, 1000.000000000000000 ) ;
#5332=CARTESIAN_POINT ( 'NONE',  ( -35.14340807120434818, -83.52964452223221770, 4.330127018922213189 ) ) ;
#5333=DIRECTION ( 'NONE',  ( -0.1566598588826321192, 0.9876526153536342445, 7.798540720466730171E-17 ) ) ;
#5334=CARTESIAN_POINT ( 'NONE',  ( -45.51376053241749986, -85.17457304049983691, -8.660254037844385522 ) ) ;
#5336=DIRECTION ( 'NONE',  ( -0.1566598588826321192, 0.9876526153536342445, 7.798540720466730171E-17 ) ) ;
#5337=EDGE_CURVE ( 'NONE', #983, #17992, #16331, .T. ) ;
#5338=DIRECTION ( 'NONE',  ( -0.9876526153536341335, -0.1566598588826327021, 0.000000000000000000 ) ) ;
#5339=EDGE_CURVE ( 'NONE', #12633, #6562, #3896, .T. ) ;
#5341=ORIENTED_EDGE ( 'NONE', *, *, #11337, .T. ) ;
#5342=ORIENTED_EDGE ( 'NONE', *, *, #8909, .F. ) ;
#5343=CARTESIAN_POINT ( 'NONE',  ( -51.47931123471709469, -28.41535075744750571, 17.32050807568881723 ) ) ;
#5346=AXIS2_PLACEMENT_3D ( 'NONE', #2098, #15176, #693 ) ;
#5347=EDGE_LOOP ( 'NONE', ( #11218, #9334 ) ) ;
#5348=ORIENTED_EDGE ( 'NONE', *, *, #16081, .T. ) ;
#5350=DIRECTION ( 'NONE',  ( -0.1566598588826321192, 0.9876526153536342445, 7.798540720466730171E-17 ) ) ;
#5351=EDGE_CURVE ( 'NONE', #9530, #8822, #14522, .T. ) ;
#5352=AXIS2_PLACEMENT_3D ( 'NONE', #6727, #18413, #9649 ) ;
#5353=CARTESIAN_POINT ( 'NONE',  ( 0.000000000000000000, 0.000000000000000000, -30.00000000000000000 ) ) ;
#5356=AXIS2_PLACEMENT_3D ( 'NONE', #4813, #17834, #10501 ) ;
#5358=CARTESIAN_POINT ( 'NONE',  ( -71.02801022084922522, -26.45362499944938861, 21.65063509461102242 ) ) ;
#5359=CARTESIAN_POINT ( 'NONE',  ( -2.590506774712417748, -20.66068774275724707, -4.330127018922184767 ) ) ;
#5360=ADVANCED_FACE ( 'NONE', ( #16007 ), #9939, .F. ) ;
#5361=CARTESIAN_POINT ( 'NONE',  ( 9.300959619709004755, -76.47995087251376845, 4.330127018922207860 ) ) ;
#5362=VERTEX_POINT ( 'NONE', #2751 ) ;
#5363=ORIENTED_EDGE ( 'NONE', *, *, #12144, .F. ) ;
#5366=VERTEX_POINT ( 'NONE', #18718 ) ;
#5367=CIRCLE ( 'NONE', #840, 1.500000000000000888 ) ;
#5368=ORIENTED_EDGE ( 'NONE', *, *, #17030, .T. ) ;
#5369=AXIS2_PLACEMENT_3D ( 'NONE', #832, #6808, #18099 ) ;
#5370=ORIENTED_EDGE ( 'NONE', *, *, #6948, .T. ) ;
#5371=CARTESIAN_POINT ( 'NONE',  ( -11.76885329963143079, -17.05403346649147878, 12.99038105676661381 ) ) ;
#5372=AXIS2_PLACEMENT_3D ( 'NONE', #5919, #17498, #4583 ) ;
#5375=ORIENTED_EDGE ( 'NONE', *, *, #5351, .T. ) ;
#5376=DIRECTION ( 'NONE',  ( 1.000000000000000000, 0.000000000000000000, 0.000000000000000000 ) ) ;
#5377=EDGE_CURVE ( 'NONE', #12139, #10552, #12374, .T. ) ;
#5379=CARTESIAN_POINT ( 'NONE',  ( -39.91695283720989096, -21.51883944464647769, -21.65063509461098334 ) ) ;
#5380=AXIS2_PLACEMENT_3D ( 'NONE', #4588, #331, #16523 ) ;
#5381=ORIENTED_EDGE ( 'NONE', *, *, #12963, .T. ) ;
#5383=ORIENTED_EDGE ( 'NONE', *, *, #5544, .T. ) ;
#5384=CYLINDRICAL_SURFACE ( 'NONE', #197, 1.500000000000000666 ) ;
#5388=CARTESIAN_POINT ( 'NONE',  ( 0.4120860815263194254, -77.88988960245745830, 17.32050807568880657 ) ) ;
#5389=EDGE_LOOP ( 'NONE', ( #7582, #9462 ) ) ;
#5390=DIRECTION ( 'NONE',  ( -0.1566598588826321192, 0.9876526153536342445, 7.798540720466731404E-17 ) ) ;
#5391=ORIENTED_EDGE ( 'NONE', *, *, #7845, .T. ) ;
#5393=ORIENTED_EDGE ( 'NONE', *, *, #7421, .F. ) ;
#5394=ORIENTED_EDGE ( 'NONE', *, *, #8911, .T. ) ;
#5395=CARTESIAN_POINT ( 'NONE',  ( -24.11451099155181055, -19.01228170252437977, 8.660254037844417496 ) ) ;
#5396=VERTEX_POINT ( 'NONE', #4624 ) ;
#5398=CARTESIAN_POINT ( 'NONE',  ( -49.01017969633302584, -28.02370111024093191, -4.330127018922181215 ) ) ;
#5399=CARTESIAN_POINT ( 'NONE',  ( -35.47251606811855851, -20.81387007967463276, -17.32050807568878170 ) ) ;
#5401=AXIS2_PLACEMENT_3D ( 'NONE', #11830, #12907, #17672 ) ;
#5402=AXIS2_PLACEMENT_3D ( 'NONE', #12249, #7397, #17998 ) ;
#5403=CARTESIAN_POINT ( 'NONE',  ( -19.17624791478365864, -18.22898240811121795, 8.660254037844417496 ) ) ;
#5404=EDGE_CURVE ( 'NONE', #6176, #17712, #16542, .T. ) ;
#5405=CARTESIAN_POINT ( 'NONE',  ( -65.30644784966793281, -30.60858878180435738, -4.330127018922181215 ) ) ;
#5406=DIRECTION ( 'NONE',  ( 0.000000000000000000, 0.000000000000000000, 1.000000000000000000 ) ) ;
#5407=CYLINDRICAL_SURFACE ( 'NONE', #1466, 1.500000000000001554 ) ;
#5408=ADVANCED_FACE ( 'NONE', ( #1693 ), #637, .F. ) ;
#5410=DIRECTION ( 'NONE',  ( -0.1566598588826321192, 0.9876526153536342445, 7.798540720466730171E-17 ) ) ;
#5411=AXIS2_PLACEMENT_3D ( 'NONE', #13569, #10546, #14912 ) ;
#5413=EDGE_LOOP ( 'NONE', ( #18043, #17305, #17956, #12193 ) ) ;
#5414=DIRECTION ( 'NONE',  ( -0.1566598588826321192, 0.9876526153536342445, 7.798540720466730171E-17 ) ) ;
#5416=FACE_BOUND ( 'NONE', #14408, .T. ) ;
#5418=AXIS2_PLACEMENT_3D ( 'NONE', #7411, #14784, #1988 ) ;
#5420=EDGE_CURVE ( 'NONE', #9991, #15242, #4533, .T. ) ;
#5421=VECTOR ( 'NONE', #32, 1000.000000000000000 ) ;
#5422=CARTESIAN_POINT ( 'NONE',  ( -53.90880776292333820, -86.50618184100221697, -8.660254037844385522 ) ) ;
#5424=VECTOR ( 'NONE', #15807, 1000.000000000000000 ) ;
#5427=DIRECTION ( 'NONE',  ( -0.9876526153536336894, -0.1566598588826349503, 0.000000000000000000 ) ) ;
#5428=DIRECTION ( 'NONE',  ( 0.000000000000000000, 0.000000000000000000, 1.000000000000000000 ) ) ;
#5430=ORIENTED_EDGE ( 'NONE', *, *, #4393, .F. ) ;
#5432=DIRECTION ( 'NONE',  ( -0.1566598588826321747, 0.9876526153536343555, 0.000000000000000000 ) ) ;
#5433=ORIENTED_EDGE ( 'NONE', *, *, #2192, .T. ) ;
#5434=EDGE_LOOP ( 'NONE', ( #4564, #7316, #37, #2894 ) ) ;
#5435=CARTESIAN_POINT ( 'NONE',  ( -30.73860631229088369, -25.12549372091224598, -12.99038105676658006 ) ) ;
#5436=VECTOR ( 'NONE', #6655, 1000.000000000000000 ) ;
#5437=EDGE_LOOP ( 'NONE', ( #11627, #9516, #11835, #8571 ) ) ;
#5438=ORIENTED_EDGE ( 'NONE', *, *, #2168, .F. ) ;
#5441=AXIS2_PLACEMENT_3D ( 'NONE', #722, #13581, #6417 ) ;
#5442=EDGE_CURVE ( 'NONE', #14934, #17878, #13595, .T. ) ;
#5443=FACE_OUTER_BOUND ( 'NONE', #12130, .T. ) ;
#5445=CARTESIAN_POINT ( 'NONE',  ( -42.55080268635656893, -84.70459346385194976, 17.32050807568881368 ) ) ;
#5446=EDGE_CURVE ( 'NONE', #2096, #959, #15988, .T. ) ;
#5448=EDGE_CURVE ( 'NONE', #697, #17456, #2104, .T. ) ;
#5449=EDGE_CURVE ( 'NONE', #5280, #10517, #18464, .T. ) ;
#5452=DIRECTION ( 'NONE',  ( 0.000000000000000000, 0.000000000000000000, 1.000000000000000000 ) ) ;
#5453=ORIENTED_EDGE ( 'NONE', *, *, #4909, .F. ) ;
#5454=CARTESIAN_POINT ( 'NONE',  ( -6.047290928450125946, -21.20899724884646531, -12.99038105676658006 ) ) ;
#5456=CARTESIAN_POINT ( 'NONE',  ( -9.299721761247353058, -16.66238381928489787, 1.561251128379126385E-14 ) ) ;
#5457=ORIENTED_EDGE ( 'NONE', *, *, #7206, .T. ) ;
#5458=ORIENTED_EDGE ( 'NONE', *, *, #8356, .T. ) ;
#5459=FACE_BOUND ( 'NONE', #17099, .T. ) ;
#5460=CARTESIAN_POINT ( 'NONE',  ( -45.34904222165485521, -22.38046866850096350, 17.32050807568881723 ) ) ;
#5461=EDGE_CURVE ( 'NONE', #11609, #2300, #18197, .T. ) ;
#5462=ORIENTED_EDGE ( 'NONE', *, *, #4446, .F. ) ;
#5463=CIRCLE ( 'NONE', #16981, 1.500000000000001332 ) ;
#5464=EDGE_CURVE ( 'NONE', #8283, #15653, #7272, .T. ) ;
#5465=VERTEX_POINT ( 'NONE', #16845 ) ;
#5466=ORIENTED_EDGE ( 'NONE', *, *, #4092, .F. ) ;
#5468=CYLINDRICAL_SURFACE ( 'NONE', #16080, 1.500000000000001554 ) ;
#5469=CIRCLE ( 'NONE', #15141, 1.500000000000000888 ) ;
#5470=AXIS2_PLACEMENT_3D ( 'NONE', #11466, #17300, #1180 ) ;
#5471=DIRECTION ( 'NONE',  ( -0.9876526153536341335, -0.1566598588826327021, 0.000000000000000000 ) ) ;
#5472=EDGE_LOOP ( 'NONE', ( #17940, #13218 ) ) ;
#5473=CIRCLE ( 'NONE', #7888, 2.000000000000000000 ) ;
#5474=DIRECTION ( 'NONE',  ( -0.9876526153536336894, -0.1566598588826350336, 0.000000000000000000 ) ) ;
#5475=CYLINDRICAL_SURFACE ( 'NONE', #18287, 139.0000000000000000 ) ;
#5476=AXIS2_PLACEMENT_3D ( 'NONE', #14427, #15937, #3664 ) ;
#5477=LINE ( 'NONE', #9750, #15813 ) ;
#5478=EDGE_CURVE ( 'NONE', #8055, #6192, #9688, .T. ) ;
#5479=CARTESIAN_POINT ( 'NONE',  ( -27.28182215855319015, -24.57718421482303484, -12.99038105676658006 ) ) ;
#5480=VERTEX_POINT ( 'NONE', #2416 ) ;
#5481=CARTESIAN_POINT ( 'NONE',  ( -51.27495791377661760, -23.32042782179675555, 21.65063509461102242 ) ) ;
#5483=DIRECTION ( 'NONE',  ( -0.1566598588826321747, 0.9876526153536343555, 0.000000000000000000 ) ) ;
#5485=VERTEX_POINT ( 'NONE', #18671 ) ;
#5486=EDGE_CURVE ( 'NONE', #9818, #10692, #17531, .T. ) ;
#5488=EDGE_CURVE ( 'NONE', #11204, #8447, #3559, .T. ) ;
#5490=EDGE_CURVE ( 'NONE', #16695, #403, #1183, .T. ) ;
#5491=ORIENTED_EDGE ( 'NONE', *, *, #17021, .T. ) ;
#5493=DIRECTION ( 'NONE',  ( -0.1566598588826321192, 0.9876526153536342445, 7.798540720466730171E-17 ) ) ;
#5494=ORIENTED_EDGE ( 'NONE', *, *, #2090, .T. ) ;
#5495=ORIENTED_EDGE ( 'NONE', *, *, #17387, .T. ) ;
#5496=VECTOR ( 'NONE', #3821, 1000.000000000000000 ) ;
#5497=CARTESIAN_POINT ( 'NONE',  ( -11.76885329963143434, -17.05403346649147878, -4.330127018922180326 ) ) ;
#5498=CIRCLE ( 'NONE', #10621, 1.500000000000000888 ) ;
#5499=DIRECTION ( 'NONE',  ( -0.1566598588826321192, 0.9876526153536342445, 7.798540720466731404E-17 ) ) ;
#5500=LINE ( 'NONE', #9313, #16459 ) ;
#5503=CARTESIAN_POINT ( 'NONE',  ( -31.52190560670403841, -20.18723064414411539, 4.330127018922218518 ) ) ;
#5504=CIRCLE ( 'NONE', #14571, 1.500000000000000888 ) ;
#5505=LINE ( 'NONE', #18715, #15697 ) ;
#5506=CARTESIAN_POINT ( 'NONE',  ( -58.84707083969148300, -87.28948113541537168, -8.660254037844385522 ) ) ;
#5508=AXIS2_PLACEMENT_3D ( 'NONE', #335, #14730, #3344 ) ;
#5510=ORIENTED_EDGE ( 'NONE', *, *, #7659, .F. ) ;
#5511=EDGE_CURVE ( 'NONE', #16387, #15786, #16607, .T. ) ;
#5512=CIRCLE ( 'NONE', #3968, 1.499999999999999556 ) ;
#5513=VERTEX_POINT ( 'NONE', #1301 ) ;
#5514=ORIENTED_EDGE ( 'NONE', *, *, #8935, .F. ) ;
#5515=DIRECTION ( 'NONE',  ( -0.1566598588826321747, 0.9876526153536343555, 0.000000000000000000 ) ) ;
#5516=EDGE_LOOP ( 'NONE', ( #14133, #3059 ) ) ;
#5517=ORIENTED_EDGE ( 'NONE', *, *, #9371, .F. ) ;
#5519=AXIS2_PLACEMENT_3D ( 'NONE', #6742, #1065, #18436 ) ;
#5520=EDGE_CURVE ( 'NONE', #8134, #4611, #12625, .T. ) ;
#5521=FACE_OUTER_BOUND ( 'NONE', #269, .T. ) ;
#5522=VECTOR ( 'NONE', #11821, 1000.000000000000000 ) ;
#5523=CYLINDRICAL_SURFACE ( 'NONE', #9164, 1.500000000000000666 ) ;
#5525=VECTOR ( 'NONE', #10516, 1000.000000000000000 ) ;
#5526=DIRECTION ( 'NONE',  ( -0.1566598588826321192, 0.9876526153536342445, 7.798540720466730171E-17 ) ) ;
#5527=CARTESIAN_POINT ( 'NONE',  ( -73.49714175923330117, -26.84527464665596241, 8.660254037844417496 ) ) ;
#5528=AXIS2_PLACEMENT_3D ( 'NONE', #942, #3935, #6723 ) ;
#5529=CARTESIAN_POINT ( 'NONE',  ( -29.21749237908258223, -82.58968536893641499, -8.660254037844385522 ) ) ;
#5531=CARTESIAN_POINT ( 'NONE',  ( -14.23798483801550674, -17.44568311369805969, 17.32050807568881368 ) ) ;
#5532=CARTESIAN_POINT ( 'NONE',  ( -35.47251606811855851, -20.81387007967464342, 8.660254037844417496 ) ) ;
#5533=VERTEX_POINT ( 'NONE', #15295 ) ;
#5535=ORIENTED_EDGE ( 'NONE', *, *, #16977, .T. ) ;
#5536=ORIENTED_EDGE ( 'NONE', *, *, #1667, .F. ) ;
#5539=ORIENTED_EDGE ( 'NONE', *, *, #4862, .F. ) ;
#5540=EDGE_LOOP ( 'NONE', ( #15730, #17261 ) ) ;
#5541=ORIENTED_EDGE ( 'NONE', *, *, #2244, .T. ) ;
#5542=DIRECTION ( 'NONE',  ( -0.1566598588826321747, 0.9876526153536343555, 0.000000000000000000 ) ) ;
#5543=CARTESIAN_POINT ( 'NONE',  ( -20.86208015875458344, -23.55889513208593655, 21.65063509461101177 ) ) ;
#5544=EDGE_CURVE ( 'NONE', #9534, #9193, #11725, .T. ) ;
#5545=DIRECTION ( 'NONE',  ( -0.1566598588826321747, 0.9876526153536343555, 0.000000000000000000 ) ) ;
#5546=DIRECTION ( 'NONE',  ( -1.000000000000000000, 0.000000000000000000, 0.000000000000000000 ) ) ;
#5547=DIRECTION ( 'NONE',  ( -0.9876526153536336894, -0.1566598588826349503, 0.000000000000000000 ) ) ;
#5549=DIRECTION ( 'NONE',  ( -0.1566598588826321192, 0.9876526153536342445, 7.798540720466730171E-17 ) ) ;
#5551=CARTESIAN_POINT ( 'NONE',  ( -77.65210554158829837, -32.56683701783724416, 8.660254037844417496 ) ) ;
#5553=CARTESIAN_POINT ( 'NONE',  ( -61.15148406731293562, -24.88702641062305787, -12.99038105676658006 ) ) ;
#5554=ORIENTED_EDGE ( 'NONE', *, *, #1958, .F. ) ;
#5555=ORIENTED_EDGE ( 'NONE', *, *, #4886, .F. ) ;
#5556=AXIS2_PLACEMENT_3D ( 'NONE', #6929, #3854, #14015 ) ;
#5557=FACE_BOUND ( 'NONE', #12558, .T. ) ;
#5558=CARTESIAN_POINT ( 'NONE',  ( -16.87183468716221313, -80.63143713290352821, 4.330127018922213189 ) ) ;
#5559=ORIENTED_EDGE ( 'NONE', *, *, #14159, .F. ) ;
#5560=DIRECTION ( 'NONE',  ( -0.9876526153536336894, -0.1566598588826349503, 0.000000000000000000 ) ) ;
#5562=ORIENTED_EDGE ( 'NONE', *, *, #13982, .T. ) ;
#5563=FACE_OUTER_BOUND ( 'NONE', #7858, .T. ) ;
#5564=ADVANCED_FACE ( 'NONE', ( #8383 ), #12456, .F. ) ;
#5565=ADVANCED_FACE ( 'NONE', ( #12731 ), #5265, .F. ) ;
#5567=EDGE_CURVE ( 'NONE', #11377, #6476, #2976, .T. ) ;
#5568=ORIENTED_EDGE ( 'NONE', *, *, #15232, .F. ) ;
#5571=DIRECTION ( 'NONE',  ( -0.1566598588826321192, 0.9876526153536342445, 7.798540720466730171E-17 ) ) ;
#5572=DIRECTION ( 'NONE',  ( -0.1566598588826321192, 0.9876526153536342445, 7.798540720466731404E-17 ) ) ;
#5573=CARTESIAN_POINT ( 'NONE',  ( -47.81817376003893827, -22.77211831570753375, -4.330127018922180326 ) ) ;
#5574=ORIENTED_EDGE ( 'NONE', *, *, #14426, .T. ) ;
#5575=CARTESIAN_POINT ( 'NONE',  ( -72.01566283620284992, -26.61028485833201174, -8.660254037844380193 ) ) ;
#5577=CARTESIAN_POINT ( 'NONE',  ( -77.65210554158829837, -32.56683701783724416, -17.32050807568878170 ) ) ;
#5578=CARTESIAN_POINT ( 'NONE',  ( -14.23798483801550674, -17.44568311369805969, 17.32050807568881368 ) ) ;
#5581=DIRECTION ( 'NONE',  ( -0.1566598588826321192, 0.9876526153536342445, 7.798540720466730171E-17 ) ) ;
#5582=ORIENTED_EDGE ( 'NONE', *, *, #5264, .F. ) ;
#5583=ADVANCED_FACE ( 'NONE', ( #5642 ), #16752, .F. ) ;
#5584=DIRECTION ( 'NONE',  ( -0.9876526153536336894, -0.1566598588826349503, 0.000000000000000000 ) ) ;
#5586=EDGE_LOOP ( 'NONE', ( #83, #9291 ) ) ;
#5587=ORIENTED_EDGE ( 'NONE', *, *, #6746, .F. ) ;
#5588=EDGE_CURVE ( 'NONE', #10247, #1314, #11438, .T. ) ;
#5589=EDGE_CURVE ( 'NONE', #1314, #2452, #10357, .T. ) ;
#5590=LINE ( 'NONE', #5786, #14577 ) ;
#5591=CARTESIAN_POINT ( 'NONE',  ( -29.75095369693726610, -24.96883386202961574, -8.660254037844380193 ) ) ;
#5592=DIRECTION ( 'NONE',  ( -0.1566598588826321192, 0.9876526153536342445, 7.798540720466731404E-17 ) ) ;
#5593=DIRECTION ( 'NONE',  ( -0.1566598588826321192, 0.9876526153536342445, 7.798540720466730171E-17 ) ) ;
#5594=DIRECTION ( 'NONE',  ( 3.208277787129350839E-17, 0.000000000000000000, -1.000000000000000000 ) ) ;
#5597=DIRECTION ( 'NONE',  ( -0.9876526153536341335, -0.1566598588826327021, 0.000000000000000000 ) ) ;
#5598=DIRECTION ( 'NONE',  ( -0.1566598588826321192, 0.9876526153536342445, 7.798540720466730171E-17 ) ) ;
#5599=FACE_BOUND ( 'NONE', #2534, .T. ) ;
#5600=DIRECTION ( 'NONE',  ( 0.000000000000000000, 0.000000000000000000, 1.000000000000000000 ) ) ;
#5601=DIRECTION ( 'NONE',  ( 0.000000000000000000, 0.000000000000000000, 1.000000000000000000 ) ) ;
#5602=LINE ( 'NONE', #2839, #14461 ) ;
#5603=LINE ( 'NONE', #17173, #14510 ) ;
#5605=DIRECTION ( 'NONE',  ( -0.9876526153536336894, -0.1566598588826349503, 0.000000000000000000 ) ) ;
#5606=ORIENTED_EDGE ( 'NONE', *, *, #15024, .T. ) ;
#5607=ORIENTED_EDGE ( 'NONE', *, *, #2282, .F. ) ;
#5609=FACE_OUTER_BOUND ( 'NONE', #3726, .T. ) ;
#5610=FACE_BOUND ( 'NONE', #10738, .T. ) ;
#5611=CARTESIAN_POINT ( 'NONE',  ( -31.52190560670403841, -20.18723064414410828, -21.65063509461097979 ) ) ;
#5613=VERTEX_POINT ( 'NONE', #14717 ) ;
#5614=EDGE_CURVE ( 'NONE', #4142, #9088, #15390, .T. ) ;
#5617=FACE_BOUND ( 'NONE', #2292, .T. ) ;
#5619=DIRECTION ( 'NONE',  ( -0.1566598588826321192, 0.9876526153536342445, 7.798540720466730171E-17 ) ) ;
#5621=LINE ( 'NONE', #12809, #11196 ) ;
#5622=CARTESIAN_POINT ( 'NONE',  ( -26.74836084069850983, -82.19803572172985184, 12.99038105676661203 ) ) ;
#5623=FACE_BOUND ( 'NONE', #16632, .T. ) ;
#5625=AXIS2_PLACEMENT_3D ( 'NONE', #2802, #11663, #8940 ) ;
#5626=ORIENTED_EDGE ( 'NONE', *, *, #9038, .F. ) ;
#5627=ORIENTED_EDGE ( 'NONE', *, *, #10296, .F. ) ;
#5628=ORIENTED_EDGE ( 'NONE', *, *, #8606, .F. ) ;
#5629=CARTESIAN_POINT ( 'NONE',  ( -65.30644784966791860, -30.60858878180435028, 21.65063509461101887 ) ) ;
#5630=ORIENTED_EDGE ( 'NONE', *, *, #10300, .F. ) ;
#5631=FACE_BOUND ( 'NONE', #4240, .T. ) ;
#5633=DIRECTION ( 'NONE',  ( -0.9876526153536341335, -0.1566598588826327021, 0.000000000000000000 ) ) ;
#5634=AXIS2_PLACEMENT_3D ( 'NONE', #2753, #5799, #5601 ) ;
#5635=DIRECTION ( 'NONE',  ( -0.9876526153536336894, -0.1566598588826349503, 0.000000000000000000 ) ) ;
#5636=DIRECTION ( 'NONE',  ( -0.1566598588826321192, 0.9876526153536342445, 7.798540720466731404E-17 ) ) ;
#5637=CYLINDRICAL_SURFACE ( 'NONE', #4282, 1.500000000000001554 ) ;
#5639=EDGE_CURVE ( 'NONE', #9448, #14533, #13862, .T. ) ;
#5640=DIRECTION ( 'NONE',  ( -0.1566598588826321192, 0.9876526153536342445, 7.798540720466730171E-17 ) ) ;
#5641=DIRECTION ( 'NONE',  ( -0.9876526153536341335, -0.1566598588826327021, 0.000000000000000000 ) ) ;
#5642=FACE_OUTER_BOUND ( 'NONE', #6711, .T. ) ;
#5643=DIRECTION ( 'NONE',  ( 0.000000000000000000, 0.000000000000000000, 1.000000000000000000 ) ) ;
#5644=ORIENTED_EDGE ( 'NONE', *, *, #6966, .F. ) ;
#5645=VERTEX_POINT ( 'NONE', #13660 ) ;
#5646=DIRECTION ( 'NONE',  ( -0.000000000000000000, -0.000000000000000000, -1.000000000000000000 ) ) ;
#5647=EDGE_LOOP ( 'NONE', ( #15476, #15282, #5245, #9861 ) ) ;
#5648=AXIS2_PLACEMENT_3D ( 'NONE', #1078, #8166, #18450 ) ;
#5649=ADVANCED_FACE ( 'NONE', ( #614 ), #702, .F. ) ;
#5650=CARTESIAN_POINT ( 'NONE',  ( -18.39294862037050393, -23.16724548487935564, 8.660254037844417496 ) ) ;
#5652=ORIENTED_EDGE ( 'NONE', *, *, #3676, .F. ) ;
#5653=DIRECTION ( 'NONE',  ( -0.000000000000000000, -0.000000000000000000, -1.000000000000000000 ) ) ;
#5654=CARTESIAN_POINT ( 'NONE',  ( -68.55887868246516348, -26.06197535224280060, 1.908195823574487804E-14 ) ) ;
#5655=VERTEX_POINT ( 'NONE', #4854 ) ;
#5656=CARTESIAN_POINT ( 'NONE',  ( -2.057045456857760524, -78.28153924966404986, -12.99038105676658539 ) ) ;
#5657=CIRCLE ( 'NONE', #8062, 1.500000000000000888 ) ;
#5658=CARTESIAN_POINT ( 'NONE',  ( -23.29157668696081629, -81.64972621564064070, 4.330127018922213189 ) ) ;
#5659=DIRECTION ( 'NONE',  ( -0.9876526153536344665, -0.1566598588826304539, 0.000000000000000000 ) ) ;
#5661=EDGE_CURVE ( 'NONE', #18619, #14180, #7522, .T. ) ;
#5662=CARTESIAN_POINT ( 'NONE',  ( -13.45468554360235203, -22.38394619046619383, -8.660254037844380193 ) ) ;
#5663=AXIS2_PLACEMENT_3D ( 'NONE', #244, #6422, #12058 ) ;
#5664=ORIENTED_EDGE ( 'NONE', *, *, #15944, .F. ) ;
#5665=DIRECTION ( 'NONE',  ( -0.1566598588826321192, 0.9876526153536342445, 7.798540720466730171E-17 ) ) ;
#5666=ORIENTED_EDGE ( 'NONE', *, *, #17995, .F. ) ;
#5668=CARTESIAN_POINT ( 'NONE',  ( -50.45202360918564466, -85.95787233491300583, 1.424741226644455312E-14 ) ) ;
#5669=ORIENTED_EDGE ( 'NONE', *, *, #4965, .T. ) ;
#5671=CARTESIAN_POINT ( 'NONE',  ( -11.93357161039406300, -79.84813783849037350, -4.330127018922185655 ) ) ;
#5672=DIRECTION ( 'NONE',  ( 0.000000000000000000, 0.000000000000000000, 1.000000000000000000 ) ) ;
#5673=ORIENTED_EDGE ( 'NONE', *, *, #9562, .F. ) ;
#5674=ADVANCED_FACE ( 'NONE', ( #16238 ), #11859, .F. ) ;
#5675=AXIS2_PLACEMENT_3D ( 'NONE', #9549, #15427, #948 ) ;
#5676=CIRCLE ( 'NONE', #4745, 1.500000000000000444 ) ;
#5677=CYLINDRICAL_SURFACE ( 'NONE', #3283, 1.500000000000001554 ) ;
#5678=VERTEX_POINT ( 'NONE', #4761 ) ;
#5679=EDGE_LOOP ( 'NONE', ( #9118, #8715, #10420, #3255 ) ) ;
#5680=CIRCLE ( 'NONE', #7207, 1.500000000000001332 ) ;
#5681=DIRECTION ( 'NONE',  ( -0.1566598588826321192, 0.9876526153536342445, 7.798540720466730171E-17 ) ) ;
#5682=CIRCLE ( 'NONE', #16263, 1.500000000000001332 ) ;
#5683=ORIENTED_EDGE ( 'NONE', *, *, #169, .T. ) ;
#5685=CARTESIAN_POINT ( 'NONE',  ( -62.63296299034339398, -25.12201619894701210, 4.330127018922218518 ) ) ;
#5686=EDGE_CURVE ( 'NONE', #7926, #4290, #8132, .T. ) ;
#5687=DIRECTION ( 'NONE',  ( -0.1566598588826321192, 0.9876526153536342445, 7.798540720466730171E-17 ) ) ;
#5688=CARTESIAN_POINT ( 'NONE',  ( -61.31620237807555895, -87.68113078262194904, 4.330127018922213189 ) ) ;
#5689=VECTOR ( 'NONE', #1838, 1000.000000000000000 ) ;
#5690=DIRECTION ( 'NONE',  ( -0.1566598588826321192, 0.9876526153536342445, 7.798540720466730171E-17 ) ) ;
#5691=CYLINDRICAL_SURFACE ( 'NONE', #790, 1.500000000000001554 ) ;
#5696=ORIENTED_EDGE ( 'NONE', *, *, #10214, .F. ) ;
#5697=VECTOR ( 'NONE', #14045, 1000.000000000000000 ) ;
#5698=EDGE_CURVE ( 'NONE', #5366, #2319, #10839, .T. ) ;
#5699=ORIENTED_EDGE ( 'NONE', *, *, #17207, .F. ) ;
#5700=ORIENTED_EDGE ( 'NONE', *, *, #18466, .F. ) ;
#5701=CYLINDRICAL_SURFACE ( 'NONE', #16631, 1.500000000000001554 ) ;
#5703=ORIENTED_EDGE ( 'NONE', *, *, #8346, .F. ) ;
#5705=CIRCLE ( 'NONE', #10174, 1.500000000000000888 ) ;
#5706=ORIENTED_EDGE ( 'NONE', *, *, #118, .F. ) ;
#5707=DIRECTION ( 'NONE',  ( -0.1566598588826321747, 0.9876526153536343555, 0.000000000000000000 ) ) ;
#5708=DIRECTION ( 'NONE',  ( -0.1566598588826321192, 0.9876526153536342445, 7.798540720466730171E-17 ) ) ;
#5709=AXIS2_PLACEMENT_3D ( 'NONE', #8683, #15976, #7280 ) ;
#5710=DIRECTION ( 'NONE',  ( -0.1566598588826321747, 0.9876526153536343555, 0.000000000000000000 ) ) ;
#5711=VERTEX_POINT ( 'NONE', #9307 ) ;
#5713=ORIENTED_EDGE ( 'NONE', *, *, #3267, .T. ) ;
#5714=EDGE_CURVE ( 'NONE', #1641, #14006, #895, .T. ) ;
#5715=DIRECTION ( 'NONE',  ( -0.9876526153536336894, -0.1566598588826349503, 0.000000000000000000 ) ) ;
#5716=DIRECTION ( 'NONE',  ( -0.9876526153536341335, -0.1566598588826327021, 0.000000000000000000 ) ) ;
#5719=AXIS2_PLACEMENT_3D ( 'NONE', #7080, #12725, #4303 ) ;
#5720=ORIENTED_EDGE ( 'NONE', *, *, #174, .F. ) ;
#5721=CARTESIAN_POINT ( 'NONE',  ( -41.60278508118079799, -26.84875216862118918, 8.660254037844417496 ) ) ;
#5723=AXIS2_PLACEMENT_3D ( 'NONE', #3422, #6487, #13744 ) ;
#5724=ORIENTED_EDGE ( 'NONE', *, *, #5377, .F. ) ;
#5727=VERTEX_POINT ( 'NONE', #12704 ) ;
#5730=ORIENTED_EDGE ( 'NONE', *, *, #9435, .T. ) ;
#5731=CYLINDRICAL_SURFACE ( 'NONE', #13063, 1.500000000000000666 ) ;
#5732=AXIS2_PLACEMENT_3D ( 'NONE', #4917, #16495, #4825 ) ;
#5733=AXIS2_PLACEMENT_3D ( 'NONE', #15760, #4076, #7240 ) ;
#5734=LINE ( 'NONE', #14155, #9111 ) ;
#5736=CIRCLE ( 'NONE', #13282, 1.499999999999999556 ) ;
#5738=ORIENTED_EDGE ( 'NONE', *, *, #4127, .F. ) ;
#5740=CYLINDRICAL_SURFACE ( 'NONE', #13821, 1.500000000000001554 ) ;
#5742=VECTOR ( 'NONE', #6977, 1000.000000000000000 ) ;
#5743=DIRECTION ( 'NONE',  ( -0.1566598588826321192, 0.9876526153536342445, 7.798540720466730171E-17 ) ) ;
#5744=EDGE_LOOP ( 'NONE', ( #13268, #16049, #7515, #7025 ) ) ;
#5745=ORIENTED_EDGE ( 'NONE', *, *, #6326, .T. ) ;
#5746=FACE_OUTER_BOUND ( 'NONE', #12068, .T. ) ;
#5747=ORIENTED_EDGE ( 'NONE', *, *, #18025, .T. ) ;
#5748=CIRCLE ( 'NONE', #16027, 1.500000000000001332 ) ;
#5749=EDGE_CURVE ( 'NONE', #11814, #10450, #11736, .T. ) ;
#5750=CARTESIAN_POINT ( 'NONE',  ( 2.447859171744379392, -14.79900155049412369, 24.99999999999998934 ) ) ;
#5752=CIRCLE ( 'NONE', #16329, 1.500000000000000888 ) ;
#5753=DIRECTION ( 'NONE',  ( 0.000000000000000000, 0.000000000000000000, 1.000000000000000000 ) ) ;
#5757=CIRCLE ( 'NONE', #14226, 1.499999999999999556 ) ;
#5759=DIRECTION ( 'NONE',  ( -0.9876526153536341335, -0.1566598588826327021, 0.000000000000000000 ) ) ;
#5760=EDGE_CURVE ( 'NONE', #13736, #10706, #6965, .T. ) ;
#5761=FACE_OUTER_BOUND ( 'NONE', #10254, .T. ) ;
#5762=AXIS2_PLACEMENT_3D ( 'NONE', #18304, #8649, #18737 ) ;
#5763=AXIS2_PLACEMENT_3D ( 'NONE', #5654, #14712, #4020 ) ;
#5767=DIRECTION ( 'NONE',  ( 0.000000000000000000, 0.000000000000000000, 1.000000000000000000 ) ) ;
#5769=ORIENTED_EDGE ( 'NONE', *, *, #15359, .T. ) ;
#5771=FACE_OUTER_BOUND ( 'NONE', #9245, .T. ) ;
#5772=AXIS2_PLACEMENT_3D ( 'NONE', #13500, #18311, #9346 ) ;
#5774=CARTESIAN_POINT ( 'NONE',  ( -49.79347899074616635, -23.08543803347280843, 12.99038105676661736 ) ) ;
#5776=ORIENTED_EDGE ( 'NONE', *, *, #10421, .T. ) ;
#5780=AXIS2_PLACEMENT_3D ( 'NONE', #15522, #6819, #9836 ) ;
#5781=VERTEX_POINT ( 'NONE', #18272 ) ;
#5782=ORIENTED_EDGE ( 'NONE', *, *, #12350, .F. ) ;
#5783=AXIS2_PLACEMENT_3D ( 'NONE', #3144, #4662, #1834 ) ;
#5784=EDGE_CURVE ( 'NONE', #13518, #9146, #12319, .T. ) ;
#5785=AXIS2_PLACEMENT_3D ( 'NONE', #6233, #11963, #14935 ) ;
#5786=CARTESIAN_POINT ( 'NONE',  ( -1.069392841504132052, -78.12487939078141608, 17.32050807568880657 ) ) ;
#5787=DIRECTION ( 'NONE',  ( -0.9876526153536336894, -0.1566598588826349503, 0.000000000000000000 ) ) ;
#5788=DIRECTION ( 'NONE',  ( -0.1566598588826321192, 0.9876526153536342445, 7.798540720466730171E-17 ) ) ;
#5790=CARTESIAN_POINT ( 'NONE',  ( -84.23462711737164454, 33.01666666666666572, 30.00000000000000000 ) ) ;
#5792=EDGE_CURVE ( 'NONE', #16790, #8885, #12520, .T. ) ;
#5793=VECTOR ( 'NONE', #151, 1000.000000000000000 ) ;
#5795=ORIENTED_EDGE ( 'NONE', *, *, #8193, .F. ) ;
#5796=CIRCLE ( 'NONE', #13029, 1.500000000000000888 ) ;
#5797=CARTESIAN_POINT ( 'NONE',  ( -34.15575545585073058, -83.37298466334958391, 8.660254037844412167 ) ) ;
#5798=CARTESIAN_POINT ( 'NONE',  ( -57.89905323451571206, -29.43363984018462176, -8.660254037844380193 ) ) ;
#5799=DIRECTION ( 'NONE',  ( -0.1566598588826321192, 0.9876526153536342445, 7.798540720466731404E-17 ) ) ;
#5803=CARTESIAN_POINT ( 'NONE',  ( -55.42992169613162190, -29.04199019297804085, 4.330127018922217630 ) ) ;
#5804=VERTEX_POINT ( 'NONE', #14141 ) ;
#5805=VERTEX_POINT ( 'NONE', #5138 ) ;
#5807=CARTESIAN_POINT ( 'NONE',  ( -74.97862068226375243, -27.08026443497990954, 8.660254037844417496 ) ) ;
#5808=AXIS2_PLACEMENT_3D ( 'NONE', #9629, #5270, #11023 ) ;
#5809=FACE_OUTER_BOUND ( 'NONE', #16822, .T. ) ;
#5810=EDGE_CURVE ( 'NONE', #2328, #5513, #9653, .T. ) ;
#5811=CIRCLE ( 'NONE', #13953, 139.0000000000000000 ) ;
#5812=EDGE_CURVE ( 'NONE', #8478, #8527, #3883, .T. ) ;
#5813=FACE_OUTER_BOUND ( 'NONE', #13152, .T. ) ;
#5814=EDGE_CURVE ( 'NONE', #11180, #18706, #2373, .T. ) ;
#5815=AXIS2_PLACEMENT_3D ( 'NONE', #16633, #13671, #6315 ) ;
#5817=AXIS2_PLACEMENT_3D ( 'NONE', #10113, #11429, #9765 ) ;
#5818=CIRCLE ( 'NONE', #7338, 1.500000000000000888 ) ;
#5819=ORIENTED_EDGE ( 'NONE', *, *, #18681, .F. ) ;
#5820=DIRECTION ( 'NONE',  ( -0.9876526153536341335, -0.1566598588826327021, 0.000000000000000000 ) ) ;
#5821=CARTESIAN_POINT ( 'NONE',  ( -2.879979761448749009, -15.64409473654778893, 8.660254037844412167 ) ) ;
#5823=ORIENTED_EDGE ( 'NONE', *, *, #2752, .T. ) ;
#5824=FACE_BOUND ( 'NONE', #16901, .T. ) ;
#5825=DIRECTION ( 'NONE',  ( -0.1566598588826321192, 0.9876526153536342445, 7.798540720466731404E-17 ) ) ;
#5826=ORIENTED_EDGE ( 'NONE', *, *, #7331, .F. ) ;
#5827=EDGE_LOOP ( 'NONE', ( #2252, #13808, #14091, #6121 ) ) ;
#5828=VERTEX_POINT ( 'NONE', #2497 ) ;
#5830=ORIENTED_EDGE ( 'NONE', *, *, #18468, .F. ) ;
#5831=FACE_BOUND ( 'NONE', #12792, .T. ) ;
#5833=CARTESIAN_POINT ( 'NONE',  ( -36.62488699423481364, -83.76463431055616127, -12.99038105676658539 ) ) ;
#5834=EDGE_CURVE ( 'NONE', #12466, #3591, #14195, .T. ) ;
#5835=VERTEX_POINT ( 'NONE', #2579 ) ;
#5836=AXIS2_PLACEMENT_3D ( 'NONE', #12554, #16962, #18404 ) ;
#5839=DIRECTION ( 'NONE',  ( -0.1566598588826321192, 0.9876526153536342445, 7.798540720466731404E-17 ) ) ;
#5842=EDGE_LOOP ( 'NONE', ( #9662, #204, #14896, #3324 ) ) ;
#5843=CARTESIAN_POINT ( 'NONE',  ( -52.96079015774754595, -28.65034054577145994, 17.32050807568881723 ) ) ;
#5844=CARTESIAN_POINT ( 'NONE',  ( -15.88418207180859021, -80.47477727402089442, 1.424741226644455312E-14 ) ) ;
#5845=DIRECTION ( 'NONE',  ( 0.000000000000000000, 0.000000000000000000, 1.000000000000000000 ) ) ;
#5846=CIRCLE ( 'NONE', #10666, 2.000000000000000000 ) ;
#5847=AXIS2_PLACEMENT_3D ( 'NONE', #11003, #12330, #18176 ) ;
#5848=EDGE_LOOP ( 'NONE', ( #2668, #5823 ) ) ;
#5849=FACE_OUTER_BOUND ( 'NONE', #1668, .T. ) ;
#5850=DIRECTION ( 'NONE',  ( -0.1566598588826321192, 0.9876526153536342445, 7.798540720466731404E-17 ) ) ;
#5852=LINE ( 'NONE', #238, #17871 ) ;
#5854=ADVANCED_FACE ( 'NONE', ( #9592 ), #15369, .F. ) ;
#5855=EDGE_CURVE ( 'NONE', #1633, #10598, #2076, .T. ) ;
#5856=AXIS2_PLACEMENT_3D ( 'NONE', #7328, #15925, #7409 ) ;
#5857=CARTESIAN_POINT ( 'NONE',  ( 1.360103686702108128, -20.03404830722672259, 17.32050807568881012 ) ) ;
#5859=CARTESIAN_POINT ( 'NONE',  ( -3.373806069125576901, -15.72242466598909871, -4.330127018922183879 ) ) ;
#5860=VERTEX_POINT ( 'NONE', #12606 ) ;
#5861=FACE_OUTER_BOUND ( 'NONE', #14471, .T. ) ;
#5862=EDGE_CURVE ( 'NONE', #7429, #898, #13265, .T. ) ;
#5863=CARTESIAN_POINT ( 'NONE',  ( -18.39294862037050393, -23.16724548487935564, 17.32050807568881012 ) ) ;
#5864=ORIENTED_EDGE ( 'NONE', *, *, #7179, .F. ) ;
#5866=CARTESIAN_POINT ( 'NONE',  ( -36.62488699423482785, -83.76463431055616127, -21.65063509461098690 ) ) ;
#5867=ORIENTED_EDGE ( 'NONE', *, *, #6828, .F. ) ;
#5869=DIRECTION ( 'NONE',  ( -0.1566598588826321192, 0.9876526153536342445, 7.798540720466730171E-17 ) ) ;
#5870=CARTESIAN_POINT ( 'NONE',  ( -10.98555400521827607, -21.99229654325962002, 21.65063509461101177 ) ) ;
#5871=CARTESIAN_POINT ( 'NONE',  ( 9.300959619709004755, -76.47995087251376845, 21.65063509461100821 ) ) ;
#5873=DIRECTION ( 'NONE',  ( -0.1566598588826321747, 0.9876526153536343555, 0.000000000000000000 ) ) ;
#5875=DIRECTION ( 'NONE',  ( -0.1566598588826321747, 0.9876526153536343555, 0.000000000000000000 ) ) ;
#5877=ORIENTED_EDGE ( 'NONE', *, *, #15746, .T. ) ;
#5881=VERTEX_POINT ( 'NONE', #11060 ) ;
#5882=ORIENTED_EDGE ( 'NONE', *, *, #16890, .F. ) ;
#5883=CARTESIAN_POINT ( 'NONE',  ( -73.70149508017377116, -31.94019758230671258, -12.99038105676658006 ) ) ;
#5884=VERTEX_POINT ( 'NONE', #13602 ) ;
#5885=EDGE_CURVE ( 'NONE', #17245, #1063, #11144, .T. ) ;
#5886=VERTEX_POINT ( 'NONE', #2326 ) ;
#5888=FACE_BOUND ( 'NONE', #16738, .T. ) ;
#5890=CARTESIAN_POINT ( 'NONE',  ( -77.65210554158829837, -32.56683701783724416, 17.32050807568881723 ) ) ;
#5893=VERTEX_POINT ( 'NONE', #9250 ) ;
#5895=ADVANCED_FACE ( 'NONE', ( #12262 ), #5066, .F. ) ;
#5896=DIRECTION ( 'NONE',  ( -0.1566598588826321192, 0.9876526153536342445, 7.798540720466731404E-17 ) ) ;
#5897=CYLINDRICAL_SURFACE ( 'NONE', #6389, 1.500000000000000666 ) ;
#5898=CARTESIAN_POINT ( 'NONE',  ( -51.43967622453925514, -86.11453219379563961, 21.65063509461101532 ) ) ;
#5899=DIRECTION ( 'NONE',  ( -0.9876526153536336894, -0.1566598588826349503, 0.000000000000000000 ) ) ;
#5900=ADVANCED_FACE ( 'NONE', ( #2150 ), #2236, .F. ) ;
#5901=ORIENTED_EDGE ( 'NONE', *, *, #18359, .T. ) ;
#5902=EDGE_CURVE ( 'NONE', #17941, #6457, #18730, .T. ) ;
#5904=ORIENTED_EDGE ( 'NONE', *, *, #8475, .T. ) ;
#5905=CARTESIAN_POINT ( 'NONE',  ( -52.75643683680709728, -23.55541761012068847, -12.99038105676658006 ) ) ;
#5907=AXIS2_PLACEMENT_3D ( 'NONE', #4122, #8409, #2270 ) ;
#5909=CARTESIAN_POINT ( 'NONE',  ( -15.22563745336913144, -17.60234297258069347, 12.99038105676661381 ) ) ;
#5912=DIRECTION ( 'NONE',  ( -0.1566598588826321747, 0.9876526153536343555, 0.000000000000000000 ) ) ;
#5913=CIRCLE ( 'NONE', #8344, 1.500000000000000888 ) ;
#5915=EDGE_CURVE ( 'NONE', #10816, #8368, #5676, .T. ) ;
#5919=CARTESIAN_POINT ( 'NONE',  ( -58.84707083969148300, -87.28948113541537168, 17.32050807568881368 ) ) ;
#5920=ORIENTED_EDGE ( 'NONE', *, *, #1675, .T. ) ;
#5921=ORIENTED_EDGE ( 'NONE', *, *, #13337, .F. ) ;
#5922=DIRECTION ( 'NONE',  ( -0.1566598588826321192, 0.9876526153536342445, 7.798540720466730171E-17 ) ) ;
#5923=EDGE_CURVE ( 'NONE', #5152, #7813, #10490, .T. ) ;
#5924=ORIENTED_EDGE ( 'NONE', *, *, #13427, .F. ) ;
#5925=CARTESIAN_POINT ( 'NONE',  ( -21.81009776393036503, -81.41473642731668292, -12.99038105676658539 ) ) ;
#5927=ORIENTED_EDGE ( 'NONE', *, *, #3668, .T. ) ;
#5928=CYLINDRICAL_SURFACE ( 'NONE', #7012, 1.500000000000001554 ) ;
#5929=AXIS2_PLACEMENT_3D ( 'NONE', #9594, #2498, #15370 ) ;
#5930=FACE_BOUND ( 'NONE', #16575, .T. ) ;
#5931=CARTESIAN_POINT ( 'NONE',  ( -30.53425299135042081, -20.03057078526147450, -17.32050807568878170 ) ) ;
#5932=DIRECTION ( 'NONE',  ( -0.9876526153536341335, -0.1566598588826327021, 0.000000000000000000 ) ) ;
#5933=AXIS2_PLACEMENT_3D ( 'NONE', #5017, #13030, #15552 ) ;
#5934=DIRECTION ( 'NONE',  ( -0.9876526153536336894, -0.1566598588826349503, 0.000000000000000000 ) ) ;
#5935=CARTESIAN_POINT ( 'NONE',  ( -52.75643683680706886, -23.55541761012070268, 21.65063509461101887 ) ) ;
#5936=DIRECTION ( 'NONE',  ( -0.1566598588826321192, 0.9876526153536342445, 7.798540720466730171E-17 ) ) ;
#5938=CARTESIAN_POINT ( 'NONE',  ( -54.89646037827696290, -86.66284169988483654, -4.330127018922185655 ) ) ;
#5941=EDGE_LOOP ( 'NONE', ( #11044, #1177, #11845, #1125 ) ) ;
#5942=CARTESIAN_POINT ( 'NONE',  ( -9.997901389864651378, -21.83563668437698269, 1.522258424776792809E-14 ) ) ;
#5943=LINE ( 'NONE', #17352, #16359 ) ;
#5944=EDGE_LOOP ( 'NONE', ( #5683, #12415 ) ) ;
#5945=EDGE_CURVE ( 'NONE', #15653, #8283, #4105, .T. ) ;
#5946=EDGE_CURVE ( 'NONE', #16090, #13071, #12692, .T. ) ;
#5947=CIRCLE ( 'NONE', #2299, 1.500000000000000888 ) ;
#5948=CARTESIAN_POINT ( 'NONE',  ( -24.27922930231443743, -81.80638607452327449, 8.660254037844412167 ) ) ;
#5949=CARTESIAN_POINT ( 'NONE',  ( -45.01993422474063777, -85.09624311105854133, 21.65063509461101532 ) ) ;
#5952=AXIS2_PLACEMENT_3D ( 'NONE', #11509, #10185, #14466 ) ;
#5953=DIRECTION ( 'NONE',  ( -0.9876526153536336894, -0.1566598588826349503, 0.000000000000000000 ) ) ;
#5954=DIRECTION ( 'NONE',  ( -0.9876526153536341335, -0.1566598588826327576, 0.000000000000000000 ) ) ;
#5955=CYLINDRICAL_SURFACE ( 'NONE', #18782, 1.500000000000001554 ) ;
#5956=ORIENTED_EDGE ( 'NONE', *, *, #14218, .F. ) ;
#5958=AXIS2_PLACEMENT_3D ( 'NONE', #3166, #1406, #13129 ) ;
#5959=PLANE ( 'NONE',  #12012 ) ;
#5961=AXIS2_PLACEMENT_3D ( 'NONE', #17000, #1169, #6949 ) ;
#5964=CIRCLE ( 'NONE', #4735, 1.500000000000000444 ) ;
#5965=ORIENTED_EDGE ( 'NONE', *, *, #4469, .T. ) ;
#5966=ADVANCED_FACE ( 'NONE', ( #13435 ), #475, .F. ) ;
#5970=DIRECTION ( 'NONE',  ( -0.1566598588826321192, 0.9876526153536342445, 7.798540720466731404E-17 ) ) ;
#5971=VECTOR ( 'NONE', #7385, 1000.000000000000000 ) ;
#5973=ORIENTED_EDGE ( 'NONE', *, *, #4649, .F. ) ;
#5974=VECTOR ( 'NONE', #2876, 1000.000000000000000 ) ;
#5975=EDGE_CURVE ( 'NONE', #12855, #1506, #8037, .T. ) ;
#5976=DIRECTION ( 'NONE',  ( -0.1566598588826321192, 0.9876526153536342445, 7.798540720466731404E-17 ) ) ;
#5977=ORIENTED_EDGE ( 'NONE', *, *, #4671, .F. ) ;
#5978=DIRECTION ( 'NONE',  ( -0.1566598588826321192, 0.9876526153536342445, 7.798540720466730171E-17 ) ) ;
#5979=ORIENTED_EDGE ( 'NONE', *, *, #18052, .T. ) ;
#5980=FACE_BOUND ( 'NONE', #10720, .T. ) ;
#5981=AXIS2_PLACEMENT_3D ( 'NONE', #1005, #7991, #10811 ) ;
#5982=DIRECTION ( 'NONE',  ( -0.1566598588826321192, 0.9876526153536342445, 7.798540720466730171E-17 ) ) ;
#5983=VERTEX_POINT ( 'NONE', #12808 ) ;
#5984=DIRECTION ( 'NONE',  ( -0.1566598588826321192, 0.9876526153536342445, 7.798540720466730171E-17 ) ) ;
#5985=CARTESIAN_POINT ( 'NONE',  ( -64.60826822105063627, -25.43533591671226901, -21.65063509461098334 ) ) ;
#5986=LINE ( 'NONE', #16316, #16014 ) ;
#5987=ORIENTED_EDGE ( 'NONE', *, *, #18316, .T. ) ;
#5989=ORIENTED_EDGE ( 'NONE', *, *, #4578, .T. ) ;
#5991=FACE_OUTER_BOUND ( 'NONE', #13739, .T. ) ;
#5992=CARTESIAN_POINT ( 'NONE',  ( -64.77298653181324539, -88.22944028871116018, 12.99038105676661203 ) ) ;
#5993=AXIS2_PLACEMENT_3D ( 'NONE', #1902, #9384, #6468 ) ;
#5994=CARTESIAN_POINT ( 'NONE',  ( -76.95392591297100182, -27.39358415274517355, 1.926565525561698076E-14 ) ) ;
#5996=EDGE_CURVE ( 'NONE', #13102, #4754, #18650, .T. ) ;
#5998=AXIS2_PLACEMENT_3D ( 'NONE', #1692, #10312, #3106 ) ;
#5999=ORIENTED_EDGE ( 'NONE', *, *, #4861, .T. ) ;
#6000=EDGE_CURVE ( 'NONE', #12139, #17674, #5329, .T. ) ;
#6001=CIRCLE ( 'NONE', #1764, 1.500000000000000444 ) ;
#6002=AXIS2_PLACEMENT_3D ( 'NONE', #18485, #4006, #9809 ) ;
#6005=AXIS2_PLACEMENT_3D ( 'NONE', #3371, #1778, #369 ) ;
#6006=CARTESIAN_POINT ( 'NONE',  ( -4.361458684479201153, -15.87908452487173427, 1.561251128379126385E-14 ) ) ;
#6008=CARTESIAN_POINT ( 'NONE',  ( -74.48479437458692587, -27.00193450553859265, -4.330127018922180326 ) ) ;
#6010=EDGE_LOOP ( 'NONE', ( #5147, #930, #10423, #2143 ) ) ;
#6011=FACE_BOUND ( 'NONE', #12768, .T. ) ;
#6012=DIRECTION ( 'NONE',  ( -0.1566598588826321747, 0.9876526153536343555, 0.000000000000000000 ) ) ;
#6013=CARTESIAN_POINT ( 'NONE',  ( -75.96627329761737712, -27.23692429386254688, 21.65063509461102242 ) ) ;
#6014=CYLINDRICAL_SURFACE ( 'NONE', #18749, 1.500000000000001554 ) ;
#6016=CIRCLE ( 'NONE', #260, 1.500000000000000000 ) ;
#6017=VERTEX_POINT ( 'NONE', #11370 ) ;
#6019=DIRECTION ( 'NONE',  ( 0.000000000000000000, 0.000000000000000000, 1.000000000000000000 ) ) ;
#6020=CARTESIAN_POINT ( 'NONE',  ( -2.096680467035594297, -20.58235781331593017, 8.660254037844412167 ) ) ;
#6021=VECTOR ( 'NONE', #6445, 1000.000000000000000 ) ;
#6022=AXIS2_PLACEMENT_3D ( 'NONE', #10945, #3646, #13496 ) ;
#6023=EDGE_CURVE ( 'NONE', #14160, #311, #18691, .T. ) ;
#6024=CARTESIAN_POINT ( 'NONE',  ( -40.61513246582718040, -26.69209230973856251, 12.99038105676661736 ) ) ;
#6025=EDGE_CURVE ( 'NONE', #202, #1113, #785, .T. ) ;
#6026=CYLINDRICAL_SURFACE ( 'NONE', #11465, 1.500000000000001554 ) ;
#6027=DIRECTION ( 'NONE',  ( 0.000000000000000000, 0.000000000000000000, 1.000000000000000000 ) ) ;
#6030=CYLINDRICAL_SURFACE ( 'NONE', #5113, 1.500000000000001554 ) ;
#6033=AXIS2_PLACEMENT_3D ( 'NONE', #12933, #3082, #243 ) ;
#6034=LINE ( 'NONE', #160, #17796 ) ;
#6035=ORIENTED_EDGE ( 'NONE', *, *, #2994, .T. ) ;
#6036=EDGE_LOOP ( 'NONE', ( #13311, #7927, #850, #10639 ) ) ;
#6037=DIRECTION ( 'NONE',  ( -0.1566598588826321192, 0.9876526153536342445, 7.798540720466731404E-17 ) ) ;
#6039=VECTOR ( 'NONE', #18699, 1000.000000000000000 ) ;
#6040=VERTEX_POINT ( 'NONE', #15471 ) ;
#6041=ORIENTED_EDGE ( 'NONE', *, *, #9746, .F. ) ;
#6042=ORIENTED_EDGE ( 'NONE', *, *, #14752, .T. ) ;
#6043=CIRCLE ( 'NONE', #17866, 1.500000000000000888 ) ;
#6044=AXIS2_PLACEMENT_3D ( 'NONE', #2710, #9745, #15512 ) ;
#6045=ORIENTED_EDGE ( 'NONE', *, *, #5490, .F. ) ;
#6046=CIRCLE ( 'NONE', #6, 1.500000000000000444 ) ;
#6048=EDGE_CURVE ( 'NONE', #6912, #11183, #2493, .T. ) ;
#6049=AXIS2_PLACEMENT_3D ( 'NONE', #9619, #15293, #12454 ) ;
#6050=ADVANCED_FACE ( 'NONE', ( #8359 ), #14137, .F. ) ;
#6051=FACE_OUTER_BOUND ( 'NONE', #7379, .T. ) ;
#6052=DIRECTION ( 'NONE',  ( -0.9876526153536336894, -0.1566598588826349503, 0.000000000000000000 ) ) ;
#6053=CIRCLE ( 'NONE', #7862, 144.0000000000000284 ) ;
#6054=AXIS2_PLACEMENT_3D ( 'NONE', #9154, #14925, #1102 ) ;
#6055=FACE_OUTER_BOUND ( 'NONE', #4037, .T. ) ;
#6061=DIRECTION ( 'NONE',  ( -0.1566598588826321192, 0.9876526153536342445, 7.798540720466731404E-17 ) ) ;
#6062=ADVANCED_FACE ( 'NONE', ( #10973 ), #12200, .F. ) ;
#6064=CARTESIAN_POINT ( 'NONE',  ( -60.36818477289978091, -29.82528948739120267, 4.330127018922217630 ) ) ;
#6065=CIRCLE ( 'NONE', #16665, 1.499999999999999556 ) ;
#6068=AXIS2_PLACEMENT_3D ( 'NONE', #15866, #7432, #17218 ) ;
#6069=VERTEX_POINT ( 'NONE', #13922 ) ;
#6070=CARTESIAN_POINT ( 'NONE',  ( -60.36818477289977380, -29.82528948739119556, 12.99038105676661736 ) ) ;
#6071=CIRCLE ( 'NONE', #11479, 1.500000000000000888 ) ;
#6072=ORIENTED_EDGE ( 'NONE', *, *, #13305, .T. ) ;
#6075=FACE_OUTER_BOUND ( 'NONE', #9010, .T. ) ;
#6076=CIRCLE ( 'NONE', #16986, 1.500000000000000888 ) ;
#6077=DIRECTION ( 'NONE',  ( -0.1566598588826321192, 0.9876526153536342445, 7.798540720466730171E-17 ) ) ;
#6079=ORIENTED_EDGE ( 'NONE', *, *, #2240, .F. ) ;
#6080=UNCERTAINTY_MEASURE_WITH_UNIT (LENGTH_MEASURE( 1.000000000000000082E-05 ), #10952, 'distance_accuracy_value', 'NONE');
#6081=AXIS2_PLACEMENT_3D ( 'NONE', #6569, #12316, #11462 ) ;
#6082=DIRECTION ( 'NONE',  ( -0.1566598588826321192, 0.9876526153536342445, 7.798540720466730171E-17 ) ) ;
#6083=LINE ( 'NONE', #1808, #4791 ) ;
#6084=VECTOR ( 'NONE', #7097, 1000.000000000000000 ) ;
#6085=EDGE_LOOP ( 'NONE', ( #17561, #205, #17107, #17075 ) ) ;
#6086=ADVANCED_FACE ( 'NONE', ( #868 ), #6646, .F. ) ;
#6089=CARTESIAN_POINT ( 'NONE',  ( -10.28737437660097775, -16.81904367816753165, 4.330127018922214965 ) ) ;
#6091=CARTESIAN_POINT ( 'NONE',  ( -53.94844277310118486, -28.80700040465408662, -21.65063509461098334 ) ) ;
#6092=CARTESIAN_POINT ( 'NONE',  ( -43.08426400421124924, -27.08374195694514341, 17.32050807568881723 ) ) ;
#6094=ORIENTED_EDGE ( 'NONE', *, *, #10580, .T. ) ;
#6095=AXIS2_PLACEMENT_3D ( 'NONE', #17808, #9240, #12164 ) ;
#6096=EDGE_LOOP ( 'NONE', ( #15238, #8034 ) ) ;
#6097=VERTEX_POINT ( 'NONE', #18434 ) ;
#6100=FACE_BOUND ( 'NONE', #6538, .T. ) ;
#6101=CARTESIAN_POINT ( 'NONE',  ( -26.58364252993588650, -19.40393134973095712, 4.330127018922218518 ) ) ;
#6102=VERTEX_POINT ( 'NONE', #3673 ) ;
#6103=DIRECTION ( 'NONE',  ( -0.9876526153536341335, 0.1566598588826326743, -0.000000000000000000 ) ) ;
#6104=ORIENTED_EDGE ( 'NONE', *, *, #3981, .F. ) ;
#6105=AXIS2_PLACEMENT_3D ( 'NONE', #16982, #1062, #4987 ) ;
#6106=VERTEX_POINT ( 'NONE', #2257 ) ;
#6107=CARTESIAN_POINT ( 'NONE',  ( -45.34904222165485521, -22.38046866850095995, 8.660254037844417496 ) ) ;
#6108=AXIS2_PLACEMENT_3D ( 'NONE', #9100, #3296, #10509 ) ;
#6109=DIRECTION ( 'NONE',  ( -0.1566598588826321192, 0.9876526153536342445, 7.798540720466730171E-17 ) ) ;
#6110=DIRECTION ( 'NONE',  ( -0.9876526153536341335, -0.1566598588826327021, 0.000000000000000000 ) ) ;
#6112=ORIENTED_EDGE ( 'NONE', *, *, #1558, .F. ) ;
#6115=ADVANCED_FACE ( 'NONE', ( #13807 ), #10967, .F. ) ;
#6116=DIRECTION ( 'NONE',  ( -0.1566598588826321747, 0.9876526153536343555, 0.000000000000000000 ) ) ;
#6117=CYLINDRICAL_SURFACE ( 'NONE', #854, 1.500000000000000666 ) ;
#6118=CIRCLE ( 'NONE', #10932, 1.500000000000000888 ) ;
#6119=ORIENTED_EDGE ( 'NONE', *, *, #6782, .F. ) ;
#6121=ORIENTED_EDGE ( 'NONE', *, *, #12171, .T. ) ;
#6122=ORIENTED_EDGE ( 'NONE', *, *, #8442, .T. ) ;
#6123=FACE_OUTER_BOUND ( 'NONE', #18489, .T. ) ;
#6124=EDGE_CURVE ( 'NONE', #16410, #3635, #2281, .T. ) ;
#6125=EDGE_LOOP ( 'NONE', ( #750, #15116 ) ) ;
#6126=CARTESIAN_POINT ( 'NONE',  ( -71.72618984946653597, -31.62687786454144856, 12.99038105676661736 ) ) ;
#6128=AXIS2_PLACEMENT_3D ( 'NONE', #390, #4545, #10325 ) ;
#6130=FACE_OUTER_BOUND ( 'NONE', #14136, .T. ) ;
#6131=CARTESIAN_POINT ( 'NONE',  ( -51.27495791377663181, -23.32042782179674845, 4.330127018922218518 ) ) ;
#6133=EDGE_LOOP ( 'NONE', ( #11769, #14281 ) ) ;
#6135=DIRECTION ( 'NONE',  ( -0.1566598588826321192, 0.9876526153536342445, 7.798540720466730171E-17 ) ) ;
#6136=DIRECTION ( 'NONE',  ( -0.1566598588826321747, 0.9876526153536343555, 0.000000000000000000 ) ) ;
#6137=DIRECTION ( 'NONE',  ( -0.1566598588826321192, 0.9876526153536342445, 7.798540720466731404E-17 ) ) ;
#6138=FACE_OUTER_BOUND ( 'NONE', #14308, .T. ) ;
#6141=CARTESIAN_POINT ( 'NONE',  ( -11.93357161039406300, -79.84813783849037350, -4.330127018922185655 ) ) ;
#6142=ORIENTED_EDGE ( 'NONE', *, *, #2556, .F. ) ;
#6143=ORIENTED_EDGE ( 'NONE', *, *, #5295, .F. ) ;
#6145=EDGE_CURVE ( 'NONE', #1703, #14341, #7686, .T. ) ;
#6146=ORIENTED_EDGE ( 'NONE', *, *, #653, .T. ) ;
#6147=ADVANCED_FACE ( 'NONE', ( #3734 ), #15410, .F. ) ;
#6148=EDGE_LOOP ( 'NONE', ( #7609, #18297, #6266, #4604 ) ) ;
#6149=FACE_OUTER_BOUND ( 'NONE', #880, .T. ) ;
#6151=ORIENTED_EDGE ( 'NONE', *, *, #12161, .F. ) ;
#6152=DIRECTION ( 'NONE',  ( -0.000000000000000000, -0.000000000000000000, -1.000000000000000000 ) ) ;
#6153=CIRCLE ( 'NONE', #4632, 1.500000000000000888 ) ;
#6154=CYLINDRICAL_SURFACE ( 'NONE', #16157, 1.500000000000001554 ) ;
#6157=CARTESIAN_POINT ( 'NONE',  ( -23.29157668696081629, -81.64972621564065491, 12.99038105676661203 ) ) ;
#6159=CARTESIAN_POINT ( 'NONE',  ( -34.19539046602859145, -25.67380322700145356, -21.65063509461098334 ) ) ;
#6160=FACE_BOUND ( 'NONE', #11941, .T. ) ;
#6161=DIRECTION ( 'NONE',  ( -0.1566598588826321747, 0.9876526153536343555, 0.000000000000000000 ) ) ;
#6162=EDGE_LOOP ( 'NONE', ( #9317, #1454 ) ) ;
#6163=DIRECTION ( 'NONE',  ( -0.9876526153536341335, -0.1566598588826327021, 0.000000000000000000 ) ) ;
#6164=EDGE_CURVE ( 'NONE', #10299, #8719, #7159, .T. ) ;
#6166=ORIENTED_EDGE ( 'NONE', *, *, #7425, .T. ) ;
#6167=ADVANCED_FACE ( 'NONE', ( #11029 ), #1040, .F. ) ;
#6169=CARTESIAN_POINT ( 'NONE',  ( -16.91146969734005268, -22.93225569655540141, 1.887572821959364500E-14 ) ) ;
#6170=AXIS2_PLACEMENT_3D ( 'NONE', #13806, #15338, #6639 ) ;
#6171=CARTESIAN_POINT ( 'NONE',  ( -44.03228160938703439, -84.93958325217590755, 1.424741226644455312E-14 ) ) ;
#6173=EDGE_LOOP ( 'NONE', ( #8847, #14361 ) ) ;
#6174=DIRECTION ( 'NONE',  ( -0.1566598588826321192, 0.9876526153536342445, 7.798540720466730171E-17 ) ) ;
#6175=CARTESIAN_POINT ( 'NONE',  ( -65.30644784966793281, -30.60858878180435738, 4.330127018922217630 ) ) ;
#6176=VERTEX_POINT ( 'NONE', #13884 ) ;
#6177=DIRECTION ( 'NONE',  ( -0.1566598588826321747, 0.9876526153536343555, 0.000000000000000000 ) ) ;
#6178=DIRECTION ( 'NONE',  ( -0.1566598588826321192, 0.9876526153536342445, 7.798540720466730171E-17 ) ) ;
#6179=AXIS2_PLACEMENT_3D ( 'NONE', #9349, #18103, #15135 ) ;
#6180=CARTESIAN_POINT ( 'NONE',  ( 55.85952145814821534, 6.938893903907228378E-15, 30.00000000000000000 ) ) ;
#6182=EDGE_LOOP ( 'NONE', ( #161, #9941, #1560, #3972 ) ) ;
#6185=DIRECTION ( 'NONE',  ( -0.1566598588826321192, 0.9876526153536342445, 7.798540720466731404E-17 ) ) ;
#6186=LINE ( 'NONE', #13368, #3585 ) ;
#6187=ORIENTED_EDGE ( 'NONE', *, *, #2134, .T. ) ;
#6188=VERTEX_POINT ( 'NONE', #16856 ) ;
#6189=ORIENTED_EDGE ( 'NONE', *, *, #11337, .F. ) ;
#6190=CYLINDRICAL_SURFACE ( 'NONE', #3499, 1.500000000000001554 ) ;
#6191=ORIENTED_EDGE ( 'NONE', *, *, #12476, .T. ) ;
#6192=VERTEX_POINT ( 'NONE', #14444 ) ;
#6193=EDGE_CURVE ( 'NONE', #7789, #9740, #4202, .T. ) ;
#6194=VERTEX_POINT ( 'NONE', #18757 ) ;
#6195=FACE_BOUND ( 'NONE', #133, .T. ) ;
#6199=DIRECTION ( 'NONE',  ( 0.000000000000000000, 0.000000000000000000, 1.000000000000000000 ) ) ;
#6200=EDGE_LOOP ( 'NONE', ( #10866, #1705 ) ) ;
#6202=ORIENTED_EDGE ( 'NONE', *, *, #9856, .T. ) ;
#6203=ORIENTED_EDGE ( 'NONE', *, *, #14100, .T. ) ;
#6204=DIRECTION ( 'NONE',  ( -0.1566598588826321192, 0.9876526153536342445, 7.798540720466730171E-17 ) ) ;
#6205=DIRECTION ( 'NONE',  ( -0.9876526153536341335, -0.1566598588826327021, 0.000000000000000000 ) ) ;
#6208=DIRECTION ( 'NONE',  ( -0.9876526153536341335, -0.1566598588826327021, 0.000000000000000000 ) ) ;
#6210=ORIENTED_EDGE ( 'NONE', *, *, #10296, .T. ) ;
#6212=AXIS2_PLACEMENT_3D ( 'NONE', #17469, #4074, #7063 ) ;
#6214=CYLINDRICAL_SURFACE ( 'NONE', #5380, 1.500000000000001554 ) ;
#6215=ORIENTED_EDGE ( 'NONE', *, *, #3022, .T. ) ;
#6216=ORIENTED_EDGE ( 'NONE', *, *, #8355, .F. ) ;
#6217=DIRECTION ( 'NONE',  ( -0.9876526153536341335, -0.1566598588826327021, 0.000000000000000000 ) ) ;
#6219=CARTESIAN_POINT ( 'NONE',  ( -37.15834831208948685, -26.14378280364935137, -12.99038105676658006 ) ) ;
#6220=EDGE_CURVE ( 'NONE', #7195, #13436, #1401, .T. ) ;
#6221=LINE ( 'NONE', #11949, #1800 ) ;
#6222=CARTESIAN_POINT ( 'NONE',  ( -40.57549745564934085, -84.39127374608668219, -8.660254037844385522 ) ) ;
#6223=CYLINDRICAL_SURFACE ( 'NONE', #15440, 1.500000000000001554 ) ;
#6224=FACE_OUTER_BOUND ( 'NONE', #688, .T. ) ;
#6226=LINE ( 'NONE', #437, #15588 ) ;
#6227=ORIENTED_EDGE ( 'NONE', *, *, #704, .T. ) ;
#6228=ORIENTED_EDGE ( 'NONE', *, *, #11365, .F. ) ;
#6229=CARTESIAN_POINT ( 'NONE',  ( -15.39035576413176187, -80.39644734457957043, -12.99038105676658539 ) ) ;
#6230=EDGE_LOOP ( 'NONE', ( #17355, #6757, #16475, #17090 ) ) ;
#6231=EDGE_LOOP ( 'NONE', ( #12143, #18498 ) ) ;
#6232=DIRECTION ( 'NONE',  ( 0.9876526153536341335, -0.1566598588826326743, 3.168663947239273463E-17 ) ) ;
#6233=CARTESIAN_POINT ( 'NONE',  ( -9.299721761247353058, -16.66238381928489787, -17.32050807568878170 ) ) ;
#6235=ORIENTED_EDGE ( 'NONE', *, *, #598, .F. ) ;
#6237=LINE ( 'NONE', #14850, #15170 ) ;
#6239=EDGE_CURVE ( 'NONE', #3635, #16410, #16217, .T. ) ;
#6240=CARTESIAN_POINT ( 'NONE',  ( 7.819480696678551723, -76.71494066083772623, -4.330127018922189208 ) ) ;
#6241=CARTESIAN_POINT ( 'NONE',  ( -57.20087360589841552, -24.26038697509254050, 1.926565525561698076E-14 ) ) ;
#6242=CARTESIAN_POINT ( 'NONE',  ( -40.61513246582718750, -26.69209230973856251, -12.99038105676658006 ) ) ;
#6244=DIRECTION ( 'NONE',  ( -0.1566598588826321192, 0.9876526153536342445, 7.798540720466730171E-17 ) ) ;
#6245=AXIS2_PLACEMENT_3D ( 'NONE', #12082, #10755, #13420 ) ;
#6247=DIRECTION ( 'NONE',  ( -0.1566598588826321747, 0.9876526153536343555, 0.000000000000000000 ) ) ;
#6248=FACE_BOUND ( 'NONE', #1755, .T. ) ;
#6249=EDGE_CURVE ( 'NONE', #11583, #6259, #17733, .T. ) ;
#6250=DIRECTION ( 'NONE',  ( 0.000000000000000000, 0.000000000000000000, 1.000000000000000000 ) ) ;
#6252=CARTESIAN_POINT ( 'NONE',  ( -53.90880776292333820, -86.50618184100220276, -17.32050807568878525 ) ) ;
#6253=EDGE_LOOP ( 'NONE', ( #2810, #2206 ) ) ;
#6256=AXIS2_PLACEMENT_3D ( 'NONE', #5325, #14125, #1472 ) ;
#6257=ORIENTED_EDGE ( 'NONE', *, *, #11692, .T. ) ;
#6258=ORIENTED_EDGE ( 'NONE', *, *, #4649, .T. ) ;
#6259=VERTEX_POINT ( 'NONE', #13829 ) ;
#6262=VECTOR ( 'NONE', #6816, 1000.000000000000000 ) ;
#6263=DIRECTION ( 'NONE',  ( -0.1566598588826321192, 0.9876526153536342445, 7.798540720466730171E-17 ) ) ;
#6264=ADVANCED_FACE ( 'NONE', ( #14118 ), #14327, .F. ) ;
#6265=DIRECTION ( 'NONE',  ( -0.9876526153536341335, -0.1566598588826327021, 0.000000000000000000 ) ) ;
#6266=ORIENTED_EDGE ( 'NONE', *, *, #8837, .T. ) ;
#6267=DIRECTION ( 'NONE',  ( -0.1566598588826321192, 0.9876526153536342445, 7.798540720466731404E-17 ) ) ;
#6268=DIRECTION ( 'NONE',  ( -0.9876526153536336894, -0.1566598588826349503, 0.000000000000000000 ) ) ;
#6269=EDGE_CURVE ( 'NONE', #5835, #1839, #10130, .T. ) ;
#6272=CARTESIAN_POINT ( 'NONE',  ( 3.231158466157545206, -19.73726462726228092, -30.00000000000000000 ) ) ;
#6274=DIRECTION ( 'NONE',  ( -0.1566598588826321192, 0.9876526153536342445, 7.798540720466730171E-17 ) ) ;
#6275=ORIENTED_EDGE ( 'NONE', *, *, #16312, .T. ) ;
#6276=EDGE_CURVE ( 'NONE', #7482, #14323, #7787, .T. ) ;
#6277=CARTESIAN_POINT ( 'NONE',  ( -75.96627329761737712, -27.23692429386252911, -21.65063509461097979 ) ) ;
#6278=ORIENTED_EDGE ( 'NONE', *, *, #662, .T. ) ;
#6279=DIRECTION ( 'NONE',  ( -0.1566598588826321192, 0.9876526153536342445, 7.798540720466730171E-17 ) ) ;
#6280=AXIS2_PLACEMENT_3D ( 'NONE', #2414, #13973, #15294 ) ;
#6282=AXIS2_PLACEMENT_3D ( 'NONE', #13022, #10169, #5845 ) ;
#6284=EDGE_LOOP ( 'NONE', ( #4377, #6258 ) ) ;
#6285=AXIS2_PLACEMENT_3D ( 'NONE', #14666, #16380, #13413 ) ;
#6286=EDGE_LOOP ( 'NONE', ( #17721, #6971 ) ) ;
#6287=EDGE_LOOP ( 'NONE', ( #7436, #5026, #18206, #10647 ) ) ;
#6289=DIRECTION ( 'NONE',  ( -0.1566598588826321192, 0.9876526153536342445, 7.798540720466730171E-17 ) ) ;
#6292=FACE_BOUND ( 'NONE', #18522, .T. ) ;
#6293=DIRECTION ( 'NONE',  ( -0.1566598588826321192, 0.9876526153536342445, 7.798540720466731404E-17 ) ) ;
#6294=AXIS2_PLACEMENT_3D ( 'NONE', #8752, #1569, #7357 ) ;
#6297=EDGE_LOOP ( 'NONE', ( #18793, #15354 ) ) ;
#6298=FACE_BOUND ( 'NONE', #10316, .T. ) ;
#6299=CIRCLE ( 'NONE', #540, 1.500000000000000888 ) ;
#6300=CYLINDRICAL_SURFACE ( 'NONE', #1824, 1.500000000000001554 ) ;
#6301=CARTESIAN_POINT ( 'NONE',  ( -2.000000000000000000, 0.000000000000000000, 30.00000000000000000 ) ) ;
#6302=EDGE_CURVE ( 'NONE', #13704, #5893, #11655, .T. ) ;
#6304=DIRECTION ( 'NONE',  ( -0.9876526153536336894, -0.1566598588826349503, 0.000000000000000000 ) ) ;
#6305=CYLINDRICAL_SURFACE ( 'NONE', #8379, 1.500000000000001554 ) ;
#6310=ORIENTED_EDGE ( 'NONE', *, *, #3098, .T. ) ;
#6312=AXIS2_PLACEMENT_3D ( 'NONE', #8046, #11063, #864 ) ;
#6313=DIRECTION ( 'NONE',  ( -0.1566598588826321192, 0.9876526153536342445, 7.798540720466730171E-17 ) ) ;
#6314=ORIENTED_EDGE ( 'NONE', *, *, #17862, .T. ) ;
#6315=DIRECTION ( 'NONE',  ( -0.9876526153536341335, -0.1566598588826327021, 0.000000000000000000 ) ) ;
#6316=ORIENTED_EDGE ( 'NONE', *, *, #8069, .F. ) ;
#6317=VECTOR ( 'NONE', #16282, 1000.000000000000000 ) ;
#6318=DIRECTION ( 'NONE',  ( -0.9876526153536341335, -0.1566598588826327021, 0.000000000000000000 ) ) ;
#6319=AXIS2_PLACEMENT_3D ( 'NONE', #14878, #3206, #4094 ) ;
#6320=CYLINDRICAL_SURFACE ( 'NONE', #9061, 20.00000000000001066 ) ;
#6321=DIRECTION ( 'NONE',  ( -0.9876526153536341335, -0.1566598588826327021, 0.000000000000000000 ) ) ;
#6322=COLOUR_RGB ( '', 0.31764706, 0.68627451, 0.89019608) ;
#6323=ORIENTED_EDGE ( 'NONE', *, *, #15525, .F. ) ;
#6324=DIRECTION ( 'NONE',  ( -0.1566598588826321192, 0.9876526153536342445, 7.798540720466731404E-17 ) ) ;
#6325=CARTESIAN_POINT ( 'NONE',  ( -25.80034323552273179, -24.34219442649909126, 4.330127018922217630 ) ) ;
#6326=EDGE_CURVE ( 'NONE', #7929, #11102, #183, .T. ) ;
#6327=CARTESIAN_POINT ( 'NONE',  ( -26.74836084069850983, -82.19803572172985184, -12.99038105676658539 ) ) ;
#6328=ORIENTED_EDGE ( 'NONE', *, *, #5128, .T. ) ;
#6329=CYLINDRICAL_SURFACE ( 'NONE', #6095, 1.500000000000001554 ) ;
#6330=ADVANCED_FACE ( 'NONE', ( #13652 ), #695, .F. ) ;
#6331=CIRCLE ( 'NONE', #16931, 1.500000000000000888 ) ;
#6332=ORIENTED_EDGE ( 'NONE', *, *, #13511, .T. ) ;
#6333=VECTOR ( 'NONE', #3103, 1000.000000000000000 ) ;
#6334=CARTESIAN_POINT ( 'NONE',  ( -34.68921677370540380, -25.75213315644277046, 1.869203119972154228E-14 ) ) ;
#6335=EDGE_CURVE ( 'NONE', #7658, #2224, #2007, .T. ) ;
#6337=EDGE_LOOP ( 'NONE', ( #445, #1075, #6599, #7226 ) ) ;
#6339=CARTESIAN_POINT ( 'NONE',  ( -11.76885329963143434, -17.05403346649147522, -21.65063509461097979 ) ) ;
#6340=VECTOR ( 'NONE', #3394, 1000.000000000000000 ) ;
#6341=DIRECTION ( 'NONE',  ( -0.9876526153536336894, -0.1566598588826349503, 0.000000000000000000 ) ) ;
#6342=CARTESIAN_POINT ( 'NONE',  ( -75.96627329761737712, -27.23692429386252911, -21.65063509461097979 ) ) ;
#6343=CYLINDRICAL_SURFACE ( 'NONE', #1920, 1.500000000000000666 ) ;
#6344=VECTOR ( 'NONE', #5336, 1000.000000000000000 ) ;
#6345=ORIENTED_EDGE ( 'NONE', *, *, #2716, .T. ) ;
#6346=CARTESIAN_POINT ( 'NONE',  ( -21.84973277410820458, -23.71555499096855613, -17.32050807568878170 ) ) ;
#6347=AXIS2_PLACEMENT_3D ( 'NONE', #9752, #9910, #11043 ) ;
#6348=DIRECTION ( 'NONE',  ( 0.000000000000000000, 0.000000000000000000, 1.000000000000000000 ) ) ;
#6349=AXIS2_PLACEMENT_3D ( 'NONE', #1971, #9263, #11809 ) ;
#6350=DIRECTION ( 'NONE',  ( -0.1566598588826321192, 0.9876526153536342445, 7.798540720466730171E-17 ) ) ;
#6351=CARTESIAN_POINT ( 'NONE',  ( -53.90880776292332399, -86.50618184100223118, 17.32050807568881368 ) ) ;
#6352=EDGE_LOOP ( 'NONE', ( #16119, #1329 ) ) ;
#6353=DIRECTION ( 'NONE',  ( -0.9876526153536341335, -0.1566598588826327021, 0.000000000000000000 ) ) ;
#6354=FACE_OUTER_BOUND ( 'NONE', #10669, .T. ) ;
#6355=FACE_OUTER_BOUND ( 'NONE', #2680, .T. ) ;
#6356=ORIENTED_EDGE ( 'NONE', *, *, #5686, .F. ) ;
#6357=CIRCLE ( 'NONE', #4807, 1.500000000000000888 ) ;
#6358=FACE_OUTER_BOUND ( 'NONE', #5010, .T. ) ;
#6359=EDGE_CURVE ( 'NONE', #10712, #15083, #10051, .T. ) ;
#6360=CIRCLE ( 'NONE', #4809, 1.500000000000000888 ) ;
#6362=VERTEX_POINT ( 'NONE', #6334 ) ;
#6363=CIRCLE ( 'NONE', #14518, 1.499999999999999556 ) ;
#6364=AXIS2_PLACEMENT_3D ( 'NONE', #1345, #14217, #2915 ) ;
#6366=EDGE_CURVE ( 'NONE', #10934, #6176, #8673, .T. ) ;
#6367=CARTESIAN_POINT ( 'NONE',  ( -15.39035576413176187, -80.39644734457958464, 21.65063509461101532 ) ) ;
#6368=CARTESIAN_POINT ( 'NONE',  ( -23.33121169713865584, -23.95054477929251036, 17.32050807568881723 ) ) ;
#6369=CARTESIAN_POINT ( 'NONE',  ( -21.64537945316773460, -18.62063205531779886, 4.330127018922218518 ) ) ;
#6370=AXIS2_PLACEMENT_3D ( 'NONE', #2348, #2457, #12261 ) ;
#6371=DIRECTION ( 'NONE',  ( -0.9876526153536341335, -0.1566598588826327021, 0.000000000000000000 ) ) ;
#6372=AXIS2_PLACEMENT_3D ( 'NONE', #3331, #9135, #6110 ) ;
#6373=LINE ( 'NONE', #13255, #6340 ) ;
#6374=FACE_OUTER_BOUND ( 'NONE', #15680, .T. ) ;
#6375=EDGE_LOOP ( 'NONE', ( #10523, #17326 ) ) ;
#6376=FACE_BOUND ( 'NONE', #18173, .T. ) ;
#6380=DIRECTION ( 'NONE',  ( -0.9876526153536341335, -0.1566598588826327021, 0.000000000000000000 ) ) ;
#6381=VECTOR ( 'NONE', #4767, 1000.000000000000000 ) ;
#6382=DIRECTION ( 'NONE',  ( -0.1566598588826321192, 0.9876526153536342445, 7.798540720466730171E-17 ) ) ;
#6383=ORIENTED_EDGE ( 'NONE', *, *, #11287, .F. ) ;
#6384=EDGE_LOOP ( 'NONE', ( #853, #5228, #6227, #15566 ) ) ;
#6385=VERTEX_POINT ( 'NONE', #16741 ) ;
#6386=CARTESIAN_POINT ( 'NONE',  ( -15.92381708198642798, -22.77559583767277473, -12.99038105676658006 ) ) ;
#6387=ADVANCED_FACE ( 'NONE', ( #5253 ), #623, .F. ) ;
#6388=EDGE_CURVE ( 'NONE', #9162, #10150, #2901, .T. ) ;
#6389=AXIS2_PLACEMENT_3D ( 'NONE', #7948, #3045, #11641 ) ;
#6390=FACE_BOUND ( 'NONE', #12095, .T. ) ;
#6391=EDGE_CURVE ( 'NONE', #8304, #16372, #7758, .T. ) ;
#6394=AXIS2_PLACEMENT_3D ( 'NONE', #3479, #7767, #12104 ) ;
#6395=EDGE_LOOP ( 'NONE', ( #12612, #1090, #11232, #6314 ) ) ;
#6396=ORIENTED_EDGE ( 'NONE', *, *, #15746, .F. ) ;
#6397=DIRECTION ( 'NONE',  ( -0.9876526153536336894, -0.1566598588826349503, 0.000000000000000000 ) ) ;
#6398=EDGE_LOOP ( 'NONE', ( #10502, #15851 ) ) ;
#6399=DIRECTION ( 'NONE',  ( -0.9876526153536336894, -0.1566598588826349503, 0.000000000000000000 ) ) ;
#6400=VECTOR ( 'NONE', #11514, 1000.000000000000000 ) ;
#6401=DIRECTION ( 'NONE',  ( -0.9876526153536341335, -0.1566598588826327021, 0.000000000000000000 ) ) ;
#6405=VERTEX_POINT ( 'NONE', #16428 ) ;
#6407=ADVANCED_FACE ( 'NONE', ( #5991 ), #12122, .F. ) ;
#6408=CARTESIAN_POINT ( 'NONE',  ( -78.43540483600145308, -27.62857394106911002, -17.32050807568878170 ) ) ;
#6410=ADVANCED_FACE ( 'NONE', ( #4654 ), #14893, .F. ) ;
#6412=ORIENTED_EDGE ( 'NONE', *, *, #14761, .F. ) ;
#6414=VERTEX_POINT ( 'NONE', #595 ) ;
#6415=DIRECTION ( 'NONE',  ( -0.1566598588826321747, 0.9876526153536343555, 0.000000000000000000 ) ) ;
#6417=DIRECTION ( 'NONE',  ( -0.9876526153536336894, -0.1566598588826349503, 0.000000000000000000 ) ) ;
#6421=DIRECTION ( 'NONE',  ( 0.000000000000000000, 0.000000000000000000, 1.000000000000000000 ) ) ;
#6422=DIRECTION ( 'NONE',  ( -0.1566598588826321192, 0.9876526153536342445, 7.798540720466730171E-17 ) ) ;
#6423=VECTOR ( 'NONE', #1511, 1000.000000000000000 ) ;
#6424=AXIS2_PLACEMENT_3D ( 'NONE', #17319, #2955, #15861 ) ;
#6425=CYLINDRICAL_SURFACE ( 'NONE', #11031, 1.500000000000001554 ) ;
#6426=ORIENTED_EDGE ( 'NONE', *, *, #10838, .T. ) ;
#6427=VERTEX_POINT ( 'NONE', #3135 ) ;
#6428=CARTESIAN_POINT ( 'NONE',  ( 7.819480696678551723, -76.71494066083772623, 12.99038105676660493 ) ) ;
#6429=ORIENTED_EDGE ( 'NONE', *, *, #8088, .T. ) ;
#6431=ORIENTED_EDGE ( 'NONE', *, *, #11947, .F. ) ;
#6433=EDGE_LOOP ( 'NONE', ( #424, #5699 ) ) ;
#6435=CARTESIAN_POINT ( 'NONE',  ( -1.109027851681966492, -20.42569795443330349, -12.99038105676658361 ) ) ;
#6436=EDGE_CURVE ( 'NONE', #855, #16087, #5947, .T. ) ;
#6438=VECTOR ( 'NONE', #18254, 1000.000000000000000 ) ;
#6439=CARTESIAN_POINT ( 'NONE',  ( -53.90880776292333820, -86.50618184100221697, 8.660254037844412167 ) ) ;
#6440=EDGE_CURVE ( 'NONE', #3894, #11326, #11069, .T. ) ;
#6443=DIRECTION ( 'NONE',  ( -0.9876526153536344665, -0.1566598588826304539, 0.000000000000000000 ) ) ;
#6444=ADVANCED_FACE ( 'NONE', ( #13178 ), #6190, .F. ) ;
#6445=DIRECTION ( 'NONE',  ( -0.1566598588826321192, 0.9876526153536342445, 7.798540720466730171E-17 ) ) ;
#6446=DIRECTION ( 'NONE',  ( -0.1566598588826321192, 0.9876526153536342445, 7.798540720466730171E-17 ) ) ;
#6447=DIRECTION ( 'NONE',  ( -0.9876526153536336894, -0.1566598588826350336, 0.000000000000000000 ) ) ;
#6448=EDGE_LOOP ( 'NONE', ( #13683, #7326, #3689, #5031, #13136, #11872, #406 ) ) ;
#6449=CARTESIAN_POINT ( 'NONE',  ( -5.059638313096497697, -21.05233738996382797, -17.32050807568878170 ) ) ;
#6450=DIRECTION ( 'NONE',  ( -0.1566598588826321747, 0.9876526153536343555, 0.000000000000000000 ) ) ;
#6451=ORIENTED_EDGE ( 'NONE', *, *, #5760, .T. ) ;
#6453=FACE_OUTER_BOUND ( 'NONE', #6230, .T. ) ;
#6454=ORIENTED_EDGE ( 'NONE', *, *, #18785, .T. ) ;
#6455=DIRECTION ( 'NONE',  ( 0.000000000000000000, 0.000000000000000000, 1.000000000000000000 ) ) ;
#6456=AXIS2_PLACEMENT_3D ( 'NONE', #2280, #3978, #6852 ) ;
#6457=VERTEX_POINT ( 'NONE', #2001 ) ;
#6458=LINE ( 'NONE', #2350, #10025 ) ;
#6459=EDGE_LOOP ( 'NONE', ( #2094, #13710 ) ) ;
#6460=DIRECTION ( 'NONE',  ( -0.1566598588826321192, 0.9876526153536342445, 7.798540720466730171E-17 ) ) ;
#6462=CYLINDRICAL_SURFACE ( 'NONE', #18218, 1.500000000000001554 ) ;
#6464=UNCERTAINTY_MEASURE_WITH_UNIT (LENGTH_MEASURE( 1.000000000000000082E-05 ), #8318, 'distance_accuracy_value', 'NONE');
#6465=EDGE_CURVE ( 'NONE', #10326, #6414, #7172, .T. ) ;
#6467=ORIENTED_EDGE ( 'NONE', *, *, #833, .F. ) ;
#6468=DIRECTION ( 'NONE',  ( 0.000000000000000000, 0.000000000000000000, 1.000000000000000000 ) ) ;
#6469=ORIENTED_EDGE ( 'NONE', *, *, #13408, .T. ) ;
#6470=CARTESIAN_POINT ( 'NONE',  ( -60.16383145195930382, -24.73036655174043830, 17.32050807568881723 ) ) ;
#6471=ADVANCED_FACE ( 'NONE', ( #14704 ), #1721, .F. ) ;
#6476=VERTEX_POINT ( 'NONE', #16224 ) ;
#6477=FACE_OUTER_BOUND ( 'NONE', #18643, .T. ) ;
#6479=FACE_BOUND ( 'NONE', #4848, .T. ) ;
#6480=CARTESIAN_POINT ( 'NONE',  ( -13.25033222266188915, -17.28902325481542235, -12.99038105676658006 ) ) ;
#6481=ORIENTED_EDGE ( 'NONE', *, *, #11786, .T. ) ;
#6482=EDGE_CURVE ( 'NONE', #862, #8986, #3192, .T. ) ;
#6483=CARTESIAN_POINT ( 'NONE',  ( -19.17624791478365864, -18.22898240811121795, 17.32050807568881368 ) ) ;
#6484=FACE_BOUND ( 'NONE', #6286, .T. ) ;
#6485=CARTESIAN_POINT ( 'NONE',  ( -39.09401853261888959, -84.15628395776272441, -8.660254037844385522 ) ) ;
#6486=CARTESIAN_POINT ( 'NONE',  ( -41.39843176024034221, -21.75382923297042481, -21.65063509461097979 ) ) ;
#6487=DIRECTION ( 'NONE',  ( -0.1566598588826321192, 0.9876526153536342445, 7.798540720466731404E-17 ) ) ;
#6489=DIRECTION ( 'NONE',  ( -0.1566598588826321192, 0.9876526153536342445, 7.798540720466730171E-17 ) ) ;
#6491=ORIENTED_EDGE ( 'NONE', *, *, #1349, .T. ) ;
#6492=DIRECTION ( 'NONE',  ( -0.1566598588826321192, 0.9876526153536342445, 7.798540720466730171E-17 ) ) ;
#6494=CARTESIAN_POINT ( 'NONE',  ( -76.66445292623467367, -32.41017715895461038, 4.330127018922217630 ) ) ;
#6495=ORIENTED_EDGE ( 'NONE', *, *, #2052, .F. ) ;
#6496=DIRECTION ( 'NONE',  ( -0.1566598588826321192, 0.9876526153536342445, 7.798540720466730171E-17 ) ) ;
#6499=ORIENTED_EDGE ( 'NONE', *, *, #16137, .T. ) ;
#6500=CARTESIAN_POINT ( 'NONE',  ( -25.10216360690543524, -19.16894156140701355, 4.330127018922218518 ) ) ;
#6502=CARTESIAN_POINT ( 'NONE',  ( -6.830590222863280658, -16.27073417207831696, 12.99038105676661026 ) ) ;
#6503=ADVANCED_FACE ( 'NONE', ( #7508 ), #13375, .F. ) ;
#6504=ADVANCED_FACE ( 'NONE', ( #10525 ), #17860, .F. ) ;
#6505=EDGE_CURVE ( 'NONE', #14684, #8813, #15356, .T. ) ;
#6506=DIRECTION ( 'NONE',  ( -0.1566598588826321192, 0.9876526153536342445, 7.798540720466731404E-17 ) ) ;
#6507=AXIS2_PLACEMENT_3D ( 'NONE', #4030, #12851, #773 ) ;
#6508=DIRECTION ( 'NONE',  ( -0.9876526153536341335, -0.1566598588826327021, 0.000000000000000000 ) ) ;
#6510=DIRECTION ( 'NONE',  ( 0.000000000000000000, 0.000000000000000000, 1.000000000000000000 ) ) ;
#6511=ORIENTED_EDGE ( 'NONE', *, *, #1694, .F. ) ;
#6512=EDGE_LOOP ( 'NONE', ( #16847, #16183, #10652, #226 ) ) ;
#6515=ORIENTED_EDGE ( 'NONE', *, *, #7985, .F. ) ;
#6516=DIRECTION ( 'NONE',  ( -0.1566598588826321192, 0.9876526153536342445, 7.798540720466730171E-17 ) ) ;
#6517=EDGE_LOOP ( 'NONE', ( #10049, #7722, #15650, #14614 ) ) ;
#6519=VERTEX_POINT ( 'NONE', #16903 ) ;
#6520=AXIS2_PLACEMENT_3D ( 'NONE', #16264, #18085, #10737 ) ;
#6521=FACE_OUTER_BOUND ( 'NONE', #1977, .T. ) ;
#6522=CARTESIAN_POINT ( 'NONE',  ( -84.16561914167411373, 33.60000000000000142, 30.00000000000000000 ) ) ;
#6525=DIRECTION ( 'NONE',  ( -0.9876526153536341335, -0.1566598588826327021, 0.000000000000000000 ) ) ;
#6526=DIRECTION ( 'NONE',  ( -0.000000000000000000, -0.000000000000000000, -1.000000000000000000 ) ) ;
#6527=CARTESIAN_POINT ( 'NONE',  ( -43.86756329862440396, -22.14547888017701638, 17.32050807568882078 ) ) ;
#6528=CYLINDRICAL_SURFACE ( 'NONE', #11421, 1.500000000000001554 ) ;
#6529=CARTESIAN_POINT ( 'NONE',  ( -29.21749237908258223, -82.58968536893642920, 17.32050807568881368 ) ) ;
#6530=AXIS2_PLACEMENT_3D ( 'NONE', #17497, #5743, #53 ) ;
#6531=CARTESIAN_POINT ( 'NONE',  ( -18.39294862037050393, -23.16724548487935564, -8.660254037844380193 ) ) ;
#6532=EDGE_LOOP ( 'NONE', ( #8546, #12257, #8881, #16343 ) ) ;
#6534=VERTEX_POINT ( 'NONE', #5321 ) ;
#6535=ADVANCED_FACE ( 'NONE', ( #18351 ), #15074, .F. ) ;
#6537=ORIENTED_EDGE ( 'NONE', *, *, #14509, .F. ) ;
#6538=EDGE_LOOP ( 'NONE', ( #16683, #18334 ) ) ;
#6539=AXIS2_PLACEMENT_3D ( 'NONE', #16797, #15339, #11824 ) ;
#6541=ORIENTED_EDGE ( 'NONE', *, *, #4930, .T. ) ;
#6542=CARTESIAN_POINT ( 'NONE',  ( -25.76070822534488869, -82.04137586284720385, -8.660254037844385522 ) ) ;
#6543=AXIS2_PLACEMENT_3D ( 'NONE', #896, #6679, #10996 ) ;
#6545=CARTESIAN_POINT ( 'NONE',  ( -24.27922930231443743, -81.80638607452326028, 1.424741226644455312E-14 ) ) ;
#6546=CARTESIAN_POINT ( 'NONE',  ( -46.50141314777110324, -85.33123289938248490, 12.99038105676661203 ) ) ;
#6547=DIRECTION ( 'NONE',  ( -0.9876526153536336894, -0.1566598588826349503, 0.000000000000000000 ) ) ;
#6548=DIRECTION ( 'NONE',  ( -0.1566598588826321747, 0.9876526153536343555, 0.000000000000000000 ) ) ;
#6549=CARTESIAN_POINT ( 'NONE',  ( -58.68235252892885256, -24.49537676341649117, 17.32050807568882078 ) ) ;
#6550=CARTESIAN_POINT ( 'NONE',  ( -24.81269062016911064, -24.18553456761645393, 1.869203119972154228E-14 ) ) ;
#6552=FACE_BOUND ( 'NONE', #6375, .T. ) ;
#6553=DIRECTION ( 'NONE',  ( -0.1566598588826321192, 0.9876526153536342445, 7.798540720466731404E-17 ) ) ;
#6555=AXIS2_PLACEMENT_3D ( 'NONE', #9212, #15463, #9693 ) ;
#6556=DIRECTION ( 'NONE',  ( -0.9876526153536341335, -0.1566598588826327021, 0.000000000000000000 ) ) ;
#6558=DIRECTION ( 'NONE',  ( -0.000000000000000000, -0.000000000000000000, -1.000000000000000000 ) ) ;
#6560=ORIENTED_EDGE ( 'NONE', *, *, #12128, .T. ) ;
#6562=VERTEX_POINT ( 'NONE', #8269 ) ;
#6563=CARTESIAN_POINT ( 'NONE',  ( -21.81009776393036503, -81.41473642731668292, 4.330127018922213189 ) ) ;
#6564=ADVANCED_FACE ( 'NONE', ( #12589 ), #14031, .F. ) ;
#6565=FACE_BOUND ( 'NONE', #8257, .T. ) ;
#6566=AXIS2_PLACEMENT_3D ( 'NONE', #9723, #8725, #4274 ) ;
#6568=ORIENTED_EDGE ( 'NONE', *, *, #8887, .T. ) ;
#6569=CARTESIAN_POINT ( 'NONE',  ( -53.90880776292332399, -86.50618184100223118, 17.32050807568881368 ) ) ;
#6570=DIRECTION ( 'NONE',  ( -0.1566598588826321192, 0.9876526153536342445, 7.798540720466730171E-17 ) ) ;
#6572=CARTESIAN_POINT ( 'NONE',  ( -36.46016868347218320, -20.97052993855726655, -12.99038105676658006 ) ) ;
#6573=CARTESIAN_POINT ( 'NONE',  ( -67.57122606711152457, -25.90531549336017747, 21.65063509461101887 ) ) ;
#6575=VERTEX_POINT ( 'NONE', #7885 ) ;
#6576=DIRECTION ( 'NONE',  ( -0.1566598588826321192, 0.9876526153536342445, 7.798540720466730171E-17 ) ) ;
#6577=AXIS2_PLACEMENT_3D ( 'NONE', #14959, #4445, #4637 ) ;
#6581=DIRECTION ( 'NONE',  ( -0.1566598588826321747, 0.9876526153536343555, 0.000000000000000000 ) ) ;
#6582=EDGE_CURVE ( 'NONE', #3440, #11862, #3867, .T. ) ;
#6583=ORIENTED_EDGE ( 'NONE', *, *, #10801, .F. ) ;
#6584=CIRCLE ( 'NONE', #13802, 144.0000000000000284 ) ;
#6585=ORIENTED_EDGE ( 'NONE', *, *, #3981, .T. ) ;
#6587=AXIS2_PLACEMENT_3D ( 'NONE', #16201, #17830, #10320 ) ;
#6588=DIRECTION ( 'NONE',  ( -0.1566598588826321747, 0.9876526153536343555, 0.000000000000000000 ) ) ;
#6590=ADVANCED_FACE ( 'NONE', ( #9580 ), #6759, .F. ) ;
#6591=CARTESIAN_POINT ( 'NONE',  ( -3.373806069125576901, -15.72242466598909871, -12.99038105676658361 ) ) ;
#6592=DIRECTION ( 'NONE',  ( -0.9876526153536341335, -0.1566598588826327021, 0.000000000000000000 ) ) ;
#6594=DIRECTION ( 'NONE',  ( -0.9876526153536344665, -0.1566598588826304539, 0.000000000000000000 ) ) ;
#6595=LINE ( 'NONE', #1106, #10782 ) ;
#6596=AXIS2_PLACEMENT_3D ( 'NONE', #2500, #798, #2210 ) ;
#6597=LINE ( 'NONE', #18198, #9841 ) ;
#6598=ORIENTED_EDGE ( 'NONE', *, *, #5915, .F. ) ;
#6599=ORIENTED_EDGE ( 'NONE', *, *, #3449, .T. ) ;
#6600=DIRECTION ( 'NONE',  ( -0.1566598588826321192, 0.9876526153536342445, 7.798540720466730171E-17 ) ) ;
#6602=AXIS2_PLACEMENT_3D ( 'NONE', #5080, #17825, #13421 ) ;
#6603=CYLINDRICAL_SURFACE ( 'NONE', #3323, 1.500000000000001554 ) ;
#6604=VERTEX_POINT ( 'NONE', #2191 ) ;
#6605=VERTEX_POINT ( 'NONE', #13729 ) ;
#6606=DIRECTION ( 'NONE',  ( -0.1566598588826321192, 0.9876526153536342445, 7.798540720466731404E-17 ) ) ;
#6607=CARTESIAN_POINT ( 'NONE',  ( -10.94591899504043830, -79.69147797960773971, -8.660254037844385522 ) ) ;
#6608=ADVANCED_FACE ( 'NONE', ( #6477 ), #11174, .T. ) ;
#6609=CIRCLE ( 'NONE', #9961, 1.500000000000000444 ) ;
#6610=ADVANCED_FACE ( 'NONE', ( #13833 ), #10982, .F. ) ;
#6611=CARTESIAN_POINT ( 'NONE',  ( -51.43967622453926936, -86.11453219379562540, -12.99038105676658539 ) ) ;
#6612=AXIS2_PLACEMENT_3D ( 'NONE', #5503, #8254, #6833 ) ;
#6613=ADVANCED_FACE ( 'NONE', ( #18051 ), #5122, .F. ) ;
#6614=ORIENTED_EDGE ( 'NONE', *, *, #5686, .T. ) ;
#6615=FACE_OUTER_BOUND ( 'NONE', #4732, .T. ) ;
#6616=LINE ( 'NONE', #16563, #11182 ) ;
#6617=CYLINDRICAL_SURFACE ( 'NONE', #15506, 1.500000000000001554 ) ;
#6618=CARTESIAN_POINT ( 'NONE',  ( -33.20773785067495254, -25.51714336811882688, -8.660254037844380193 ) ) ;
#6621=CIRCLE ( 'NONE', #13250, 1.500000000000000888 ) ;
#6622=FACE_OUTER_BOUND ( 'NONE', #6532, .T. ) ;
#6624=DIRECTION ( 'NONE',  ( 0.000000000000000000, 0.000000000000000000, 1.000000000000000000 ) ) ;
#6626=DIRECTION ( 'NONE',  ( 0.000000000000000000, 0.000000000000000000, 1.000000000000000000 ) ) ;
#6627=EDGE_LOOP ( 'NONE', ( #13443, #6715 ) ) ;
#6630=ORIENTED_EDGE ( 'NONE', *, *, #13694, .F. ) ;
#6631=VERTEX_POINT ( 'NONE', #5013 ) ;
#6632=AXIS2_PLACEMENT_3D ( 'NONE', #16816, #17005, #15363 ) ;
#6633=EDGE_CURVE ( 'NONE', #6767, #10467, #12583, .T. ) ;
#6634=AXIS2_PLACEMENT_3D ( 'NONE', #15647, #121, #5899 ) ;
#6636=EDGE_LOOP ( 'NONE', ( #4947, #17880 ) ) ;
#6637=AXIS2_PLACEMENT_3D ( 'NONE', #15449, #17164, #1253 ) ;
#6639=DIRECTION ( 'NONE',  ( 1.000000000000000000, 0.000000000000000000, -2.995206001686573514E-16 ) ) ;
#6641=CARTESIAN_POINT ( 'NONE',  ( -52.96079015774756016, -28.65034054577145994, 8.660254037844417496 ) ) ;
#6642=DIRECTION ( 'NONE',  ( -0.1566598588826321192, 0.9876526153536342445, 7.798540720466730171E-17 ) ) ;
#6643=CARTESIAN_POINT ( 'NONE',  ( -11.76885329963143079, -17.05403346649147878, 4.330127018922214965 ) ) ;
#6645=CARTESIAN_POINT ( 'NONE',  ( 6.338001773648100468, -76.94993044916168401, 4.330127018922207860 ) ) ;
#6646=CYLINDRICAL_SURFACE ( 'NONE', #2889, 1.500000000000001554 ) ;
#6648=CARTESIAN_POINT ( 'NONE',  ( -25.80034323552273179, -24.34219442649909126, -4.330127018922181215 ) ) ;
#6649=ORIENTED_EDGE ( 'NONE', *, *, #15138, .T. ) ;
#6650=AXIS2_PLACEMENT_3D ( 'NONE', #8660, #1462, #13100 ) ;
#6652=CARTESIAN_POINT ( 'NONE',  ( -60.32854976272193426, -87.52447092373932946, 1.424741226644455312E-14 ) ) ;
#6653=CIRCLE ( 'NONE', #5112, 1.500000000000000888 ) ;
#6654=CIRCLE ( 'NONE', #10849, 1.500000000000000888 ) ;
#6655=DIRECTION ( 'NONE',  ( -0.1566598588826321192, 0.9876526153536342445, 7.798540720466730171E-17 ) ) ;
#6656=VECTOR ( 'NONE', #1400, 1000.000000000000114 ) ;
#6657=AXIS2_PLACEMENT_3D ( 'NONE', #10017, #11248, #9918 ) ;
#6658=EDGE_LOOP ( 'NONE', ( #18381, #17098, #18280, #11727 ) ) ;
#6659=ORIENTED_EDGE ( 'NONE', *, *, #7525, .T. ) ;
#6661=CARTESIAN_POINT ( 'NONE',  ( -61.15148406731293562, -24.88702641062305432, -21.65063509461097979 ) ) ;
#6662=DIRECTION ( 'NONE',  ( -0.1566598588826321192, 0.9876526153536342445, 7.798540720466730171E-17 ) ) ;
#6663=FACE_BOUND ( 'NONE', #6173, .T. ) ;
#6664=CIRCLE ( 'NONE', #13904, 1.500000000000000444 ) ;
#6665=CIRCLE ( 'NONE', #5763, 1.500000000000000000 ) ;
#6667=AXIS2_PLACEMENT_3D ( 'NONE', #2385, #15368, #8179 ) ;
#6670=AXIS2_PLACEMENT_3D ( 'NONE', #16259, #6506, #1856 ) ;
#6671=ADVANCED_FACE ( 'NONE', ( #5609 ), #14507, .F. ) ;
#6672=AXIS2_PLACEMENT_3D ( 'NONE', #10000, #8599, #16794 ) ;
#6673=DIRECTION ( 'NONE',  ( -0.9876526153536336894, -0.1566598588826349503, 0.000000000000000000 ) ) ;
#6674=EDGE_CURVE ( 'NONE', #7247, #8478, #1420, .T. ) ;
#6675=DIRECTION ( 'NONE',  ( -0.1566598588826321747, 0.9876526153536343555, 0.000000000000000000 ) ) ;
#6678=AXIS2_PLACEMENT_3D ( 'NONE', #16668, #13889, #938 ) ;
#6679=DIRECTION ( 'NONE',  ( -0.1566598588826321747, 0.9876526153536343555, 0.000000000000000000 ) ) ;
#6680=ORIENTED_EDGE ( 'NONE', *, *, #13245, .F. ) ;
#6681=ORIENTED_EDGE ( 'NONE', *, *, #14864, .F. ) ;
#6682=CARTESIAN_POINT ( 'NONE',  ( -79.23462711737164454, 33.01666666666666572, 35.00000000000000000 ) ) ;
#6684=AXIS2_PLACEMENT_3D ( 'NONE', #13513, #1968, #6353 ) ;
#6685=LINE ( 'NONE', #8077, #535 ) ;
#6686=VERTEX_POINT ( 'NONE', #4269 ) ;
#6687=VERTEX_POINT ( 'NONE', #11275 ) ;
#6688=CIRCLE ( 'NONE', #5783, 1.500000000000000000 ) ;
#6690=AXIS2_PLACEMENT_3D ( 'NONE', #577, #13809, #9474 ) ;
#6691=ORIENTED_EDGE ( 'NONE', *, *, #4340, .T. ) ;
#6693=CIRCLE ( 'NONE', #14262, 1.499999999999999556 ) ;
#6694=DIRECTION ( 'NONE',  ( -0.1566598588826321192, 0.9876526153536342445, 7.798540720466731404E-17 ) ) ;
#6695=AXIS2_PLACEMENT_3D ( 'NONE', #1408, #17348, #1501 ) ;
#6698=EDGE_CURVE ( 'NONE', #1785, #11499, #4062, .T. ) ;
#6701=CARTESIAN_POINT ( 'NONE',  ( -61.15148406731293562, -24.88702641062306498, 4.330127018922218518 ) ) ;
#6702=DIRECTION ( 'NONE',  ( -0.000000000000000000, -0.000000000000000000, -1.000000000000000000 ) ) ;
#6703=CIRCLE ( 'NONE', #4557, 1.500000000000000444 ) ;
#6704=CARTESIAN_POINT ( 'NONE',  ( -26.78799585087635649, -24.49885428538171794, 1.887572821959364500E-14 ) ) ;
#6705=ORIENTED_EDGE ( 'NONE', *, *, #18448, .F. ) ;
#6707=CARTESIAN_POINT ( 'NONE',  ( -65.10209452872746283, -25.51366584615358235, -17.32050807568878170 ) ) ;
#6708=LINE ( 'NONE', #1115, #15776 ) ;
#6709=EDGE_CURVE ( 'NONE', #495, #11172, #3514, .T. ) ;
#6710=CIRCLE ( 'NONE', #12426, 1.500000000000001332 ) ;
#6711=EDGE_LOOP ( 'NONE', ( #15884, #14174, #13431, #9586 ) ) ;
#6714=CIRCLE ( 'NONE', #11515, 1.500000000000000888 ) ;
#6715=ORIENTED_EDGE ( 'NONE', *, *, #17929, .T. ) ;
#6716=CARTESIAN_POINT ( 'NONE',  ( 1.399738696879940791, -77.73322974357483872, -12.99038105676658539 ) ) ;
#6717=DIRECTION ( 'NONE',  ( -0.1566598588826321192, 0.9876526153536342445, 7.798540720466730171E-17 ) ) ;
#6718=VECTOR ( 'NONE', #3890, 1000.000000000000000 ) ;
#6719=DIRECTION ( 'NONE',  ( -0.1566598588826321192, 0.9876526153536342445, 7.798540720466730171E-17 ) ) ;
#6720=FACE_OUTER_BOUND ( 'NONE', #17156, .T. ) ;
#6722=EDGE_LOOP ( 'NONE', ( #8948, #18422, #3755, #12459 ) ) ;
#6723=DIRECTION ( 'NONE',  ( -0.9876526153536336894, -0.1566598588826349503, 0.000000000000000000 ) ) ;
#6724=CIRCLE ( 'NONE', #5817, 1.500000000000000888 ) ;
#6725=VECTOR ( 'NONE', #4576, 1000.000000000000000 ) ;
#6726=DIRECTION ( 'NONE',  ( -0.1566598588826321192, 0.9876526153536342445, 7.798540720466730171E-17 ) ) ;
#6727=CARTESIAN_POINT ( 'NONE',  ( -1.109027851681966492, -20.42569795443330349, 4.330127018922212301 ) ) ;
#6730=ADVANCED_FACE ( 'NONE', ( #17288 ), #10046, .F. ) ;
#6731=VERTEX_POINT ( 'NONE', #5807 ) ;
#6733=CARTESIAN_POINT ( 'NONE',  ( -33.20773785067495965, -25.51714336811882688, 8.660254037844417496 ) ) ;
#6734=ORIENTED_EDGE ( 'NONE', *, *, #17995, .T. ) ;
#6735=EDGE_LOOP ( 'NONE', ( #1810, #13339, #14482, #10597 ) ) ;
#6736=CIRCLE ( 'NONE', #4598, 1.500000000000000888 ) ;
#6739=SHAPE_REPRESENTATION ( 'Heavy-Duty Perforated Sieve Plate', ( #18772 ), #7243 ) ;
#6741=CARTESIAN_POINT ( 'NONE',  ( -13.45468554360235203, -22.38394619046619383, 17.32050807568881012 ) ) ;
#6742=CARTESIAN_POINT ( 'NONE',  ( 5.350349158294472218, -77.10659030804430358, -8.660254037844389075 ) ) ;
#6743=DIRECTION ( 'NONE',  ( -0.1566598588826321192, 0.9876526153536342445, 7.798540720466730171E-17 ) ) ;
#6746=EDGE_CURVE ( 'NONE', #12053, #8550, #16559, .T. ) ;
#6747=EDGE_CURVE ( 'NONE', #592, #10493, #7480, .T. ) ;
#6748=CARTESIAN_POINT ( 'NONE',  ( 0.3724510713484854851, -20.19070816610934926, -4.330127018922184767 ) ) ;
#6750=ADVANCED_FACE ( 'NONE', ( #1268 ), #17183, .F. ) ;
#6751=CYLINDRICAL_SURFACE ( 'NONE', #8086, 1.500000000000001554 ) ;
#6752=DIRECTION ( 'NONE',  ( -0.1566598588826321192, 0.9876526153536342445, 7.798540720466731404E-17 ) ) ;
#6753=DIRECTION ( 'NONE',  ( 0.000000000000000000, 0.000000000000000000, 1.000000000000000000 ) ) ;
#6754=VECTOR ( 'NONE', #18264, 1000.000000000000000 ) ;
#6755=AXIS2_PLACEMENT_3D ( 'NONE', #18070, #9797, #5035 ) ;
#6756=VERTEX_POINT ( 'NONE', #7228 ) ;
#6757=ORIENTED_EDGE ( 'NONE', *, *, #2364, .T. ) ;
#6758=ORIENTED_EDGE ( 'NONE', *, *, #12819, .F. ) ;
#6759=CYLINDRICAL_SURFACE ( 'NONE', #12888, 1.500000000000001554 ) ;
#6760=FACE_BOUND ( 'NONE', #13461, .T. ) ;
#6761=CARTESIAN_POINT ( 'NONE',  ( -62.30385499342917655, -87.83779064150458282, 17.32050807568881368 ) ) ;
#6763=CARTESIAN_POINT ( 'NONE',  ( 2.447859171744382056, -14.79900155049411659, 30.00000000000000000 ) ) ;
#6764=AXIS2_PLACEMENT_3D ( 'NONE', #18128, #1152, #8252 ) ;
#6765=DIRECTION ( 'NONE',  ( -0.9876526153536341335, -0.1566598588826327021, 0.000000000000000000 ) ) ;
#6766=DIRECTION ( 'NONE',  ( -0.1566598588826321192, 0.9876526153536342445, 7.798540720466731404E-17 ) ) ;
#6767=VERTEX_POINT ( 'NONE', #2765 ) ;
#6769=CARTESIAN_POINT ( 'NONE',  ( -68.76323200340563346, -31.15689828789355786, -4.330127018922181215 ) ) ;
#6773=ORIENTED_EDGE ( 'NONE', *, *, #8841, .F. ) ;
#6774=DIRECTION ( 'NONE',  ( -0.1566598588826321747, 0.9876526153536343555, 0.000000000000000000 ) ) ;
#6776=EDGE_CURVE ( 'NONE', #6575, #10405, #15327, .T. ) ;
#6778=EDGE_LOOP ( 'NONE', ( #608, #18440 ) ) ;
#6779=ORIENTED_EDGE ( 'NONE', *, *, #9879, .F. ) ;
#6780=ORIENTED_EDGE ( 'NONE', *, *, #3079, .F. ) ;
#6781=DIRECTION ( 'NONE',  ( -0.9876526153536336894, -0.1566598588826349503, 0.000000000000000000 ) ) ;
#6782=EDGE_CURVE ( 'NONE', #18003, #9146, #2917, .T. ) ;
#6783=ORIENTED_EDGE ( 'NONE', *, *, #8007, .F. ) ;
#6784=ORIENTED_EDGE ( 'NONE', *, *, #9685, .T. ) ;
#6785=CARTESIAN_POINT ( 'NONE',  ( -50.49165861936347710, -28.25869089856488614, -4.330127018922181215 ) ) ;
#6786=DIRECTION ( 'NONE',  ( -0.1566598588826321192, 0.9876526153536342445, 7.798540720466730171E-17 ) ) ;
#6787=CARTESIAN_POINT ( 'NONE',  ( -27.73601345605213098, -82.35469558061248563, 8.660254037844412167 ) ) ;
#6788=ORIENTED_EDGE ( 'NONE', *, *, #7078, .F. ) ;
#6790=FACE_OUTER_BOUND ( 'NONE', #3008, .T. ) ;
#6791=DIRECTION ( 'NONE',  ( -0.1566598588826321192, 0.9876526153536342445, 7.798540720466730171E-17 ) ) ;
#6792=EDGE_LOOP ( 'NONE', ( #15256, #13335, #18274, #11790 ) ) ;
#6793=CARTESIAN_POINT ( 'NONE',  ( -79.24244631363546887, 32.81909429640987952, 35.00000000000000000 ) ) ;
#6794=CARTESIAN_POINT ( 'NONE',  ( -9.299721761247353058, -16.66238381928489787, -8.660254037844380193 ) ) ;
#6796=ORIENTED_EDGE ( 'NONE', *, *, #3719, .T. ) ;
#6799=EDGE_LOOP ( 'NONE', ( #14200, #3844 ) ) ;
#6801=VERTEX_POINT ( 'NONE', #8350 ) ;
#6802=EDGE_CURVE ( 'NONE', #18385, #13575, #10178, .T. ) ;
#6803=DIRECTION ( 'NONE',  ( -0.9876526153536336894, -0.1566598588826349503, 0.000000000000000000 ) ) ;
#6805=ORIENTED_EDGE ( 'NONE', *, *, #945, .F. ) ;
#6806=DIRECTION ( 'NONE',  ( -0.1566598588826321192, 0.9876526153536342445, 7.798540720466730171E-17 ) ) ;
#6808=DIRECTION ( 'NONE',  ( -0.1566598588826321192, 0.9876526153536342445, 7.798540720466731404E-17 ) ) ;
#6810=DIRECTION ( 'NONE',  ( -0.1566598588826321747, 0.9876526153536343555, 0.000000000000000000 ) ) ;
#6811=CARTESIAN_POINT ( 'NONE',  ( -1.069392841504132052, -78.12487939078141608, 8.660254037844408614 ) ) ;
#6812=CARTESIAN_POINT ( 'NONE',  ( -33.99103714508810725, -20.57888029135068564, -17.32050807568878170 ) ) ;
#6813=EDGE_CURVE ( 'NONE', #8885, #17191, #814, .T. ) ;
#6815=ORIENTED_EDGE ( 'NONE', *, *, #18720, .T. ) ;
#6816=DIRECTION ( 'NONE',  ( -0.1566598588826321192, 0.9876526153536342445, 7.798540720466730171E-17 ) ) ;
#6818=VERTEX_POINT ( 'NONE', #8449 ) ;
#6819=DIRECTION ( 'NONE',  ( -0.1566598588826321192, 0.9876526153536342445, 7.798540720466731404E-17 ) ) ;
#6820=CARTESIAN_POINT ( 'NONE',  ( -1.892327146095128310, -15.48743487766515337, -21.65063509461097979 ) ) ;
#6824=AXIS2_PLACEMENT_3D ( 'NONE', #14696, #1715, #295 ) ;
#6825=CARTESIAN_POINT ( 'NONE',  ( -61.15148406731292852, -24.88702641062306853, 12.99038105676661736 ) ) ;
#6828=EDGE_CURVE ( 'NONE', #7702, #4043, #15943, .T. ) ;
#6830=ORIENTED_EDGE ( 'NONE', *, *, #16402, .F. ) ;
#6831=CARTESIAN_POINT ( 'NONE',  ( 0.5768043922889515285, -15.09578523045857601, 1.387778780781445676E-14 ) ) ;
#6832=DIRECTION ( 'NONE',  ( -0.9876526153536336894, -0.1566598588826349503, 0.000000000000000000 ) ) ;
#6833=DIRECTION ( 'NONE',  ( 0.000000000000000000, 0.000000000000000000, 1.000000000000000000 ) ) ;
#6834=ADVANCED_FACE ( 'NONE', ( #278 ), #13432, .F. ) ;
#6835=CARTESIAN_POINT ( 'NONE',  ( -74.48479437458692587, -27.00193450553859975, 12.99038105676661736 ) ) ;
#6836=AXIS2_PLACEMENT_3D ( 'NONE', #4412, #4603, #1671 ) ;
#6838=CARTESIAN_POINT ( 'NONE',  ( -24.11451099155181055, -19.01228170252437621, 1.908195823574487804E-14 ) ) ;
#6839=DIRECTION ( 'NONE',  ( -0.1566598588826321192, 0.9876526153536342445, 7.798540720466730171E-17 ) ) ;
#6840=CARTESIAN_POINT ( 'NONE',  ( 3.868870235264020963, -77.34158009636824715, 8.660254037844406838 ) ) ;
#6841=DIRECTION ( 'NONE',  ( -0.1566598588826321192, 0.9876526153536342445, 7.798540720466730171E-17 ) ) ;
#6842=DIRECTION ( 'NONE',  ( -0.1566598588826321747, 0.9876526153536343555, 0.000000000000000000 ) ) ;
#6844=ORIENTED_EDGE ( 'NONE', *, *, #3876, .F. ) ;
#6845=ORIENTED_EDGE ( 'NONE', *, *, #17437, .F. ) ;
#6846=DIRECTION ( 'NONE',  ( -0.1566598588826321192, 0.9876526153536342445, 7.798540720466730171E-17 ) ) ;
#6847=VECTOR ( 'NONE', #13289, 1000.000000000000000 ) ;
#6848=FACE_BOUND ( 'NONE', #1003, .T. ) ;
#6850=EDGE_CURVE ( 'NONE', #9530, #15072, #16018, .T. ) ;
#6852=DIRECTION ( 'NONE',  ( -0.9876526153536336894, -0.1566598588826349503, 0.000000000000000000 ) ) ;
#6853=ADVANCED_FACE ( 'NONE', ( #10324 ), #7681, .F. ) ;
#6854=VECTOR ( 'NONE', #17010, 1000.000000000000000 ) ;
#6855=LINE ( 'NONE', #15555, #2790 ) ;
#6856=VERTEX_POINT ( 'NONE', #1891 ) ;
#6857=EDGE_CURVE ( 'NONE', #3864, #11862, #1141, .T. ) ;
#6858=CARTESIAN_POINT ( 'NONE',  ( -15.88418207180859021, -80.47477727402089442, 17.32050807568881368 ) ) ;
#6859=CYLINDRICAL_SURFACE ( 'NONE', #14548, 1.500000000000001554 ) ;
#6860=CIRCLE ( 'NONE', #12271, 1.500000000000000000 ) ;
#6861=FACE_OUTER_BOUND ( 'NONE', #5941, .T. ) ;
#6862=DIRECTION ( 'NONE',  ( -0.1566598588826321192, 0.9876526153536342445, 7.798540720466730171E-17 ) ) ;
#6863=VERTEX_POINT ( 'NONE', #7588 ) ;
#6864=DIRECTION ( 'NONE',  ( -0.1566598588826321192, 0.9876526153536342445, 7.798540720466731404E-17 ) ) ;
#6865=DIRECTION ( 'NONE',  ( -0.1566598588826321192, 0.9876526153536342445, 7.798540720466731404E-17 ) ) ;
#6867=ORIENTED_EDGE ( 'NONE', *, *, #149, .T. ) ;
#6868=DIRECTION ( 'NONE',  ( -0.9876526153536336894, -0.1566598588826349503, 0.000000000000000000 ) ) ;
#6869=AXIS2_PLACEMENT_3D ( 'NONE', #11921, #3408, #7701 ) ;
#6870=ORIENTED_EDGE ( 'NONE', *, *, #12537, .F. ) ;
#6871=VERTEX_POINT ( 'NONE', #14600 ) ;
#6872=EDGE_LOOP ( 'NONE', ( #11162, #9996 ) ) ;
#6873=DIRECTION ( 'NONE',  ( -0.1566598588826321747, 0.9876526153536343555, 0.000000000000000000 ) ) ;
#6874=EDGE_CURVE ( 'NONE', #4290, #2224, #3384, .T. ) ;
#6875=CARTESIAN_POINT ( 'NONE',  ( -31.68662391746666884, -82.98133501614299234, -21.65063509461098690 ) ) ;
#6876=EDGE_CURVE ( 'NONE', #16997, #15396, #17665, .T. ) ;
#6877=AXIS2_PLACEMENT_3D ( 'NONE', #15519, #2535, #8321 ) ;
#6878=CARTESIAN_POINT ( 'NONE',  ( -25.59598991458226536, -19.24727149084832334, 1.908195823574487804E-14 ) ) ;
#6879=EDGE_CURVE ( 'NONE', #10372, #16881, #9888, .T. ) ;
#6880=ADVANCED_FACE ( 'NONE', ( #3289 ), #13354, .F. ) ;
#6881=LINE ( 'NONE', #5445, #2705 ) ;
#6883=PRODUCT_CONTEXT ( 'NONE', #7500, 'mechanical' ) ;
#6884=EDGE_CURVE ( 'NONE', #17521, #15703, #14735, .T. ) ;
#6885=CARTESIAN_POINT ( 'NONE',  ( -44.07191661956487394, -27.24040181582776299, 21.65063509461101887 ) ) ;
#6886=CARTESIAN_POINT ( 'NONE',  ( -10.94591899504043830, -79.69147797960773971, 17.32050807568880657 ) ) ;
#6887=CARTESIAN_POINT ( 'NONE',  ( -62.63296299034337977, -25.12201619894701921, 21.65063509461101887 ) ) ;
#6888=CARTESIAN_POINT ( 'NONE',  ( -42.38608437559395981, -21.91048909185305860, -17.32050807568878170 ) ) ;
#6889=EDGE_LOOP ( 'NONE', ( #14349, #9083 ) ) ;
#6890=ORIENTED_EDGE ( 'NONE', *, *, #2261, .F. ) ;
#6891=CARTESIAN_POINT ( 'NONE',  ( -6.830590222863280658, -16.27073417207831696, -12.99038105676658006 ) ) ;
#6892=DIRECTION ( 'NONE',  ( -0.1566598588826321192, 0.9876526153536342445, 7.798540720466730171E-17 ) ) ;
#6893=CIRCLE ( 'NONE', #4441, 1.500000000000000888 ) ;
#6894=VERTEX_POINT ( 'NONE', #8820 ) ;
#6895=CIRCLE ( 'NONE', #12602, 1.500000000000000444 ) ;
#6896=ORIENTED_EDGE ( 'NONE', *, *, #15184, .T. ) ;
#6898=CIRCLE ( 'NONE', #6285, 1.500000000000000888 ) ;
#6899=ORIENTED_EDGE ( 'NONE', *, *, #14075, .F. ) ;
#6900=CARTESIAN_POINT ( 'NONE',  ( -60.36818477289978091, -29.82528948739120267, -4.330127018922181215 ) ) ;
#6901=CIRCLE ( 'NONE', #207, 1.500000000000000000 ) ;
#6902=FACE_OUTER_BOUND ( 'NONE', #9213, .T. ) ;
#6903=EDGE_LOOP ( 'NONE', ( #14678, #731 ) ) ;
#6904=CARTESIAN_POINT ( 'NONE',  ( -6.830590222863280658, -16.27073417207831696, -21.65063509461097979 ) ) ;
#6905=CYLINDRICAL_SURFACE ( 'NONE', #8217, 1.500000000000001554 ) ;
#6907=CYLINDRICAL_SURFACE ( 'NONE', #5528, 1.500000000000001554 ) ;
#6909=CIRCLE ( 'NONE', #4156, 1.500000000000000888 ) ;
#6910=EDGE_CURVE ( 'NONE', #13845, #9583, #3205, .T. ) ;
#6911=CARTESIAN_POINT ( 'NONE',  ( 3.231158466157551423, 19.73726462726227737, 30.00000000000000000 ) ) ;
#6912=VERTEX_POINT ( 'NONE', #17562 ) ;
#6913=CARTESIAN_POINT ( 'NONE',  ( -5.842937607509656850, -16.11407431319567962, -8.660254037844383745 ) ) ;
#6914=VECTOR ( 'NONE', #1138, 1000.000000000000000 ) ;
#6915=DIRECTION ( 'NONE',  ( 0.000000000000000000, 0.000000000000000000, 1.000000000000000000 ) ) ;
#6916=VERTEX_POINT ( 'NONE', #11903 ) ;
#6917=ORIENTED_EDGE ( 'NONE', *, *, #14126, .F. ) ;
#6919=EDGE_CURVE ( 'NONE', #7360, #8286, #5657, .T. ) ;
#6920=CARTESIAN_POINT ( 'NONE',  ( -55.39028668595378946, -86.74117162932616054, 1.424741226644455312E-14 ) ) ;
#6923=ORIENTED_EDGE ( 'NONE', *, *, #10688, .F. ) ;
#6925=CARTESIAN_POINT ( 'NONE',  ( -37.15834831208948685, -26.14378280364935137, 4.330127018922217630 ) ) ;
#6926=ORIENTED_EDGE ( 'NONE', *, *, #11211, .T. ) ;
#6928=AXIS2_PLACEMENT_3D ( 'NONE', #3279, #2914, #16006 ) ;
#6929=CARTESIAN_POINT ( 'NONE',  ( -16.70711637639958269, -17.83733276090463704, -12.99038105676658006 ) ) ;
#6930=AXIS2_PLACEMENT_3D ( 'NONE', #1478, #10361, #14820 ) ;
#6932=FACE_OUTER_BOUND ( 'NONE', #6792, .T. ) ;
#6933=DIRECTION ( 'NONE',  ( -0.1566598588826321747, 0.9876526153536343555, 0.000000000000000000 ) ) ;
#6935=AXIS2_PLACEMENT_3D ( 'NONE', #14271, #13975, #11303 ) ;
#6937=DIRECTION ( 'NONE',  ( -0.9876526153536341335, -0.1566598588826327021, 0.000000000000000000 ) ) ;
#6938=LINE ( 'NONE', #3860, #5331 ) ;
#6942=EDGE_CURVE ( 'NONE', #8675, #2583, #10475, .T. ) ;
#6945=DIRECTION ( 'NONE',  ( -0.1566598588826321192, 0.9876526153536342445, 7.798540720466730171E-17 ) ) ;
#6946=AXIS2_PLACEMENT_3D ( 'NONE', #7148, #8366, #8652 ) ;
#6947=ORIENTED_EDGE ( 'NONE', *, *, #17202, .F. ) ;
#6948=EDGE_CURVE ( 'NONE', #17749, #6040, #11965, .T. ) ;
#6949=DIRECTION ( 'NONE',  ( 0.000000000000000000, 0.000000000000000000, 1.000000000000000000 ) ) ;
#6950=AXIS2_PLACEMENT_3D ( 'NONE', #15037, #554, #3275 ) ;
#6951=AXIS2_PLACEMENT_3D ( 'NONE', #11018, #15960, #17222 ) ;
#6952=FACE_BOUND ( 'NONE', #1581, .T. ) ;
#6953=AXIS2_PLACEMENT_3D ( 'NONE', #16028, #3038, #6955 ) ;
#6954=AXIS2_PLACEMENT_3D ( 'NONE', #7988, #13847, #13749 ) ;
#6955=DIRECTION ( 'NONE',  ( 1.000000000000000000, 0.000000000000000000, 0.000000000000000000 ) ) ;
#6956=DIRECTION ( 'NONE',  ( 0.000000000000000000, 0.000000000000000000, 1.000000000000000000 ) ) ;
#6957=ORIENTED_EDGE ( 'NONE', *, *, #7845, .F. ) ;
#6958=FACE_BOUND ( 'NONE', #7399, .T. ) ;
#6959=ORIENTED_EDGE ( 'NONE', *, *, #2803, .T. ) ;
#6962=CIRCLE ( 'NONE', #2093, 1.500000000000000000 ) ;
#6963=AXIS2_PLACEMENT_3D ( 'NONE', #2897, #11424, #17257 ) ;
#6964=CYLINDRICAL_SURFACE ( 'NONE', #1254, 1.500000000000001554 ) ;
#6965=LINE ( 'NONE', #13949, #18478 ) ;
#6966=EDGE_CURVE ( 'NONE', #495, #1369, #12745, .T. ) ;
#6968=ADVANCED_FACE ( 'NONE', ( #5563 ), #11028, .F. ) ;
#6969=ORIENTED_EDGE ( 'NONE', *, *, #14374, .F. ) ;
#6970=EDGE_CURVE ( 'NONE', #7134, #7610, #18553, .T. ) ;
#6971=ORIENTED_EDGE ( 'NONE', *, *, #14943, .T. ) ;
#6972=AXIS2_PLACEMENT_3D ( 'NONE', #1695, #11808, #17736 ) ;
#6973=ORIENTED_EDGE ( 'NONE', *, *, #1147, .F. ) ;
#6974=CARTESIAN_POINT ( 'NONE',  ( -75.18297400320422241, -32.17518737063066681, -12.99038105676658006 ) ) ;
#6976=CARTESIAN_POINT ( 'NONE',  ( -18.39294862037050393, -23.16724548487935564, 17.32050807568881012 ) ) ;
#6977=DIRECTION ( 'NONE',  ( -0.1566598588826321192, 0.9876526153536342445, 7.798540720466730171E-17 ) ) ;
#6979=AXIS2_PLACEMENT_3D ( 'NONE', #8434, #14108, #1252 ) ;
#6980=CARTESIAN_POINT ( 'NONE',  ( -18.35331361019266794, -80.86642692122747178, -21.65063509461098690 ) ) ;
#6982=DIRECTION ( 'NONE',  ( -0.1566598588826321192, 0.9876526153536342445, 7.798540720466730171E-17 ) ) ;
#6984=CARTESIAN_POINT ( 'NONE',  ( -2.096680467035594297, -20.58235781331593017, 17.32050807568881012 ) ) ;
#6987=EDGE_CURVE ( 'NONE', #4041, #405, #2524, .T. ) ;
#6989=CIRCLE ( 'NONE', #9699, 1.500000000000000888 ) ;
#6990=FACE_OUTER_BOUND ( 'NONE', #11626, .T. ) ;
#6991=ADVANCED_FACE ( 'NONE', ( #4109 ), #15684, .F. ) ;
#6992=DIRECTION ( 'NONE',  ( -0.1566598588826321747, 0.9876526153536343555, 0.000000000000000000 ) ) ;
#6994=EDGE_CURVE ( 'NONE', #10517, #13155, #1039, .T. ) ;
#6995=EDGE_LOOP ( 'NONE', ( #3194, #1957 ) ) ;
#6996=ORIENTED_EDGE ( 'NONE', *, *, #909, .F. ) ;
#6997=FACE_BOUND ( 'NONE', #14198, .T. ) ;
#6998=DIRECTION ( 'NONE',  ( -0.1566598588826321747, 0.9876526153536343555, 0.000000000000000000 ) ) ;
#6999=ORIENTED_EDGE ( 'NONE', *, *, #5217, .T. ) ;
#7003=CIRCLE ( 'NONE', #9985, 1.500000000000000888 ) ;
#7004=AXIS2_PLACEMENT_3D ( 'NONE', #560, #17471, #2064 ) ;
#7005=DIRECTION ( 'NONE',  ( -0.1566598588826321192, 0.9876526153536342445, 7.798540720466731404E-17 ) ) ;
#7006=ORIENTED_EDGE ( 'NONE', *, *, #12572, .T. ) ;
#7007=AXIS2_PLACEMENT_3D ( 'NONE', #17388, #7237, #5820 ) ;
#7010=CIRCLE ( 'NONE', #17608, 1.500000000000000000 ) ;
#7011=DIRECTION ( 'NONE',  ( -0.1566598588826321747, 0.9876526153536343555, 0.000000000000000000 ) ) ;
#7012=AXIS2_PLACEMENT_3D ( 'NONE', #4591, #18680, #4404 ) ;
#7013=LINE ( 'NONE', #6911, #16951 ) ;
#7015=FACE_OUTER_BOUND ( 'NONE', #9447, .T. ) ;
#7016=AXIS2_PLACEMENT_3D ( 'NONE', #6904, #12643, #18504 ) ;
#7019=ORIENTED_EDGE ( 'NONE', *, *, #12476, .F. ) ;
#7020=CARTESIAN_POINT ( 'NONE',  ( -48.80582637539257718, -22.92877817459016043, -17.32050807568878170 ) ) ;
#7021=DIRECTION ( 'NONE',  ( -0.1566598588826321747, 0.9876526153536343555, 0.000000000000000000 ) ) ;
#7022=VERTEX_POINT ( 'NONE', #18303 ) ;
#7023=DIRECTION ( 'NONE',  ( 0.000000000000000000, 0.000000000000000000, 1.000000000000000000 ) ) ;
#7024=ORIENTED_EDGE ( 'NONE', *, *, #3448, .F. ) ;
#7025=ORIENTED_EDGE ( 'NONE', *, *, #9830, .T. ) ;
#7027=EDGE_CURVE ( 'NONE', #5678, #15183, #8312, .T. ) ;
#7028=CARTESIAN_POINT ( 'NONE',  ( -59.83472345504510770, -87.44614099429800547, 21.65063509461101532 ) ) ;
#7030=VECTOR ( 'NONE', #449, 1000.000000000000000 ) ;
#7031=EDGE_CURVE ( 'NONE', #9513, #12208, #14074, .T. ) ;
#7033=EDGE_LOOP ( 'NONE', ( #6045, #7245 ) ) ;
#7034=CARTESIAN_POINT ( 'NONE',  ( -24.27922930231443743, -81.80638607452326028, 1.424741226644455312E-14 ) ) ;
#7035=DIRECTION ( 'NONE',  ( -0.1566598588826321747, 0.9876526153536343555, 0.000000000000000000 ) ) ;
#7038=CARTESIAN_POINT ( 'NONE',  ( -54.44226908077801141, -28.88533033409540351, 8.660254037844417496 ) ) ;
#7039=CARTESIAN_POINT ( 'NONE',  ( -76.66445292623467367, -32.41017715895461038, -12.99038105676658006 ) ) ;
#7040=FACE_OUTER_BOUND ( 'NONE', #2708, .T. ) ;
#7042=AXIS2_PLACEMENT_3D ( 'NONE', #14871, #11723, #17836 ) ;
#7044=LINE ( 'NONE', #12789, #10792 ) ;
#7048=FACE_OUTER_BOUND ( 'NONE', #17667, .T. ) ;
#7049=ORIENTED_EDGE ( 'NONE', *, *, #5461, .T. ) ;
#7051=CARTESIAN_POINT ( 'NONE',  ( -53.74408945216072198, -23.71207746900332225, -8.660254037844380193 ) ) ;
#7052=FACE_BOUND ( 'NONE', #3040, .T. ) ;
#7054=EDGE_CURVE ( 'NONE', #10692, #17807, #2709, .T. ) ;
#7055=DIRECTION ( 'NONE',  ( 0.000000000000000000, 0.000000000000000000, 1.000000000000000000 ) ) ;
#7056=ORIENTED_EDGE ( 'NONE', *, *, #8959, .F. ) ;
#7058=CARTESIAN_POINT ( 'NONE',  ( -31.52190560670403841, -20.18723064414410828, -12.99038105676658006 ) ) ;
#7059=EDGE_CURVE ( 'NONE', #9193, #9534, #332, .T. ) ;
#7060=ORIENTED_EDGE ( 'NONE', *, *, #13715, .F. ) ;
#7061=AXIS2_PLACEMENT_3D ( 'NONE', #2008, #13551, #4931 ) ;
#7062=DIRECTION ( 'NONE',  ( -0.9876526153536341335, -0.1566598588826327021, 0.000000000000000000 ) ) ;
#7063=DIRECTION ( 'NONE',  ( 0.000000000000000000, 0.000000000000000000, 1.000000000000000000 ) ) ;
#7064=DIRECTION ( 'NONE',  ( -0.1566598588826321192, 0.9876526153536342445, 7.798540720466730171E-17 ) ) ;
#7065=DIRECTION ( 'NONE',  ( 0.000000000000000000, 0.000000000000000000, 1.000000000000000000 ) ) ;
#7066=FACE_BOUND ( 'NONE', #18470, .T. ) ;
#7067=DIRECTION ( 'NONE',  ( -0.9876526153536341335, -0.1566598588826327021, 0.000000000000000000 ) ) ;
#7072=CARTESIAN_POINT ( 'NONE',  ( 55.85952145814821534, 6.938893903907228378E-15, -24.99999999999999289 ) ) ;
#7073=EDGE_LOOP ( 'NONE', ( #12749, #10474, #470, #9876 ) ) ;
#7074=ORIENTED_EDGE ( 'NONE', *, *, #2995, .T. ) ;
#7076=CARTESIAN_POINT ( 'NONE',  ( 3.868870235264020963, -77.34158009636824715, 1.077796531449093893E-14 ) ) ;
#7078=EDGE_CURVE ( 'NONE', #9210, #17772, #17313, .T. ) ;
#7079=CYLINDRICAL_SURFACE ( 'NONE', #10574, 1.500000000000001554 ) ;
#7080=CARTESIAN_POINT ( 'NONE',  ( -75.96627329761737712, -27.23692429386253977, 4.330127018922218518 ) ) ;
#7081=EDGE_CURVE ( 'NONE', #17878, #14934, #18540, .T. ) ;
#7082=DIRECTION ( 'NONE',  ( -0.1566598588826321192, 0.9876526153536342445, 7.798540720466730171E-17 ) ) ;
#7083=DIRECTION ( 'NONE',  ( -0.1566598588826321192, 0.9876526153536342445, 7.798540720466730171E-17 ) ) ;
#7084=DIRECTION ( 'NONE',  ( -0.1566598588826321192, 0.9876526153536342445, 7.798540720466730171E-17 ) ) ;
#7085=DIRECTION ( 'NONE',  ( 0.000000000000000000, 0.000000000000000000, 1.000000000000000000 ) ) ;
#7086=ORIENTED_EDGE ( 'NONE', *, *, #4861, .F. ) ;
#7087=ORIENTED_EDGE ( 'NONE', *, *, #1244, .T. ) ;
#7088=CIRCLE ( 'NONE', #4326, 1.500000000000000888 ) ;
#7089=LINE ( 'NONE', #12461, #5160 ) ;
#7091=CARTESIAN_POINT ( 'NONE',  ( -58.84707083969148300, -87.28948113541537168, 1.424741226644455312E-14 ) ) ;
#7092=VERTEX_POINT ( 'NONE', #13883 ) ;
#7093=EDGE_CURVE ( 'NONE', #10493, #202, #9637, .T. ) ;
#7094=ORIENTED_EDGE ( 'NONE', *, *, #13085, .T. ) ;
#7095=CYLINDRICAL_SURFACE ( 'NONE', #13939, 1.500000000000001554 ) ;
#7096=ADVANCED_FACE ( 'NONE', ( #18398 ), #5468, .F. ) ;
#7097=DIRECTION ( 'NONE',  ( -0.1566598588826321192, 0.9876526153536342445, 7.798540720466730171E-17 ) ) ;
#7098=EDGE_CURVE ( 'NONE', #272, #2139, #8812, .T. ) ;
#7099=EDGE_CURVE ( 'NONE', #6259, #13724, #2136, .T. ) ;
#7100=DIRECTION ( 'NONE',  ( -0.1566598588826321747, 0.9876526153536343555, 0.000000000000000000 ) ) ;
#7102=DIRECTION ( 'NONE',  ( -0.9876526153536336894, -0.1566598588826349503, 0.000000000000000000 ) ) ;
#7104=EDGE_CURVE ( 'NONE', #15556, #6894, #13026, .T. ) ;
#7108=CYLINDRICAL_SURFACE ( 'NONE', #5952, 1.500000000000001554 ) ;
#7109=CARTESIAN_POINT ( 'NONE',  ( -67.73594437787414790, -88.69941986535906153, -12.99038105676658539 ) ) ;
#7110=EDGE_LOOP ( 'NONE', ( #14339, #6451, #5368, #7679 ) ) ;
#7111=FACE_OUTER_BOUND ( 'NONE', #12997, .T. ) ;
#7112=DIRECTION ( 'NONE',  ( -0.1566598588826321192, 0.9876526153536342445, 7.798540720466731404E-17 ) ) ;
#7113=CARTESIAN_POINT ( 'NONE',  ( -72.01566283620284992, -26.61028485833202240, 17.32050807568881723 ) ) ;
#7114=EDGE_LOOP ( 'NONE', ( #4335, #16149 ) ) ;
#7115=ORIENTED_EDGE ( 'NONE', *, *, #11659, .F. ) ;
#7116=ORIENTED_EDGE ( 'NONE', *, *, #1372, .F. ) ;
#7117=CARTESIAN_POINT ( 'NONE',  ( 1.893565004556770903, -77.65489981413351472, -17.32050807568878525 ) ) ;
#7118=EDGE_CURVE ( 'NONE', #17282, #10247, #63, .T. ) ;
#7121=CYLINDRICAL_SURFACE ( 'NONE', #10925, 1.500000000000001554 ) ;
#7123=CARTESIAN_POINT ( 'NONE',  ( -66.29410046502154330, -30.76524864068697696, -17.32050807568878170 ) ) ;
#7125=FACE_BOUND ( 'NONE', #6872, .T. ) ;
#7126=ADVANCED_FACE ( 'NONE', ( #16073 ), #7095, .F. ) ;
#7127=CIRCLE ( 'NONE', #3153, 1.500000000000000888 ) ;
#7128=ORIENTED_EDGE ( 'NONE', *, *, #17030, .F. ) ;
#7129=EDGE_LOOP ( 'NONE', ( #8561, #9311, #18308, #5433 ) ) ;
#7130=FACE_OUTER_BOUND ( 'NONE', #12820, .T. ) ;
#7131=ORIENTED_EDGE ( 'NONE', *, *, #11680, .F. ) ;
#7132=ORIENTED_EDGE ( 'NONE', *, *, #8627, .T. ) ;
#7133=CARTESIAN_POINT ( 'NONE',  ( -51.43967622453926936, -86.11453219379563961, 4.330127018922213189 ) ) ;
#7134=VERTEX_POINT ( 'NONE', #3076 ) ;
#7135=CARTESIAN_POINT ( 'NONE',  ( 10.28861223506262412, -76.32329101363113466, 17.32050807568880657 ) ) ;
#7136=FACE_BOUND ( 'NONE', #17729, .T. ) ;
#7137=DIRECTION ( 'NONE',  ( 0.000000000000000000, 0.000000000000000000, 1.000000000000000000 ) ) ;
#7138=AXIS2_PLACEMENT_3D ( 'NONE', #17124, #18486, #16753 ) ;
#7139=ORIENTED_EDGE ( 'NONE', *, *, #890, .T. ) ;
#7140=DIRECTION ( 'NONE',  ( -0.9876526153536336894, -0.1566598588826349503, 0.000000000000000000 ) ) ;
#7141=FACE_BOUND ( 'NONE', #9438, .T. ) ;
#7142=EDGE_CURVE ( 'NONE', #4359, #7782, #11215, .T. ) ;
#7143=ORIENTED_EDGE ( 'NONE', *, *, #18681, .T. ) ;
#7144=DIRECTION ( 'NONE',  ( -0.1566598588826321192, 0.9876526153536342445, 7.798540720466731404E-17 ) ) ;
#7145=DIRECTION ( 'NONE',  ( -0.9876526153536336894, -0.1566598588826349503, 0.000000000000000000 ) ) ;
#7147=EDGE_LOOP ( 'NONE', ( #1967, #10211 ) ) ;
#7148=CARTESIAN_POINT ( 'NONE',  ( 0.5768043922889515285, -15.09578523045857601, -8.660254037844383745 ) ) ;
#7149=EDGE_CURVE ( 'NONE', #6686, #18200, #10898, .T. ) ;
#7150=VECTOR ( 'NONE', #11090, 1000.000000000000000 ) ;
#7151=ORIENTED_EDGE ( 'NONE', *, *, #10376, .T. ) ;
#7152=ORIENTED_EDGE ( 'NONE', *, *, #17460, .T. ) ;
#7153=ORIENTED_EDGE ( 'NONE', *, *, #1649, .F. ) ;
#7154=DIRECTION ( 'NONE',  ( -0.1566598588826321192, 0.9876526153536342445, 7.798540720466731404E-17 ) ) ;
#7155=ORIENTED_EDGE ( 'NONE', *, *, #1735, .F. ) ;
#7156=VERTEX_POINT ( 'NONE', #11596 ) ;
#7157=FACE_BOUND ( 'NONE', #15765, .T. ) ;
#7158=DIRECTION ( 'NONE',  ( -0.1566598588826321192, 0.9876526153536342445, 7.798540720466730171E-17 ) ) ;
#7159=CIRCLE ( 'NONE', #7452, 1.500000000000000888 ) ;
#7160=CARTESIAN_POINT ( 'NONE',  ( -0.5755665338273089349, -78.04654946134009208, -4.330127018922185655 ) ) ;
#7161=CARTESIAN_POINT ( 'NONE',  ( -10.78120068427780964, -16.89737360760884144, 17.32050807568881012 ) ) ;
#7162=DIRECTION ( 'NONE',  ( -0.1566598588826321192, 0.9876526153536342445, 7.798540720466731404E-17 ) ) ;
#7163=DIRECTION ( 'NONE',  ( -0.1566598588826321192, 0.9876526153536342445, 7.798540720466730171E-17 ) ) ;
#7164=ORIENTED_EDGE ( 'NONE', *, *, #22, .F. ) ;
#7166=CARTESIAN_POINT ( 'NONE',  ( -70.24471092643608472, -31.39188807621751209, 4.330127018922217630 ) ) ;
#7168=CYLINDRICAL_SURFACE ( 'NONE', #6530, 1.500000000000001554 ) ;
#7169=EDGE_LOOP ( 'NONE', ( #9140, #366 ) ) ;
#7171=DIRECTION ( 'NONE',  ( -0.9876526153536336894, -0.1566598588826349503, 0.000000000000000000 ) ) ;
#7172=CIRCLE ( 'NONE', #6869, 1.500000000000000000 ) ;
#7174=DIRECTION ( 'NONE',  ( -0.9876526153536336894, -0.1566598588826349503, 0.000000000000000000 ) ) ;
#7176=AXIS2_PLACEMENT_3D ( 'NONE', #9911, #8609, #15695 ) ;
#7177=ORIENTED_EDGE ( 'NONE', *, *, #15412, .T. ) ;
#7178=CARTESIAN_POINT ( 'NONE',  ( -63.78533391645962780, -88.07278042982852639, 1.424741226644455312E-14 ) ) ;
#7179=EDGE_CURVE ( 'NONE', #13174, #9184, #6703, .T. ) ;
#7180=ORIENTED_EDGE ( 'NONE', *, *, #10884, .F. ) ;
#7181=DIRECTION ( 'NONE',  ( -0.9876526153536341335, -0.1566598588826327021, 0.000000000000000000 ) ) ;
#7182=DIRECTION ( 'NONE',  ( -0.1566598588826321192, 0.9876526153536342445, 7.798540720466731404E-17 ) ) ;
#7183=AXIS2_PLACEMENT_3D ( 'NONE', #186, #14775, #16406 ) ;
#7184=DIRECTION ( 'NONE',  ( -0.1566598588826321192, 0.9876526153536342445, 7.798540720466731404E-17 ) ) ;
#7185=DIRECTION ( 'NONE',  ( -0.1566598588826321192, 0.9876526153536342445, 7.798540720466731404E-17 ) ) ;
#7187=CYLINDRICAL_SURFACE ( 'NONE', #589, 1.500000000000001554 ) ;
#7188=AXIS2_PLACEMENT_3D ( 'NONE', #7454, #4876, #16366 ) ;
#7189=EDGE_CURVE ( 'NONE', #9493, #16874, #9107, .T. ) ;
#7190=DIRECTION ( 'NONE',  ( 0.000000000000000000, 0.000000000000000000, 1.000000000000000000 ) ) ;
#7191=AXIS2_PLACEMENT_3D ( 'NONE', #10403, #11987, #382 ) ;
#7192=FACE_OUTER_BOUND ( 'NONE', #36, .T. ) ;
#7193=CARTESIAN_POINT ( 'NONE',  ( -28.06512145296634486, -19.63892113805489359, -21.65063509461098334 ) ) ;
#7194=EDGE_LOOP ( 'NONE', ( #10891, #17833, #2504, #2736 ) ) ;
#7195=VERTEX_POINT ( 'NONE', #11406 ) ;
#7196=CARTESIAN_POINT ( 'NONE',  ( -39.62747985047355570, -26.53543245085592517, 1.175313729581431390E-14 ) ) ;
#7197=VECTOR ( 'NONE', #16186, 1000.000000000000000 ) ;
#7198=DIRECTION ( 'NONE',  ( -0.9876526153536336894, -0.1566598588826349503, 0.000000000000000000 ) ) ;
#7199=EDGE_LOOP ( 'NONE', ( #1626, #6356, #805, #4962 ) ) ;
#7200=ORIENTED_EDGE ( 'NONE', *, *, #10771, .F. ) ;
#7202=EDGE_CURVE ( 'NONE', #3195, #13266, #11507, .T. ) ;
#7203=ADVANCED_FACE ( 'NONE', ( #11770 ), #5928, .F. ) ;
#7204=ORIENTED_EDGE ( 'NONE', *, *, #9408, .F. ) ;
#7205=EDGE_LOOP ( 'NONE', ( #10066, #2824, #5606, #3944 ) ) ;
#7206=EDGE_CURVE ( 'NONE', #9188, #15855, #2456, .T. ) ;
#7207=AXIS2_PLACEMENT_3D ( 'NONE', #4005, #9808, #1300 ) ;
#7209=DIRECTION ( 'NONE',  ( -0.9876526153536336894, -0.1566598588826349503, 0.000000000000000000 ) ) ;
#7211=FACE_OUTER_BOUND ( 'NONE', #16378, .T. ) ;
#7212=DIRECTION ( 'NONE',  ( -0.1566598588826321192, 0.9876526153536342445, 7.798540720466730171E-17 ) ) ;
#7213=EDGE_LOOP ( 'NONE', ( #6467, #15 ) ) ;
#7214=DIRECTION ( 'NONE',  ( -0.1566598588826321192, 0.9876526153536342445, 7.798540720466730171E-17 ) ) ;
#7215=CARTESIAN_POINT ( 'NONE',  ( -5.513829610595458064, -78.82984875575326100, 4.330127018922213189 ) ) ;
#7216=CARTESIAN_POINT ( 'NONE',  ( -9.504075082187823043, -21.75730675493566579, 12.99038105676661381 ) ) ;
#7217=CARTESIAN_POINT ( 'NONE',  ( 4.362696542940843081, -77.26325016692693737, -21.65063509461098690 ) ) ;
#7218=CARTESIAN_POINT ( 'NONE',  ( -70.24471092643608472, -31.39188807621751209, -12.99038105676658006 ) ) ;
#7220=CARTESIAN_POINT ( 'NONE',  ( -4.361458684479201153, -15.87908452487173427, -8.660254037844383745 ) ) ;
#7221=DIRECTION ( 'NONE',  ( -0.1566598588826321192, 0.9876526153536342445, 7.798540720466730171E-17 ) ) ;
#7222=ORIENTED_EDGE ( 'NONE', *, *, #6505, .T. ) ;
#7224=ORIENTED_EDGE ( 'NONE', *, *, #3378, .F. ) ;
#7225=LINE ( 'NONE', #12971, #275 ) ;
#7226=ORIENTED_EDGE ( 'NONE', *, *, #15478, .T. ) ;
#7227=ORIENTED_EDGE ( 'NONE', *, *, #1018, .F. ) ;
#7228=CARTESIAN_POINT ( 'NONE',  ( -52.75643683680709728, -23.55541761012068491, -21.65063509461098334 ) ) ;
#7229=AXIS2_PLACEMENT_3D ( 'NONE', #10682, #15042, #6447 ) ;
#7230=CARTESIAN_POINT ( 'NONE',  ( -7.982961148979534016, -79.22149840295983836, 17.32050807568880657 ) ) ;
#7231=AXIS2_PLACEMENT_3D ( 'NONE', #12401, #12106, #4822 ) ;
#7233=AXIS2_PLACEMENT_3D ( 'NONE', #7872, #11911, #3486 ) ;
#7234=DIRECTION ( 'NONE',  ( -0.1566598588826321192, 0.9876526153536342445, 7.798540720466731404E-17 ) ) ;
#7235=FACE_BOUND ( 'NONE', #16449, .T. ) ;
#7236=EDGE_LOOP ( 'NONE', ( #1678, #9793 ) ) ;
#7237=DIRECTION ( 'NONE',  ( -0.1566598588826321747, 0.9876526153536343555, 0.000000000000000000 ) ) ;
#7238=CARTESIAN_POINT ( 'NONE',  ( -47.48906576312474215, -85.48789275826510448, -8.660254037844385522 ) ) ;
#7240=DIRECTION ( 'NONE',  ( -1.000000000000000000, 0.000000000000000000, 0.000000000000000000 ) ) ;
#7241=AXIS2_PLACEMENT_3D ( 'NONE', #16622, #17696, #4664 ) ;
#7242=ORIENTED_EDGE ( 'NONE', *, *, #1522, .T. ) ;
#7243=( GEOMETRIC_REPRESENTATION_CONTEXT ( 3 ) GLOBAL_UNCERTAINTY_ASSIGNED_CONTEXT ( ( #6080 ) ) GLOBAL_UNIT_ASSIGNED_CONTEXT ( ( #10952, #3739, #15319 ) ) REPRESENTATION_CONTEXT ( 'NONE', 'WORKASPACE' ) );
#7244=ORIENTED_EDGE ( 'NONE', *, *, #4293, .T. ) ;
#7245=ORIENTED_EDGE ( 'NONE', *, *, #1244, .F. ) ;
#7246=CYLINDRICAL_SURFACE ( 'NONE', #3063, 1.500000000000001554 ) ;
#7247=VERTEX_POINT ( 'NONE', #9997 ) ;
#7248=LINE ( 'NONE', #11743, #4581 ) ;
#7249=EDGE_CURVE ( 'NONE', #8900, #17816, #15154, .T. ) ;
#7250=AXIS2_PLACEMENT_3D ( 'NONE', #4174, #7234, #12982 ) ;
#7251=LINE ( 'NONE', #43, #3595 ) ;
#7252=ADVANCED_FACE ( 'NONE', ( #5849 ), #17334, .F. ) ;
#7253=ORIENTED_EDGE ( 'NONE', *, *, #10015, .T. ) ;
#7255=EDGE_CURVE ( 'NONE', #12715, #14620, #2880, .T. ) ;
#7256=VECTOR ( 'NONE', #17657, 1000.000000000000000 ) ;
#7258=LINE ( 'NONE', #8855, #18265 ) ;
#7260=DIRECTION ( 'NONE',  ( -0.9876526153536344665, -0.1566598588826304539, 0.000000000000000000 ) ) ;
#7261=DIRECTION ( 'NONE',  ( 3.208277787129350839E-17, 0.000000000000000000, -1.000000000000000000 ) ) ;
#7262=VECTOR ( 'NONE', #1291, 1000.000000000000000 ) ;
#7264=CYLINDRICAL_SURFACE ( 'NONE', #5372, 1.500000000000001554 ) ;
#7265=ORIENTED_EDGE ( 'NONE', *, *, #5588, .T. ) ;
#7266=ORIENTED_EDGE ( 'NONE', *, *, #10730, .F. ) ;
#7267=CARTESIAN_POINT ( 'NONE',  ( 0.000000000000000000, 0.000000000000000000, 30.00000000000000000 ) ) ;
#7269=CARTESIAN_POINT ( 'NONE',  ( -6.007655918272284623, -78.90817868519457079, 17.32050807568880657 ) ) ;
#7270=DIRECTION ( 'NONE',  ( -0.1566598588826321192, 0.9876526153536342445, 7.798540720466731404E-17 ) ) ;
#7271=AXIS2_PLACEMENT_3D ( 'NONE', #17822, #16675, #12270 ) ;
#7272=CIRCLE ( 'NONE', #17872, 1.500000000000000444 ) ;
#7276=DIRECTION ( 'NONE',  ( 1.000000000000000000, 0.000000000000000000, 0.000000000000000000 ) ) ;
#7278=CIRCLE ( 'NONE', #17891, 1.500000000000000444 ) ;
#7280=DIRECTION ( 'NONE',  ( -1.000000000000000000, 0.000000000000000000, 0.000000000000000000 ) ) ;
#7282=VERTEX_POINT ( 'NONE', #14459 ) ;
#7283=AXIS2_PLACEMENT_3D ( 'NONE', #9729, #9522, #17036 ) ;
#7284=FACE_OUTER_BOUND ( 'NONE', #7995, .T. ) ;
#7285=VECTOR ( 'NONE', #1212, 1000.000000000000000 ) ;
#7286=EDGE_LOOP ( 'NONE', ( #16445, #12100 ) ) ;
#7287=CYLINDRICAL_SURFACE ( 'NONE', #11961, 1.500000000000001554 ) ;
#7290=ORIENTED_EDGE ( 'NONE', *, *, #316, .T. ) ;
#7291=ORIENTED_EDGE ( 'NONE', *, *, #8427, .F. ) ;
#7294=VERTEX_POINT ( 'NONE', #10458 ) ;
#7295=CARTESIAN_POINT ( 'NONE',  ( -53.74408945216069355, -23.71207746900333291, 17.32050807568882078 ) ) ;
#7296=CIRCLE ( 'NONE', #4548, 144.0000000000000284 ) ;
#7297=ORIENTED_EDGE ( 'NONE', *, *, #5125, .T. ) ;
#7299=ORIENTED_EDGE ( 'NONE', *, *, #6366, .T. ) ;
#7300=CIRCLE ( 'NONE', #15457, 1.500000000000000444 ) ;
#7301=DIRECTION ( 'NONE',  ( -0.9876526153536341335, -0.1566598588826327021, 0.000000000000000000 ) ) ;
#7302=DIRECTION ( 'NONE',  ( -0.9876526153536341335, -0.1566598588826327021, 0.000000000000000000 ) ) ;
#7304=CARTESIAN_POINT ( 'NONE',  ( -70.04035760549561473, -26.29696514056675127, 8.660254037844417496 ) ) ;
#7305=DIRECTION ( 'NONE',  ( -0.9876526153536341335, -0.1566598588826327021, 0.000000000000000000 ) ) ;
#7307=AXIS2_PLACEMENT_3D ( 'NONE', #808, #6694, #13676 ) ;
#7308=EDGE_CURVE ( 'NONE', #17245, #15425, #7724, .T. ) ;
#7309=CARTESIAN_POINT ( 'NONE',  ( -24.11451099155181055, -19.01228170252437266, -17.32050807568878170 ) ) ;
#7310=ORIENTED_EDGE ( 'NONE', *, *, #8193, .T. ) ;
#7311=DIRECTION ( 'NONE',  ( 0.000000000000000000, 0.000000000000000000, 1.000000000000000000 ) ) ;
#7312=EDGE_CURVE ( 'NONE', #3161, #4161, #17622, .T. ) ;
#7313=CARTESIAN_POINT ( 'NONE',  ( -17.40529600501688279, -23.01058562599671831, 4.330127018922217630 ) ) ;
#7315=CARTESIAN_POINT ( 'NONE',  ( -45.55339554259532520, -27.47539160415171722, 12.99038105676661736 ) ) ;
#7316=ORIENTED_EDGE ( 'NONE', *, *, #16792, .T. ) ;
#7317=AXIS2_PLACEMENT_3D ( 'NONE', #7367, #15794, #5759 ) ;
#7320=DIRECTION ( 'NONE',  ( -0.1566598588826321192, 0.9876526153536342445, 7.798540720466730171E-17 ) ) ;
#7321=EDGE_LOOP ( 'NONE', ( #3043, #8917, #11629, #15748 ) ) ;
#7322=ORIENTED_EDGE ( 'NONE', *, *, #2633, .F. ) ;
#7323=ORIENTED_EDGE ( 'NONE', *, *, #8041, .T. ) ;
#7324=DIRECTION ( 'NONE',  ( -0.1566598588826321192, 0.9876526153536342445, 7.798540720466730171E-17 ) ) ;
#7325=DIRECTION ( 'NONE',  ( -0.1566598588826321192, 0.9876526153536342445, 7.798540720466730171E-17 ) ) ;
#7326=ORIENTED_EDGE ( 'NONE', *, *, #11096, .F. ) ;
#7327=AXIS2_PLACEMENT_3D ( 'NONE', #16830, #8370, #10813 ) ;
#7328=CARTESIAN_POINT ( 'NONE',  ( -51.27495791377661760, -23.32042782179675555, 21.65063509461102242 ) ) ;
#7330=CIRCLE ( 'NONE', #13348, 1.499999999999999556 ) ;
#7331=EDGE_CURVE ( 'NONE', #14760, #13568, #15167, .T. ) ;
#7332=EDGE_CURVE ( 'NONE', #6192, #7092, #7814, .T. ) ;
#7333=LINE ( 'NONE', #9380, #313 ) ;
#7334=CARTESIAN_POINT ( 'NONE',  ( -21.81009776393036503, -81.41473642731666871, -21.65063509461098690 ) ) ;
#7335=ORIENTED_EDGE ( 'NONE', *, *, #7613, .F. ) ;
#7337=CIRCLE ( 'NONE', #14439, 1.500000000000000444 ) ;
#7338=AXIS2_PLACEMENT_3D ( 'NONE', #11084, #16909, #17006 ) ;
#7340=CARTESIAN_POINT ( 'NONE',  ( -10.98555400521827963, -21.99229654325962002, -21.65063509461098334 ) ) ;
#7341=FACE_OUTER_BOUND ( 'NONE', #16762, .T. ) ;
#7342=ORIENTED_EDGE ( 'NONE', *, *, #6023, .T. ) ;
#7343=CIRCLE ( 'NONE', #11827, 1.499999999999999556 ) ;
#7344=ORIENTED_EDGE ( 'NONE', *, *, #17175, .T. ) ;
#7345=ORIENTED_EDGE ( 'NONE', *, *, #362, .F. ) ;
#7346=DIRECTION ( 'NONE',  ( 0.000000000000000000, 0.000000000000000000, 1.000000000000000000 ) ) ;
#7347=ORIENTED_EDGE ( 'NONE', *, *, #5478, .F. ) ;
#7348=VERTEX_POINT ( 'NONE', #10653 ) ;
#7349=CARTESIAN_POINT ( 'NONE',  ( -57.85941822433785120, -87.13282127653275211, 21.65063509461101532 ) ) ;
#7350=EDGE_CURVE ( 'NONE', #16387, #10257, #16450, .T. ) ;
#7351=DIRECTION ( 'NONE',  ( -0.1566598588826321192, 0.9876526153536342445, 7.798540720466730171E-17 ) ) ;
#7352=ORIENTED_EDGE ( 'NONE', *, *, #7503, .T. ) ;
#7354=AXIS2_PLACEMENT_3D ( 'NONE', #1226, #7011, #11319 ) ;
#7355=CARTESIAN_POINT ( 'NONE',  ( -34.68921677370541090, -25.75213315644277046, 17.32050807568881723 ) ) ;
#7356=FACE_OUTER_BOUND ( 'NONE', #17740, .T. ) ;
#7357=DIRECTION ( 'NONE',  ( -0.9876526153536336894, -0.1566598588826350336, 0.000000000000000000 ) ) ;
#7358=EDGE_CURVE ( 'NONE', #15786, #2545, #7638, .T. ) ;
#7360=VERTEX_POINT ( 'NONE', #13576 ) ;
#7361=EDGE_CURVE ( 'NONE', #14719, #15217, #15481, .T. ) ;
#7362=ORIENTED_EDGE ( 'NONE', *, *, #17537, .T. ) ;
#7365=ORIENTED_EDGE ( 'NONE', *, *, #4087, .T. ) ;
#7366=ORIENTED_EDGE ( 'NONE', *, *, #4321, .F. ) ;
#7367=CARTESIAN_POINT ( 'NONE',  ( -15.92381708198642798, -22.77559583767277473, -21.65063509461098334 ) ) ;
#7368=CARTESIAN_POINT ( 'NONE',  ( -30.73860631229088725, -25.12549372091224598, 12.99038105676661736 ) ) ;
#7369=CARTESIAN_POINT ( 'NONE',  ( -62.13913668266656032, -25.04368626950569521, -8.660254037844380193 ) ) ;
#7370=CARTESIAN_POINT ( 'NONE',  ( 0.5768043922889515285, -15.09578523045857601, 17.32050807568881368 ) ) ;
#7371=AXIS2_PLACEMENT_3D ( 'NONE', #14779, #1804, #7591 ) ;
#7372=DIRECTION ( 'NONE',  ( -0.1566598588826321747, 0.9876526153536343555, 0.000000000000000000 ) ) ;
#7373=CARTESIAN_POINT ( 'NONE',  ( -56.21322099054479082, -24.10372711620990316, -4.330127018922180326 ) ) ;
#7374=ADVANCED_FACE ( 'NONE', ( #6123 ), #12235, .F. ) ;
#7375=CARTESIAN_POINT ( 'NONE',  ( -38.14600092744309734, -26.30044266253198160, -8.660254037844380193 ) ) ;
#7376=ORIENTED_EDGE ( 'NONE', *, *, #6633, .F. ) ;
#7377=CARTESIAN_POINT ( 'NONE',  ( -62.79768130110601021, -87.91612057094589261, -21.65063509461098690 ) ) ;
#7378=EDGE_CURVE ( 'NONE', #4161, #1436, #17706, .T. ) ;
#7379=EDGE_LOOP ( 'NONE', ( #879, #3050, #17474, #16226 ) ) ;
#7380=ADVANCED_FACE ( 'NONE', ( #625 ), #13303, .F. ) ;
#7381=CARTESIAN_POINT ( 'NONE',  ( -19.34096622554629263, -81.02308678011009135, -17.32050807568878525 ) ) ;
#7382=ORIENTED_EDGE ( 'NONE', *, *, #8530, .T. ) ;
#7383=ORIENTED_EDGE ( 'NONE', *, *, #15678, .T. ) ;
#7384=CIRCLE ( 'NONE', #8886, 1.499999999999999556 ) ;
#7385=DIRECTION ( 'NONE',  ( -0.1566598588826321192, 0.9876526153536342445, 7.798540720466730171E-17 ) ) ;
#7386=ADVANCED_FACE ( 'NONE', ( #5039 ), #10728, .T. ) ;
#7387=DIRECTION ( 'NONE',  ( -0.1566598588826321747, 0.9876526153536343555, 0.000000000000000000 ) ) ;
#7388=CARTESIAN_POINT ( 'NONE',  ( -14.44233815895597672, -22.54060604934882051, -21.65063509461098334 ) ) ;
#7389=ORIENTED_EDGE ( 'NONE', *, *, #13483, .F. ) ;
#7390=DIRECTION ( 'NONE',  ( -0.1566598588826321747, 0.9876526153536343555, 0.000000000000000000 ) ) ;
#7392=DIRECTION ( 'NONE',  ( -0.9876526153536341335, -0.1566598588826327021, 0.000000000000000000 ) ) ;
#7393=CARTESIAN_POINT ( 'NONE',  ( -35.63723437888119605, -83.60797445167352748, -17.32050807568878525 ) ) ;
#7394=EDGE_LOOP ( 'NONE', ( #13841, #2235, #5276, #10733 ) ) ;
#7397=DIRECTION ( 'NONE',  ( -0.1566598588826321192, 0.9876526153536342445, 7.798540720466730171E-17 ) ) ;
#7399=EDGE_LOOP ( 'NONE', ( #9180, #17108 ) ) ;
#7400=VERTEX_POINT ( 'NONE', #15101 ) ;
#7401=DIRECTION ( 'NONE',  ( -0.1566598588826321747, 0.9876526153536343555, 0.000000000000000000 ) ) ;
#7405=ORIENTED_EDGE ( 'NONE', *, *, #7189, .T. ) ;
#7406=DIRECTION ( 'NONE',  ( 0.000000000000000000, 0.000000000000000000, 1.000000000000000000 ) ) ;
#7407=DIRECTION ( 'NONE',  ( -0.1566598588826321192, 0.9876526153536342445, 7.798540720466730171E-17 ) ) ;
#7408=EDGE_CURVE ( 'NONE', #3070, #4072, #14272, .T. ) ;
#7409=DIRECTION ( 'NONE',  ( 0.000000000000000000, 0.000000000000000000, 1.000000000000000000 ) ) ;
#7411=CARTESIAN_POINT ( 'NONE',  ( 0.000000000000000000, 0.000000000000000000, -24.99999999999999289 ) ) ;
#7412=ORIENTED_EDGE ( 'NONE', *, *, #5511, .T. ) ;
#7413=EDGE_LOOP ( 'NONE', ( #1922, #4689 ) ) ;
#7414=FACE_OUTER_BOUND ( 'NONE', #7829, .T. ) ;
#7417=ORIENTED_EDGE ( 'NONE', *, *, #280, .F. ) ;
#7418=VERTEX_POINT ( 'NONE', #4771 ) ;
#7419=ORIENTED_EDGE ( 'NONE', *, *, #13193, .F. ) ;
#7420=CARTESIAN_POINT ( 'NONE',  ( 0.000000000000000000, 0.000000000000000000, 30.00000000000000000 ) ) ;
#7421=EDGE_CURVE ( 'NONE', #7348, #9121, #10631, .T. ) ;
#7424=LINE ( 'NONE', #7349, #18263 ) ;
#7425=EDGE_CURVE ( 'NONE', #3795, #12785, #4874, .T. ) ;
#7426=LINE ( 'NONE', #4569, #1206 ) ;
#7427=EDGE_LOOP ( 'NONE', ( #3337, #5795 ) ) ;
#7428=EDGE_CURVE ( 'NONE', #3494, #1209, #7330, .T. ) ;
#7429=VERTEX_POINT ( 'NONE', #3715 ) ;
#7430=ADVANCED_FACE ( 'NONE', ( #2505 ), #2398, .F. ) ;
#7431=ORIENTED_EDGE ( 'NONE', *, *, #18600, .T. ) ;
#7432=DIRECTION ( 'NONE',  ( -0.1566598588826321192, 0.9876526153536342445, 7.798540720466731404E-17 ) ) ;
#7433=VECTOR ( 'NONE', #16367, 1000.000000000000000 ) ;
#7434=DIRECTION ( 'NONE',  ( 0.000000000000000000, 0.000000000000000000, 1.000000000000000000 ) ) ;
#7436=ORIENTED_EDGE ( 'NONE', *, *, #17101, .F. ) ;
#7438=LINE ( 'NONE', #1932, #18476 ) ;
#7439=CARTESIAN_POINT ( 'NONE',  ( -39.91695283720987675, -21.51883944464649545, 21.65063509461101887 ) ) ;
#7440=FACE_OUTER_BOUND ( 'NONE', #16231, .T. ) ;
#7443=VERTEX_POINT ( 'NONE', #8083 ) ;
#7446=CIRCLE ( 'NONE', #11645, 1.500000000000000888 ) ;
#7447=EDGE_CURVE ( 'NONE', #11326, #7506, #8291, .T. ) ;
#7448=EDGE_CURVE ( 'NONE', #10670, #14934, #1098, .T. ) ;
#7450=DIRECTION ( 'NONE',  ( -0.1566598588826321747, 0.9876526153536343555, 0.000000000000000000 ) ) ;
#7452=AXIS2_PLACEMENT_3D ( 'NONE', #2429, #8114, #18210 ) ;
#7454=CARTESIAN_POINT ( 'NONE',  ( -1.892327146095121204, -15.48743487766515337, -4.330127018922183879 ) ) ;
#7457=EDGE_LOOP ( 'NONE', ( #5568, #9626, #11822, #4125 ) ) ;
#7458=ORIENTED_EDGE ( 'NONE', *, *, #14027, .T. ) ;
#7459=DIRECTION ( 'NONE',  ( -0.1566598588826321192, 0.9876526153536342445, 7.798540720466731404E-17 ) ) ;
#7461=DIRECTION ( 'NONE',  ( -0.9876526153536341335, -0.1566598588826327021, 0.000000000000000000 ) ) ;
#7463=DIRECTION ( 'NONE',  ( -0.9876526153536336894, -0.1566598588826349503, 0.000000000000000000 ) ) ;
#7464=ORIENTED_EDGE ( 'NONE', *, *, #3146, .T. ) ;
#7466=ADVANCED_FACE ( 'NONE', ( #8373 ), #8192, .F. ) ;
#7468=EDGE_CURVE ( 'NONE', #15912, #9201, #8825, .T. ) ;
#7470=CIRCLE ( 'NONE', #7176, 1.499999999999999556 ) ;
#7471=DIRECTION ( 'NONE',  ( 0.000000000000000000, 0.000000000000000000, 1.000000000000000000 ) ) ;
#7472=CARTESIAN_POINT ( 'NONE',  ( -64.31879523431432233, -30.45192892292171294, -17.32050807568878170 ) ) ;
#7473=DIRECTION ( 'NONE',  ( 0.000000000000000000, 0.000000000000000000, 1.000000000000000000 ) ) ;
#7474=EDGE_CURVE ( 'NONE', #4718, #16444, #16096, .T. ) ;
#7475=DIRECTION ( 'NONE',  ( -0.9876526153536344665, -0.1566598588826304539, 0.000000000000000000 ) ) ;
#7476=CYLINDRICAL_SURFACE ( 'NONE', #12881, 1.500000000000001554 ) ;
#7477=CIRCLE ( 'NONE', #15040, 1.500000000000001332 ) ;
#7478=CARTESIAN_POINT ( 'NONE',  ( -42.55080268635658314, -84.70459346385194976, 8.660254037844412167 ) ) ;
#7479=DIRECTION ( 'NONE',  ( -0.1566598588826321747, 0.9876526153536343555, 0.000000000000000000 ) ) ;
#7480=CIRCLE ( 'NONE', #18425, 1.500000000000000888 ) ;
#7481=CARTESIAN_POINT ( 'NONE',  ( -40.41077914488672462, -21.59716937408779103, -17.32050807568878170 ) ) ;
#7482=VERTEX_POINT ( 'NONE', #908 ) ;
#7483=ORIENTED_EDGE ( 'NONE', *, *, #4644, .F. ) ;
#7484=DIRECTION ( 'NONE',  ( -0.1566598588826321747, 0.9876526153536343555, 0.000000000000000000 ) ) ;
#7486=EDGE_LOOP ( 'NONE', ( #1512, #8049, #13929, #15175 ) ) ;
#7487=AXIS2_PLACEMENT_3D ( 'NONE', #4715, #16289, #9086 ) ;
#7488=ORIENTED_EDGE ( 'NONE', *, *, #8761, .F. ) ;
#7489=EDGE_LOOP ( 'NONE', ( #10648, #13832 ) ) ;
#7491=DIRECTION ( 'NONE',  ( -0.1566598588826321192, 0.9876526153536342445, 7.798540720466730171E-17 ) ) ;
#7492=AXIS2_PLACEMENT_3D ( 'NONE', #6013, #7531, #11763 ) ;
#7493=FACE_OUTER_BOUND ( 'NONE', #2255, .T. ) ;
#7495=EDGE_CURVE ( 'NONE', #6575, #15928, #1011, .T. ) ;
#7498=AXIS2_PLACEMENT_3D ( 'NONE', #10455, #8945, #14823 ) ;
#7499=CARTESIAN_POINT ( 'NONE',  ( -1.109027851681966492, -20.42569795443330349, -4.330127018922184767 ) ) ;
#7500=APPLICATION_CONTEXT ( 'automotive_design' ) ;
#7502=CARTESIAN_POINT ( 'NONE',  ( -42.09661138885762455, -26.92708209806250608, -4.330127018922181215 ) ) ;
#7503=EDGE_CURVE ( 'NONE', #9998, #11443, #13003, .T. ) ;
#7504=DIRECTION ( 'NONE',  ( -0.1566598588826321192, 0.9876526153536342445, 7.798540720466731404E-17 ) ) ;
#7505=VERTEX_POINT ( 'NONE', #15946 ) ;
#7506=VERTEX_POINT ( 'NONE', #2682 ) ;
#7507=ORIENTED_EDGE ( 'NONE', *, *, #6388, .F. ) ;
#7508=FACE_OUTER_BOUND ( 'NONE', #8338, .T. ) ;
#7509=EDGE_LOOP ( 'NONE', ( #15898, #13828, #16248, #12132 ) ) ;
#7510=FACE_BOUND ( 'NONE', #14641, .T. ) ;
#7512=DIRECTION ( 'NONE',  ( -0.1566598588826321192, 0.9876526153536342445, 7.798540720466730171E-17 ) ) ;
#7514=FACE_OUTER_BOUND ( 'NONE', #18660, .T. ) ;
#7515=ORIENTED_EDGE ( 'NONE', *, *, #8033, .T. ) ;
#7517=DIRECTION ( 'NONE',  ( -0.9876526153536341335, -0.1566598588826327021, 0.000000000000000000 ) ) ;
#7518=EDGE_CURVE ( 'NONE', #1621, #18301, #7248, .T. ) ;
#7519=CIRCLE ( 'NONE', #5719, 1.500000000000000444 ) ;
#7521=DIRECTION ( 'NONE',  ( -0.1566598588826321192, 0.9876526153536342445, 7.798540720466730171E-17 ) ) ;
#7522=CIRCLE ( 'NONE', #5723, 1.500000000000001332 ) ;
#7525=EDGE_CURVE ( 'NONE', #9571, #14620, #7343, .T. ) ;
#7526=CARTESIAN_POINT ( 'NONE',  ( -0.4108482230646692823, -15.25244508934120802, -12.99038105676658361 ) ) ;
#7527=CARTESIAN_POINT ( 'NONE',  ( -53.90880776292333820, -86.50618184100221697, 8.660254037844412167 ) ) ;
#7528=ORIENTED_EDGE ( 'NONE', *, *, #9376, .T. ) ;
#7529=ORIENTED_EDGE ( 'NONE', *, *, #8585, .T. ) ;
#7530=DIRECTION ( 'NONE',  ( -0.1566598588826321747, 0.9876526153536343555, 0.000000000000000000 ) ) ;
#7531=DIRECTION ( 'NONE',  ( -0.1566598588826321192, 0.9876526153536342445, 7.798540720466731404E-17 ) ) ;
#7532=CARTESIAN_POINT ( 'NONE',  ( -58.84707083969148300, -87.28948113541537168, -8.660254037844385522 ) ) ;
#7534=AXIS2_PLACEMENT_3D ( 'NONE', #10334, #17763, #17678 ) ;
#7535=ORIENTED_EDGE ( 'NONE', *, *, #12086, .F. ) ;
#7536=CARTESIAN_POINT ( 'NONE',  ( -67.73594437787414790, -88.69941986535906153, 21.65063509461101532 ) ) ;
#7537=CIRCLE ( 'NONE', #17250, 1.500000000000001332 ) ;
#7541=DIRECTION ( 'NONE',  ( 0.000000000000000000, 0.000000000000000000, 1.000000000000000000 ) ) ;
#7547=AXIS2_PLACEMENT_3D ( 'NONE', #10243, #7783, #3048 ) ;
#7548=CARTESIAN_POINT ( 'NONE',  ( -34.15575545585074480, -83.37298466334958391, -8.660254037844385522 ) ) ;
#7549=DIRECTION ( 'NONE',  ( -0.1566598588826321192, 0.9876526153536342445, 7.798540720466730171E-17 ) ) ;
#7551=DIRECTION ( 'NONE',  ( -0.1566598588826321747, 0.9876526153536343555, 0.000000000000000000 ) ) ;
#7552=ORIENTED_EDGE ( 'NONE', *, *, #8475, .F. ) ;
#7553=VERTEX_POINT ( 'NONE', #1563 ) ;
#7554=DIRECTION ( 'NONE',  ( -0.9876526153536341335, -0.1566598588826327021, 0.000000000000000000 ) ) ;
#7555=VECTOR ( 'NONE', #9728, 1000.000000000000000 ) ;
#7556=AXIS2_PLACEMENT_3D ( 'NONE', #10219, #16008, #4536 ) ;
#7557=AXIS2_PLACEMENT_3D ( 'NONE', #16454, #7821, #16535 ) ;
#7558=ORIENTED_EDGE ( 'NONE', *, *, #14992, .T. ) ;
#7559=EDGE_LOOP ( 'NONE', ( #10766, #14568, #1919, #8390 ) ) ;
#7561=CIRCLE ( 'NONE', #6370, 1.500000000000000888 ) ;
#7563=CIRCLE ( 'NONE', #6667, 1.500000000000000444 ) ;
#7565=AXIS2_PLACEMENT_3D ( 'NONE', #221, #5912, #17405 ) ;
#7566=CARTESIAN_POINT ( 'NONE',  ( 0.000000000000000000, 0.000000000000000000, -24.99999999999999289 ) ) ;
#7567=CARTESIAN_POINT ( 'NONE',  ( 0.4120860815263194254, -77.88988960245745830, 1.077796531449093893E-14 ) ) ;
#7568=AXIS2_PLACEMENT_3D ( 'NONE', #6342, #12074, #9906 ) ;
#7570=DIRECTION ( 'NONE',  ( 0.000000000000000000, 0.000000000000000000, 1.000000000000000000 ) ) ;
#7571=LINE ( 'NONE', #16193, #18161 ) ;
#7573=CIRCLE ( 'NONE', #14242, 1.499999999999999556 ) ;
#7574=CARTESIAN_POINT ( 'NONE',  ( -35.67686938905902849, -25.90879301532540779, 12.99038105676661736 ) ) ;
#7575=ORIENTED_EDGE ( 'NONE', *, *, #8063, .F. ) ;
#7578=ORIENTED_EDGE ( 'NONE', *, *, #5855, .F. ) ;
#7579=ADVANCED_FACE ( 'NONE', ( #2862 ), #5731, .F. ) ;
#7580=EDGE_LOOP ( 'NONE', ( #8468, #5016 ) ) ;
#7581=AXIS2_PLACEMENT_3D ( 'NONE', #3232, #6109, #6399 ) ;
#7582=ORIENTED_EDGE ( 'NONE', *, *, #7428, .F. ) ;
#7584=CARTESIAN_POINT ( 'NONE',  ( -39.09401853261887538, -84.15628395776273862, 17.32050807568881368 ) ) ;
#7585=CIRCLE ( 'NONE', #13624, 1.500000000000000444 ) ;
#7586=ORIENTED_EDGE ( 'NONE', *, *, #8928, .T. ) ;
#7587=EDGE_LOOP ( 'NONE', ( #2758, #6560 ) ) ;
#7588=CARTESIAN_POINT ( 'NONE',  ( -7.528769851480577202, -21.44398703717040888, -4.330127018922184767 ) ) ;
#7589=CARTESIAN_POINT ( 'NONE',  ( -61.31620237807555895, -87.68113078262196325, 12.99038105676661203 ) ) ;
#7590=AXIS2_PLACEMENT_3D ( 'NONE', #12155, #13860, #3717 ) ;
#7591=DIRECTION ( 'NONE',  ( -0.9876526153536336894, -0.1566598588826349503, 0.000000000000000000 ) ) ;
#7592=AXIS2_PLACEMENT_3D ( 'NONE', #5671, #11420, #17253 ) ;
#7593=ORIENTED_EDGE ( 'NONE', *, *, #13938, .T. ) ;
#7594=CARTESIAN_POINT ( 'NONE',  ( -46.50141314777111745, -85.33123289938248490, -4.330127018922185655 ) ) ;
#7595=CIRCLE ( 'NONE', #18232, 1.500000000000001332 ) ;
#7596=LINE ( 'NONE', #9103, #7819 ) ;
#7597=DIRECTION ( 'NONE',  ( -0.1566598588826321192, 0.9876526153536342445, 7.798540720466730171E-17 ) ) ;
#7598=DIRECTION ( 'NONE',  ( 0.000000000000000000, 0.000000000000000000, 1.000000000000000000 ) ) ;
#7599=ORIENTED_EDGE ( 'NONE', *, *, #12705, .T. ) ;
#7600=FACE_BOUND ( 'NONE', #5472, .T. ) ;
#7603=CARTESIAN_POINT ( 'NONE',  ( -3.538524379888208227, -78.51652903798800764, 4.330127018922209636 ) ) ;
#7605=CARTESIAN_POINT ( 'NONE',  ( -56.21322099054477661, -24.10372711620991026, 12.99038105676661736 ) ) ;
#7606=ORIENTED_EDGE ( 'NONE', *, *, #14706, .F. ) ;
#7607=VECTOR ( 'NONE', #6600, 1000.000000000000000 ) ;
#7608=VERTEX_POINT ( 'NONE', #1289 ) ;
#7609=ORIENTED_EDGE ( 'NONE', *, *, #14943, .F. ) ;
#7610=VERTEX_POINT ( 'NONE', #11574 ) ;
#7612=AXIS2_PLACEMENT_3D ( 'NONE', #5435, #6581, #15484 ) ;
#7613=EDGE_CURVE ( 'NONE', #859, #14096, #7424, .T. ) ;
#7614=FACE_BOUND ( 'NONE', #3688, .T. ) ;
#7615=EDGE_LOOP ( 'NONE', ( #5587, #12165, #14385, #2233 ) ) ;
#7616=CARTESIAN_POINT ( 'NONE',  ( -2.879979761448749009, -15.64409473654778893, 17.32050807568881012 ) ) ;
#7617=ORIENTED_EDGE ( 'NONE', *, *, #9056, .F. ) ;
#7618=ADVANCED_FACE ( 'NONE', ( #4084, #17481, #5831, #14257, #4384, #17312, #1374, #18663, #4471, #10251, #5631, #17209, #13181, #15771, #14535, #209, #2789, #8576, #14347, #4296, #10069, #7157, #15856, #4842, #11846, #6390, #4655, #3221, #9017, #6479, #498, #1724, #9122, #6195, #14989, #10709, #9296, #13650, #16430, #597, #17864, #11924, #16227, #3411, #16510, #13272, #3498, #13549, #3321, #10630, #12124, #1918, #13377, #15076, #2099, #7886, #9214, #2004, #17683, #7793, #694, #14708, #410, #17771, #17586, #17964, #10529, #4928, #4748, #4568, #7704, #16324, #10342, #7614, #1823, #14897, #16143, #3136, #8927, #7510, #308, #10434, #6100, #13456, #14800, #6292, #12020, #782, #5416, #12310, #2483, #3778, #9494, #989, #11175, #18054, #12511, #14032, #17003, #9581, #16715, #3870, #1171, #9696, #16812, #12214, #8167, #2278, #8272, #5233, #5323, #6760, #15358, #6565, #18352, #1079, #8061, #3594, #2374, #16608, #7975, #6663, #5015, #13837, #15261, #884, #3977, #10793, #6848, #2566, #15549, #9402, #13936, #15465, #11080, #16905, #15180, #5124, #14122, #8352, #12418, #12593, #18262, #18452, #10983, #9779, #18154, #2194, #13732, #10896, #3691, #1441, #11277, #9864, #15840, #7052, #11549, #6952, #4065, #4272, #17289, #8452, #11633, #7136, #12977, #17459, #14330, #5610, #17380, #5888, #2659, #4448, #2928, #11453, #17, #1536, #10050, #2768, #105, #10228, #16021, #5809 ), #14603, .F. ) ;
#7619=CIRCLE ( 'NONE', #2474, 1.500000000000000888 ) ;
#7620=CIRCLE ( 'NONE', #7911, 2.500000000000002220 ) ;
#7623=FACE_BOUND ( 'NONE', #4354, .T. ) ;
#7624=AXIS2_PLACEMENT_3D ( 'NONE', #4047, #18338, #3955 ) ;
#7625=FACE_OUTER_BOUND ( 'NONE', #13684, .T. ) ;
#7627=CIRCLE ( 'NONE', #7935, 2.500000000000002220 ) ;
#7630=ORIENTED_EDGE ( 'NONE', *, *, #3962, .T. ) ;
#7631=ORIENTED_EDGE ( 'NONE', *, *, #17607, .T. ) ;
#7632=CARTESIAN_POINT ( 'NONE',  ( -60.16383145195931803, -24.73036655174042409, -17.32050807568878170 ) ) ;
#7633=CARTESIAN_POINT ( 'NONE',  ( -52.92115514756970640, -86.34952198211959740, 12.99038105676661203 ) ) ;
#7634=CIRCLE ( 'NONE', #7923, 1.499999999999999556 ) ;
#7635=EDGE_CURVE ( 'NONE', #7782, #4359, #2783, .T. ) ;
#7636=VERTEX_POINT ( 'NONE', #15924 ) ;
#7637=EDGE_LOOP ( 'NONE', ( #7115, #13195, #1185, #7799 ) ) ;
#7638=LINE ( 'NONE', #1749, #3648 ) ;
#7639=CARTESIAN_POINT ( 'NONE',  ( 6.831828081324923474, -76.87160051972034580, 1.096166233436304165E-14 ) ) ;
#7640=AXIS2_PLACEMENT_3D ( 'NONE', #550, #1874, #4972 ) ;
#7641=FACE_BOUND ( 'NONE', #1769, .T. ) ;
#7642=EDGE_CURVE ( 'NONE', #1565, #10521, #10036, .T. ) ;
#7643=DIRECTION ( 'NONE',  ( 0.000000000000000000, 0.000000000000000000, 1.000000000000000000 ) ) ;
#7644=CARTESIAN_POINT ( 'NONE',  ( -2.000000000000000000, 0.000000000000000000, -24.99999999999999289 ) ) ;
#7645=LINE ( 'NONE', #10559, #281 ) ;
#7647=EDGE_LOOP ( 'NONE', ( #17634, #18658 ) ) ;
#7648=VECTOR ( 'NONE', #16804, 1000.000000000000000 ) ;
#7652=EDGE_LOOP ( 'NONE', ( #10797, #14956 ) ) ;
#7653=ORIENTED_EDGE ( 'NONE', *, *, #3850, .F. ) ;
#7655=CARTESIAN_POINT ( 'NONE',  ( 7.819480696678544618, -76.71494066083772623, -21.65063509461098690 ) ) ;
#7656=AXIS2_PLACEMENT_3D ( 'NONE', #17309, #8573, #7346 ) ;
#7658=VERTEX_POINT ( 'NONE', #8554 ) ;
#7659=EDGE_CURVE ( 'NONE', #14531, #17742, #14287, .T. ) ;
#7660=ORIENTED_EDGE ( 'NONE', *, *, #5090, .T. ) ;
#7661=ADVANCED_FACE ( 'NONE', ( #5521 ), #11364, .F. ) ;
#7662=EDGE_CURVE ( 'NONE', #18009, #2581, #4594, .T. ) ;
#7663=LINE ( 'NONE', #10576, #15953 ) ;
#7664=EDGE_CURVE ( 'NONE', #16734, #17282, #7627, .T. ) ;
#7665=AXIS2_PLACEMENT_3D ( 'NONE', #16413, #9195, #14965 ) ;
#7667=DIRECTION ( 'NONE',  ( -0.9876526153536336894, -0.1566598588826350336, 0.000000000000000000 ) ) ;
#7668=ORIENTED_EDGE ( 'NONE', *, *, #16412, .T. ) ;
#7672=ORIENTED_EDGE ( 'NONE', *, *, #13982, .F. ) ;
#7673=DIRECTION ( 'NONE',  ( -0.1566598588826321192, 0.9876526153536342445, 7.798540720466730171E-17 ) ) ;
#7674=DIRECTION ( 'NONE',  ( -0.1566598588826321192, 0.9876526153536342445, 7.798540720466730171E-17 ) ) ;
#7675=DIRECTION ( 'NONE',  ( 0.000000000000000000, 0.000000000000000000, 1.000000000000000000 ) ) ;
#7676=CYLINDRICAL_SURFACE ( 'NONE', #10259, 1.500000000000001554 ) ;
#7677=EDGE_LOOP ( 'NONE', ( #5582, #15521 ) ) ;
#7678=DIRECTION ( 'NONE',  ( -0.9876526153536341335, -0.1566598588826327021, 0.000000000000000000 ) ) ;
#7679=ORIENTED_EDGE ( 'NONE', *, *, #11619, .F. ) ;
#7681=CYLINDRICAL_SURFACE ( 'NONE', #15028, 1.500000000000001554 ) ;
#7682=EDGE_CURVE ( 'NONE', #9201, #16508, #14414, .T. ) ;
#7683=DIRECTION ( 'NONE',  ( -0.1566598588826321747, 0.9876526153536343555, 0.000000000000000000 ) ) ;
#7684=VERTEX_POINT ( 'NONE', #10503 ) ;
#7685=CARTESIAN_POINT ( 'NONE',  ( -16.91146969734005268, -22.93225569655540141, 8.660254037844417496 ) ) ;
#7686=LINE ( 'NONE', #6607, #4699 ) ;
#7687=CARTESIAN_POINT ( 'NONE',  ( 2.447859171744379392, -14.79900155049412014, -24.99999999999999289 ) ) ;
#7688=EDGE_CURVE ( 'NONE', #15443, #2695, #10644, .T. ) ;
#7689=EDGE_CURVE ( 'NONE', #3263, #4160, #1625, .T. ) ;
#7691=CARTESIAN_POINT ( 'NONE',  ( 2.000000000000000000, 2.449293598294706414E-16, 30.00000000000000000 ) ) ;
#7693=CARTESIAN_POINT ( 'NONE',  ( -1.892327146095128310, -15.48743487766515337, -21.65063509461097979 ) ) ;
#7694=ORIENTED_EDGE ( 'NONE', *, *, #1068, .T. ) ;
#7695=ORIENTED_EDGE ( 'NONE', *, *, #1576, .F. ) ;
#7696=DIRECTION ( 'NONE',  ( -0.1566598588826321192, 0.9876526153536342445, 7.798540720466730171E-17 ) ) ;
#7697=CARTESIAN_POINT ( 'NONE',  ( -31.52190560670403841, -20.18723064414412249, 21.65063509461102242 ) ) ;
#7698=ORIENTED_EDGE ( 'NONE', *, *, #2195, .T. ) ;
#7700=ORIENTED_EDGE ( 'NONE', *, *, #10985, .T. ) ;
#7701=DIRECTION ( 'NONE',  ( 0.000000000000000000, 0.000000000000000000, 1.000000000000000000 ) ) ;
#7702=VERTEX_POINT ( 'NONE', #9192 ) ;
#7704=FACE_BOUND ( 'NONE', #15528, .T. ) ;
#7705=VERTEX_POINT ( 'NONE', #13355 ) ;
#7706=ORIENTED_EDGE ( 'NONE', *, *, #11389, .T. ) ;
#7708=EDGE_CURVE ( 'NONE', #7294, #10326, #13433, .T. ) ;
#7709=EDGE_LOOP ( 'NONE', ( #3086, #12853, #17911, #1032 ) ) ;
#7710=CARTESIAN_POINT ( 'NONE',  ( -38.14600092744310444, -26.30044266253198160, 17.32050807568881723 ) ) ;
#7712=LINE ( 'NONE', #13658, #17297 ) ;
#7713=CARTESIAN_POINT ( 'NONE',  ( -50.49165861936346289, -28.25869089856487903, 12.99038105676661736 ) ) ;
#7714=DIRECTION ( 'NONE',  ( -0.9876526153536341335, -0.1566598588826327021, 0.000000000000000000 ) ) ;
#7716=ORIENTED_EDGE ( 'NONE', *, *, #239, .F. ) ;
#7717=ORIENTED_EDGE ( 'NONE', *, *, #8633, .F. ) ;
#7718=CARTESIAN_POINT ( 'NONE',  ( -19.34096622554629263, -81.02308678011010556, -8.660254037844385522 ) ) ;
#7719=VECTOR ( 'NONE', #7696, 1000.000000000000000 ) ;
#7720=CYLINDRICAL_SURFACE ( 'NONE', #10869, 1.500000000000001554 ) ;
#7721=CARTESIAN_POINT ( 'NONE',  ( -10.78120068427780964, -16.89737360760884144, 1.561251128379126385E-14 ) ) ;
#7722=ORIENTED_EDGE ( 'NONE', *, *, #10438, .T. ) ;
#7723=VERTEX_POINT ( 'NONE', #4638 ) ;
#7724=LINE ( 'NONE', #13475, #10317 ) ;
#7725=ORIENTED_EDGE ( 'NONE', *, *, #17460, .F. ) ;
#7726=DIRECTION ( 'NONE',  ( 2.887450008416415878E-16, 0.000000000000000000, 1.000000000000000000 ) ) ;
#7730=CARTESIAN_POINT ( 'NONE',  ( -24.11451099155181055, -19.01228170252437266, -17.32050807568878170 ) ) ;
#7732=LINE ( 'NONE', #7924, #2869 ) ;
#7733=ORIENTED_EDGE ( 'NONE', *, *, #11578, .T. ) ;
#7734=ORIENTED_EDGE ( 'NONE', *, *, #12221, .F. ) ;
#7735=LINE ( 'NONE', #10381, #15464 ) ;
#7737=EDGE_CURVE ( 'NONE', #17224, #5271, #1585, .T. ) ;
#7738=CARTESIAN_POINT ( 'NONE',  ( -55.22556837519115902, -23.94706725732727648, 8.660254037844417496 ) ) ;
#7739=AXIS2_PLACEMENT_3D ( 'NONE', #138, #13013, #18761 ) ;
#7740=ADVANCED_FACE ( 'NONE', ( #11904 ), #473, .F. ) ;
#7741=EDGE_LOOP ( 'NONE', ( #9915, #17483 ) ) ;
#7742=DIRECTION ( 'NONE',  ( 0.000000000000000000, 0.000000000000000000, 1.000000000000000000 ) ) ;
#7743=FACE_OUTER_BOUND ( 'NONE', #13449, .T. ) ;
#7745=LINE ( 'NONE', #11971, #18269 ) ;
#7746=LINE ( 'NONE', #16191, #17240 ) ;
#7748=AXIS2_PLACEMENT_3D ( 'NONE', #14021, #2265, #9570 ) ;
#7751=DIRECTION ( 'NONE',  ( -0.1566598588826321192, 0.9876526153536342445, 7.798540720466730171E-17 ) ) ;
#7753=ADVANCED_FACE ( 'NONE', ( #17745 ), #3386, .F. ) ;
#7754=CARTESIAN_POINT ( 'NONE',  ( -28.06512145296634486, -19.63892113805490425, 4.330127018922218518 ) ) ;
#7755=ORIENTED_EDGE ( 'NONE', *, *, #18331, .T. ) ;
#7756=EDGE_CURVE ( 'NONE', #18320, #11583, #12770, .T. ) ;
#7757=CARTESIAN_POINT ( 'NONE',  ( -57.69469991357523497, -24.33871690453385739, 12.99038105676661736 ) ) ;
#7758=CIRCLE ( 'NONE', #18402, 1.500000000000001332 ) ;
#7759=VERTEX_POINT ( 'NONE', #7764 ) ;
#7760=ORIENTED_EDGE ( 'NONE', *, *, #1940, .F. ) ;
#7761=EDGE_LOOP ( 'NONE', ( #9860, #15009, #13900, #7224 ) ) ;
#7762=DIRECTION ( 'NONE',  ( -0.9876526153536336894, -0.1566598588826349503, 0.000000000000000000 ) ) ;
#7763=CIRCLE ( 'NONE', #16867, 1.499999999999999556 ) ;
#7764=CARTESIAN_POINT ( 'NONE',  ( -74.48479437458692587, -27.00193450553858554, -21.65063509461098334 ) ) ;
#7765=EDGE_LOOP ( 'NONE', ( #18473, #5462 ) ) ;
#7766=LINE ( 'NONE', #6367, #1029 ) ;
#7767=DIRECTION ( 'NONE',  ( -0.1566598588826321192, 0.9876526153536342445, 7.798540720466730171E-17 ) ) ;
#7768=DIRECTION ( 'NONE',  ( -0.9876526153536336894, -0.1566598588826349503, 0.000000000000000000 ) ) ;
#7772=CARTESIAN_POINT ( 'NONE',  ( -54.89646037827696290, -86.66284169988483654, -21.65063509461098690 ) ) ;
#7773=DIRECTION ( 'NONE',  ( 0.000000000000000000, 0.000000000000000000, 1.000000000000000000 ) ) ;
#7774=DIRECTION ( 'NONE',  ( -0.1566598588826321192, 0.9876526153536342445, 7.798540720466730171E-17 ) ) ;
#7775=ORIENTED_EDGE ( 'NONE', *, *, #15544, .T. ) ;
#7776=FACE_BOUND ( 'NONE', #8617, .T. ) ;
#7777=EDGE_CURVE ( 'NONE', #11377, #1673, #4818, .T. ) ;
#7779=ORIENTED_EDGE ( 'NONE', *, *, #15572, .T. ) ;
#7780=DIRECTION ( 'NONE',  ( -0.9876526153536336894, -0.1566598588826349503, 0.000000000000000000 ) ) ;
#7781=CIRCLE ( 'NONE', #10184, 1.500000000000000888 ) ;
#7782=VERTEX_POINT ( 'NONE', #187 ) ;
#7783=DIRECTION ( 'NONE',  ( -0.1566598588826321747, 0.9876526153536343555, 0.000000000000000000 ) ) ;
#7785=ORIENTED_EDGE ( 'NONE', *, *, #16522, .T. ) ;
#7786=ORIENTED_EDGE ( 'NONE', *, *, #15864, .F. ) ;
#7787=LINE ( 'NONE', #5157, #1116 ) ;
#7788=ORIENTED_EDGE ( 'NONE', *, *, #10748, .T. ) ;
#7789=VERTEX_POINT ( 'NONE', #10694 ) ;
#7790=DIRECTION ( 'NONE',  ( 0.000000000000000000, 0.000000000000000000, 1.000000000000000000 ) ) ;
#7791=AXIS2_PLACEMENT_3D ( 'NONE', #14090, #16870, #12852 ) ;
#7792=EDGE_LOOP ( 'NONE', ( #8504, #9735, #7938, #6146 ) ) ;
#7793=FACE_BOUND ( 'NONE', #18424, .T. ) ;
#7794=CARTESIAN_POINT ( 'NONE',  ( -14.23798483801550674, -17.44568311369805969, 1.908195823574487804E-14 ) ) ;
#7795=ORIENTED_EDGE ( 'NONE', *, *, #14134, .F. ) ;
#7796=CIRCLE ( 'NONE', #1745, 1.500000000000000000 ) ;
#7797=VERTEX_POINT ( 'NONE', #570 ) ;
#7798=FACE_BOUND ( 'NONE', #8065, .T. ) ;
#7799=ORIENTED_EDGE ( 'NONE', *, *, #13175, .T. ) ;
#7801=DIRECTION ( 'NONE',  ( -0.9876526153536341335, -0.1566598588826327021, 0.000000000000000000 ) ) ;
#7803=CARTESIAN_POINT ( 'NONE',  ( -2.879979761448749009, -15.64409473654778893, -8.660254037844383745 ) ) ;
#7804=CARTESIAN_POINT ( 'NONE',  ( -15.71946376104596155, -17.68067290202200326, -8.660254037844380193 ) ) ;
#7805=ORIENTED_EDGE ( 'NONE', *, *, #5158, .F. ) ;
#7806=VERTEX_POINT ( 'NONE', #12099 ) ;
#7807=DIRECTION ( 'NONE',  ( -0.1566598588826321192, 0.9876526153536342445, 7.798540720466730171E-17 ) ) ;
#7809=DIRECTION ( 'NONE',  ( -0.1566598588826321192, 0.9876526153536342445, 7.798540720466730171E-17 ) ) ;
#7810=ADVANCED_FACE ( 'NONE', ( #6075 ), #4910, .F. ) ;
#7811=CARTESIAN_POINT ( 'NONE',  ( 7.819480696678551723, -76.71494066083772623, 12.99038105676660493 ) ) ;
#7812=ADVANCED_FACE ( 'NONE', ( #14686 ), #13161, .F. ) ;
#7813=VERTEX_POINT ( 'NONE', #10870 ) ;
#7814=LINE ( 'NONE', #12046, #14574 ) ;
#7815=EDGE_LOOP ( 'NONE', ( #6142, #9440 ) ) ;
#7817=AXIS2_PLACEMENT_3D ( 'NONE', #6064, #6161, #3186 ) ;
#7818=CARTESIAN_POINT ( 'NONE',  ( -61.31620237807555895, -87.68113078262193483, -21.65063509461098690 ) ) ;
#7819=VECTOR ( 'NONE', #6082, 1000.000000000000000 ) ;
#7820=AXIS2_PLACEMENT_3D ( 'NONE', #13769, #3533, #16197 ) ;
#7821=DIRECTION ( 'NONE',  ( -0.1566598588826321192, 0.9876526153536342445, 7.798540720466731404E-17 ) ) ;
#7824=CARTESIAN_POINT ( 'NONE',  ( -47.81817376003892406, -22.77211831570754441, 21.65063509461101887 ) ) ;
#7825=DIRECTION ( 'NONE',  ( 0.000000000000000000, 0.000000000000000000, 1.000000000000000000 ) ) ;
#7826=DIRECTION ( 'NONE',  ( -0.1566598588826321747, 0.9876526153536343555, 0.000000000000000000 ) ) ;
#7828=CARTESIAN_POINT ( 'NONE',  ( -80.30645961545690170, -27.92535762103353392, -24.99999999999999645 ) ) ;
#7829=EDGE_LOOP ( 'NONE', ( #13753, #6310, #443, #14629 ) ) ;
#7830=ORIENTED_EDGE ( 'NONE', *, *, #5814, .T. ) ;
#7831=CARTESIAN_POINT ( 'NONE',  ( -15.22563745336913144, -17.60234297258069347, -4.330127018922180326 ) ) ;
#7832=ORIENTED_EDGE ( 'NONE', *, *, #4294, .T. ) ;
#7837=DIRECTION ( 'NONE',  ( -0.9876526153536341335, -0.1566598588826327021, 0.000000000000000000 ) ) ;
#7838=DIRECTION ( 'NONE',  ( 0.000000000000000000, 0.000000000000000000, 1.000000000000000000 ) ) ;
#7839=CIRCLE ( 'NONE', #2683, 1.500000000000001332 ) ;
#7840=EDGE_LOOP ( 'NONE', ( #11882, #525 ) ) ;
#7842=AXIS2_PLACEMENT_3D ( 'NONE', #8568, #9792, #2855 ) ;
#7843=EDGE_LOOP ( 'NONE', ( #7775, #10043 ) ) ;
#7845=EDGE_CURVE ( 'NONE', #299, #15709, #14014, .T. ) ;
#7846=AXIS2_PLACEMENT_3D ( 'NONE', #2245, #10588, #16389 ) ;
#7847=CARTESIAN_POINT ( 'NONE',  ( -46.33669483700850122, -22.53712852738357952, -21.65063509461097979 ) ) ;
#7850=CARTESIAN_POINT ( 'NONE',  ( -36.62488699423479943, -83.76463431055617548, 12.99038105676661203 ) ) ;
#7851=CARTESIAN_POINT ( 'NONE',  ( -43.86756329862441817, -22.14547888017700217, -17.32050807568878170 ) ) ;
#7852=ORIENTED_EDGE ( 'NONE', *, *, #11572, .F. ) ;
#7853=CARTESIAN_POINT ( 'NONE',  ( -75.18297400320422241, -32.17518737063066681, -21.65063509461098334 ) ) ;
#7854=EDGE_LOOP ( 'NONE', ( #1658, #9486, #17910, #1049 ) ) ;
#7855=VECTOR ( 'NONE', #17401, 1000.000000000000000 ) ;
#7856=DIRECTION ( 'NONE',  ( -0.9876526153536336894, -0.1566598588826350336, 0.000000000000000000 ) ) ;
#7857=AXIS2_PLACEMENT_3D ( 'NONE', #1716, #7504, #1074 ) ;
#7858=EDGE_LOOP ( 'NONE', ( #8234, #11548, #5747, #16182 ) ) ;
#7859=VERTEX_POINT ( 'NONE', #2459 ) ;
#7860=CIRCLE ( 'NONE', #12060, 1.500000000000000000 ) ;
#7861=EDGE_CURVE ( 'NONE', #1673, #14356, #8555, .T. ) ;
#7862=AXIS2_PLACEMENT_3D ( 'NONE', #14025, #9573, #9773 ) ;
#7865=DIRECTION ( 'NONE',  ( -0.9876526153536341335, -0.1566598588826327021, 0.000000000000000000 ) ) ;
#7866=FACE_OUTER_BOUND ( 'NONE', #7637, .T. ) ;
#7869=VECTOR ( 'NONE', #12168, 1000.000000000000000 ) ;
#7870=LINE ( 'NONE', #3678, #8726 ) ;
#7872=CARTESIAN_POINT ( 'NONE',  ( -39.09401853261890381, -84.15628395776272441, -17.32050807568878525 ) ) ;
#7873=ORIENTED_EDGE ( 'NONE', *, *, #13364, .T. ) ;
#7874=FACE_BOUND ( 'NONE', #7286, .T. ) ;
#7875=VECTOR ( 'NONE', #5640, 1000.000000000000000 ) ;
#7878=CARTESIAN_POINT ( 'NONE',  ( -61.31620237807555895, -87.68113078262196325, 12.99038105676661203 ) ) ;
#7880=VERTEX_POINT ( 'NONE', #9372 ) ;
#7882=VECTOR ( 'NONE', #5493, 1000.000000000000000 ) ;
#7883=ORIENTED_EDGE ( 'NONE', *, *, #9495, .F. ) ;
#7884=ORIENTED_EDGE ( 'NONE', *, *, #101, .F. ) ;
#7885=CARTESIAN_POINT ( 'NONE',  ( -24.81269062016910709, -24.18553456761645393, -17.32050807568878170 ) ) ;
#7886=FACE_BOUND ( 'NONE', #1416, .T. ) ;
#7887=EDGE_CURVE ( 'NONE', #17944, #6916, #17329, .T. ) ;
#7888=AXIS2_PLACEMENT_3D ( 'NONE', #10143, #15931, #14521 ) ;
#7889=EDGE_CURVE ( 'NONE', #12097, #3494, #18032, .T. ) ;
#7892=CIRCLE ( 'NONE', #5476, 1.499999999999999556 ) ;
#7893=CIRCLE ( 'NONE', #10302, 1.500000000000001332 ) ;
#7894=DIRECTION ( 'NONE',  ( 0.000000000000000000, 0.000000000000000000, 1.000000000000000000 ) ) ;
#7895=CIRCLE ( 'NONE', #3940, 1.500000000000000000 ) ;
#7896=DIRECTION ( 'NONE',  ( -0.1566598588826321192, 0.9876526153536342445, 7.798540720466730171E-17 ) ) ;
#7897=DIRECTION ( 'NONE',  ( -0.1566598588826321747, 0.9876526153536343555, 0.000000000000000000 ) ) ;
#7902=VERTEX_POINT ( 'NONE', #858 ) ;
#7903=ORIENTED_EDGE ( 'NONE', *, *, #13408, .F. ) ;
#7904=CARTESIAN_POINT ( 'NONE',  ( -16.87183468716221313, -80.63143713290352821, -12.99038105676658539 ) ) ;
#7905=CARTESIAN_POINT ( 'NONE',  ( -35.14340807120437660, -83.52964452223220349, -21.65063509461098690 ) ) ;
#7906=DIRECTION ( 'NONE',  ( -0.1566598588826321192, 0.9876526153536342445, 7.798540720466730171E-17 ) ) ;
#7907=VECTOR ( 'NONE', #5181, 1000.000000000000000 ) ;
#7908=ORIENTED_EDGE ( 'NONE', *, *, #18226, .T. ) ;
#7910=ORIENTED_EDGE ( 'NONE', *, *, #12350, .T. ) ;
#7911=AXIS2_PLACEMENT_3D ( 'NONE', #1773, #6152, #16100 ) ;
#7915=DIRECTION ( 'NONE',  ( -0.1566598588826321192, 0.9876526153536342445, 7.798540720466730171E-17 ) ) ;
#7916=AXIS2_PLACEMENT_3D ( 'NONE', #17843, #8045, #13811 ) ;
#7917=FACE_OUTER_BOUND ( 'NONE', #1609, .T. ) ;
#7918=ADVANCED_FACE ( 'NONE', ( #9468 ), #15442, .F. ) ;
#7919=ORIENTED_EDGE ( 'NONE', *, *, #16789, .F. ) ;
#7920=EDGE_CURVE ( 'NONE', #15461, #16941, #3851, .T. ) ;
#7922=DIRECTION ( 'NONE',  ( -0.1566598588826321192, 0.9876526153536342445, 7.798540720466731404E-17 ) ) ;
#7923=AXIS2_PLACEMENT_3D ( 'NONE', #46, #17403, #4386 ) ;
#7924=CARTESIAN_POINT ( 'NONE',  ( -30.20514499443621759, -82.74634522781903456, -12.99038105676658539 ) ) ;
#7925=CARTESIAN_POINT ( 'NONE',  ( -20.65772683781411345, -18.46397219643515797, -17.32050807568878170 ) ) ;
#7926=VERTEX_POINT ( 'NONE', #13913 ) ;
#7927=ORIENTED_EDGE ( 'NONE', *, *, #5488, .F. ) ;
#7928=DIRECTION ( 'NONE',  ( 0.000000000000000000, 0.000000000000000000, 1.000000000000000000 ) ) ;
#7929=VERTEX_POINT ( 'NONE', #10767 ) ;
#7930=ORIENTED_EDGE ( 'NONE', *, *, #14580, .F. ) ;
#7931=CIRCLE ( 'NONE', #18577, 1.500000000000000888 ) ;
#7932=ORIENTED_EDGE ( 'NONE', *, *, #3193, .F. ) ;
#7933=LINE ( 'NONE', #825, #17906 ) ;
#7934=EDGE_LOOP ( 'NONE', ( #16899, #16526, #505, #18414 ) ) ;
#7935=AXIS2_PLACEMENT_3D ( 'NONE', #15745, #10134, #4165 ) ;
#7936=DIRECTION ( 'NONE',  ( -0.9876526153536341335, -0.1566598588826327021, 0.000000000000000000 ) ) ;
#7937=DIRECTION ( 'NONE',  ( -0.1566598588826321192, 0.9876526153536342445, 7.798540720466730171E-17 ) ) ;
#7938=ORIENTED_EDGE ( 'NONE', *, *, #7920, .T. ) ;
#7939=AXIS2_PLACEMENT_3D ( 'NONE', #7499, #13444, #1547 ) ;
#7940=CARTESIAN_POINT ( 'NONE',  ( -79.24244631363546887, 32.81909429640987952, 30.00000000000000000 ) ) ;
#7941=DIRECTION ( 'NONE',  ( -0.1566598588826321192, 0.9876526153536342445, 7.798540720466730171E-17 ) ) ;
#7944=EDGE_CURVE ( 'NONE', #4208, #7859, #17026, .T. ) ;
#7945=CIRCLE ( 'NONE', #371, 1.499999999999999556 ) ;
#7946=CARTESIAN_POINT ( 'NONE',  ( -30.73860631229088369, -25.12549372091224598, -4.330127018922181215 ) ) ;
#7947=FACE_OUTER_BOUND ( 'NONE', #18518, .T. ) ;
#7948=CARTESIAN_POINT ( 'NONE',  ( -2.057045456857760524, -78.28153924966404986, -4.330127018922185655 ) ) ;
#7949=EDGE_CURVE ( 'NONE', #6894, #4082, #9751, .T. ) ;
#7950=DIRECTION ( 'NONE',  ( -0.1566598588826321192, 0.9876526153536342445, 7.798540720466731404E-17 ) ) ;
#7951=ORIENTED_EDGE ( 'NONE', *, *, #11122, .F. ) ;
#7952=DIRECTION ( 'NONE',  ( -0.1566598588826321192, 0.9876526153536342445, 7.798540720466731404E-17 ) ) ;
#7955=DIRECTION ( 'NONE',  ( 0.000000000000000000, 0.000000000000000000, 1.000000000000000000 ) ) ;
#7956=CARTESIAN_POINT ( 'NONE',  ( -44.03228160938702018, -84.93958325217590755, 17.32050807568881368 ) ) ;
#7957=DIRECTION ( 'NONE',  ( -0.1566598588826321192, 0.9876526153536342445, 7.798540720466730171E-17 ) ) ;
#7958=FACE_OUTER_BOUND ( 'NONE', #8301, .T. ) ;
#7960=DIRECTION ( 'NONE',  ( -0.1566598588826321192, 0.9876526153536342445, 7.798540720466730171E-17 ) ) ;
#7961=DIRECTION ( 'NONE',  ( -0.1566598588826321192, 0.9876526153536342445, 7.798540720466731404E-17 ) ) ;
#7963=CARTESIAN_POINT ( 'NONE',  ( -40.08167114797249297, -84.31294381664537241, 21.65063509461101532 ) ) ;
#7965=VECTOR ( 'NONE', #1896, 1000.000000000000000 ) ;
#7966=EDGE_CURVE ( 'NONE', #14612, #7022, #6458, .T. ) ;
#7967=DIRECTION ( 'NONE',  ( -0.1566598588826321192, 0.9876526153536342445, 7.798540720466731404E-17 ) ) ;
#7968=DIRECTION ( 'NONE',  ( -0.9876526153536336894, -0.1566598588826349503, 0.000000000000000000 ) ) ;
#7969=ORIENTED_EDGE ( 'NONE', *, *, #17517, .F. ) ;
#7970=EDGE_CURVE ( 'NONE', #4208, #13075, #3569, .T. ) ;
#7971=VERTEX_POINT ( 'NONE', #2254 ) ;
#7972=EDGE_LOOP ( 'NONE', ( #6396, #2762, #4444, #3305 ) ) ;
#7975=FACE_BOUND ( 'NONE', #18012, .T. ) ;
#7976=CIRCLE ( 'NONE', #12504, 1.500000000000000888 ) ;
#7977=CARTESIAN_POINT ( 'NONE',  ( -30.69897130211303349, -82.82467515726035856, 7.308518362537324739E-15 ) ) ;
#7980=CARTESIAN_POINT ( 'NONE',  ( 2.000000000000000000, 2.449293598294706414E-16, -30.00000000000000000 ) ) ;
#7982=ORIENTED_EDGE ( 'NONE', *, *, #16319, .F. ) ;
#7983=LINE ( 'NONE', #16915, #17585 ) ;
#7984=DIRECTION ( 'NONE',  ( -0.1566598588826321192, 0.9876526153536342445, 7.798540720466730171E-17 ) ) ;
#7985=EDGE_CURVE ( 'NONE', #11183, #12777, #9127, .T. ) ;
#7986=EDGE_LOOP ( 'NONE', ( #7903, #14982, #7310, #3419 ) ) ;
#7988=CARTESIAN_POINT ( 'NONE',  ( -65.30644784966793281, -30.60858878180435738, -4.330127018922181215 ) ) ;
#7989=EDGE_CURVE ( 'NONE', #18620, #8246, #5193, .T. ) ;
#7991=DIRECTION ( 'NONE',  ( -0.1566598588826321192, 0.9876526153536342445, 7.798540720466731404E-17 ) ) ;
#7992=VERTEX_POINT ( 'NONE', #15532 ) ;
#7993=ORIENTED_EDGE ( 'NONE', *, *, #24, .T. ) ;
#7994=CARTESIAN_POINT ( 'NONE',  ( 7.819480696678544618, -76.71494066083772623, -21.65063509461098690 ) ) ;
#7995=EDGE_LOOP ( 'NONE', ( #8921, #8073, #5904, #3026 ) ) ;
#7996=DIRECTION ( 'NONE',  ( -0.9876526153536341335, -0.1566598588826327021, 0.000000000000000000 ) ) ;
#7998=EDGE_LOOP ( 'NONE', ( #759, #16404 ) ) ;
#7999=CARTESIAN_POINT ( 'NONE',  ( -14.23798483801550674, -17.44568311369805613, -17.32050807568878170 ) ) ;
#8000=DIRECTION ( 'NONE',  ( 0.000000000000000000, 0.000000000000000000, 1.000000000000000000 ) ) ;
#8002=DIRECTION ( 'NONE',  ( 0.000000000000000000, 0.000000000000000000, 1.000000000000000000 ) ) ;
#8003=CIRCLE ( 'NONE', #6824, 1.500000000000000888 ) ;
#8005=CARTESIAN_POINT ( 'NONE',  ( 3.133606229046292935, -19.12225244224100962, -24.99999999999999289 ) ) ;
#8007=EDGE_CURVE ( 'NONE', #8907, #13690, #10024, .T. ) ;
#8008=VERTEX_POINT ( 'NONE', #6925 ) ;
#8009=ORIENTED_EDGE ( 'NONE', *, *, #14993, .F. ) ;
#8010=CARTESIAN_POINT ( 'NONE',  ( -52.26261052913027072, -23.47708768067937513, -17.32050807568878170 ) ) ;
#8011=ORIENTED_EDGE ( 'NONE', *, *, #8909, .T. ) ;
#8013=ORIENTED_EDGE ( 'NONE', *, *, #7104, .F. ) ;
#8014=EDGE_CURVE ( 'NONE', #9857, #8644, #14867, .T. ) ;
#8016=AXIS2_PLACEMENT_3D ( 'NONE', #7375, #8688, #17345 ) ;
#8017=CARTESIAN_POINT ( 'NONE',  ( -59.67000514428248437, -24.65203662229911430, -12.99038105676658006 ) ) ;
#8018=DIRECTION ( 'NONE',  ( -0.1566598588826321192, 0.9876526153536342445, 7.798540720466731404E-17 ) ) ;
#8019=VERTEX_POINT ( 'NONE', #8620 ) ;
#8020=LINE ( 'NONE', #6811, #14345 ) ;
#8021=DIRECTION ( 'NONE',  ( -1.000000000000000000, 0.000000000000000000, 0.000000000000000000 ) ) ;
#8023=LINE ( 'NONE', #9257, #6021 ) ;
#8024=DIRECTION ( 'NONE',  ( -0.1566598588826321192, 0.9876526153536342445, 7.798540720466730171E-17 ) ) ;
#8025=FACE_BOUND ( 'NONE', #14692, .T. ) ;
#8026=CARTESIAN_POINT ( 'NONE',  ( -19.34096622554629263, -81.02308678011010556, -8.660254037844385522 ) ) ;
#8028=AXIS2_PLACEMENT_3D ( 'NONE', #324, #15087, #6304 ) ;
#8029=ORIENTED_EDGE ( 'NONE', *, *, #8104, .T. ) ;
#8030=DIRECTION ( 'NONE',  ( -0.9876526153536336894, -0.1566598588826350336, 0.000000000000000000 ) ) ;
#8031=EDGE_LOOP ( 'NONE', ( #9835, #9736, #1763, #9465 ) ) ;
#8033=EDGE_CURVE ( 'NONE', #4998, #11150, #5590, .T. ) ;
#8034=ORIENTED_EDGE ( 'NONE', *, *, #16407, .T. ) ;
#8035=ORIENTED_EDGE ( 'NONE', *, *, #4651, .F. ) ;
#8037=CIRCLE ( 'NONE', #12267, 1.500000000000000888 ) ;
#8038=CARTESIAN_POINT ( 'NONE',  ( -3.538524379888211335, -78.51652903798800764, -21.65063509461098690 ) ) ;
#8039=DIRECTION ( 'NONE',  ( -0.1566598588826321192, 0.9876526153536342445, 7.798540720466730171E-17 ) ) ;
#8041=EDGE_CURVE ( 'NONE', #11968, #12573, #14101, .T. ) ;
#8042=CARTESIAN_POINT ( 'NONE',  ( -65.26681283949008616, -88.30777021815248418, 8.660254037844412167 ) ) ;
#8043=CIRCLE ( 'NONE', #18698, 1.500000000000000444 ) ;
#8044=ORIENTED_EDGE ( 'NONE', *, *, #15952, .F. ) ;
#8045=DIRECTION ( 'NONE',  ( -0.1566598588826321747, 0.9876526153536343555, 0.000000000000000000 ) ) ;
#8046=CARTESIAN_POINT ( 'NONE',  ( -19.17624791478365864, -18.22898240811121440, -17.32050807568878170 ) ) ;
#8048=CARTESIAN_POINT ( 'NONE',  ( -76.17062661855784711, -32.33184722951329348, 1.887572821959364500E-14 ) ) ;
#8049=ORIENTED_EDGE ( 'NONE', *, *, #6023, .F. ) ;
#8051=DIRECTION ( 'NONE',  ( 0.000000000000000000, 0.000000000000000000, 1.000000000000000000 ) ) ;
#8052=AXIS2_PLACEMENT_3D ( 'NONE', #17091, #16, #8637 ) ;
#8053=CARTESIAN_POINT ( 'NONE',  ( -3.578159390066044665, -20.81734760163988440, -17.32050807568878170 ) ) ;
#8054=CYLINDRICAL_SURFACE ( 'NONE', #18178, 1.500000000000001554 ) ;
#8055=VERTEX_POINT ( 'NONE', #18526 ) ;
#8056=CIRCLE ( 'NONE', #2302, 144.0000000000000284 ) ;
#8057=ORIENTED_EDGE ( 'NONE', *, *, #1018, .T. ) ;
#8058=ORIENTED_EDGE ( 'NONE', *, *, #8953, .F. ) ;
#8059=VERTEX_POINT ( 'NONE', #11253 ) ;
#8060=CARTESIAN_POINT ( 'NONE',  ( -60.32854976272193426, -87.52447092373932946, 17.32050807568881368 ) ) ;
#8061=FACE_BOUND ( 'NONE', #7677, .T. ) ;
#8062=AXIS2_PLACEMENT_3D ( 'NONE', #16126, #16204, #386 ) ;
#8063=EDGE_CURVE ( 'NONE', #1063, #17245, #6724, .T. ) ;
#8065=EDGE_LOOP ( 'NONE', ( #11589, #4812 ) ) ;
#8066=EDGE_CURVE ( 'NONE', #7806, #14381, #10636, .T. ) ;
#8068=EDGE_LOOP ( 'NONE', ( #16852, #10719, #16686, #9216 ) ) ;
#8069=EDGE_CURVE ( 'NONE', #3169, #1267, #17074, .T. ) ;
#8072=CIRCLE ( 'NONE', #10194, 1.500000000000000888 ) ;
#8073=ORIENTED_EDGE ( 'NONE', *, *, #11006, .T. ) ;
#8074=ORIENTED_EDGE ( 'NONE', *, *, #18344, .F. ) ;
#8075=DIRECTION ( 'NONE',  ( -0.1566598588826321192, 0.9876526153536342445, 7.798540720466730171E-17 ) ) ;
#8076=CARTESIAN_POINT ( 'NONE',  ( 2.841582609732560272, -19.79905851890276836, -17.32050807568878170 ) ) ;
#8077=CARTESIAN_POINT ( 'NONE',  ( -32.67427653282028643, -83.13799487502562613, -8.660254037844385522 ) ) ;
#8079=ORIENTED_EDGE ( 'NONE', *, *, #11202, .T. ) ;
#8080=CARTESIAN_POINT ( 'NONE',  ( -31.68662391746665463, -82.98133501614300656, 12.99038105676661203 ) ) ;
#8081=AXIS2_PLACEMENT_3D ( 'NONE', #14546, #7261, #8381 ) ;
#8083=CARTESIAN_POINT ( 'NONE',  ( -65.10209452872746283, -25.51366584615358946, 1.908195823574487804E-14 ) ) ;
#8085=DIRECTION ( 'NONE',  ( -0.9876526153536336894, -0.1566598588826349503, 0.000000000000000000 ) ) ;
#8086=AXIS2_PLACEMENT_3D ( 'NONE', #7527, #4763, #4666 ) ;
#8087=DIRECTION ( 'NONE',  ( 0.000000000000000000, 0.000000000000000000, 1.000000000000000000 ) ) ;
#8088=EDGE_CURVE ( 'NONE', #8327, #18200, #1421, .T. ) ;
#8089=DIRECTION ( 'NONE',  ( -0.1566598588826321747, 0.9876526153536343555, 0.000000000000000000 ) ) ;
#8091=CARTESIAN_POINT ( 'NONE',  ( -34.15575545585074480, -83.37298466334958391, -17.32050807568878525 ) ) ;
#8093=ADVANCED_FACE ( 'NONE', ( #18709 ), #8422, .F. ) ;
#8095=LINE ( 'NONE', #8300, #2025 ) ;
#8097=AXIS2_PLACEMENT_3D ( 'NONE', #14456, #12835, #14553 ) ;
#8098=DIRECTION ( 'NONE',  ( -0.9876526153536341335, -0.1566598588826327021, 0.000000000000000000 ) ) ;
#8100=DIRECTION ( 'NONE',  ( -0.9876526153536336894, -0.1566598588826349503, 0.000000000000000000 ) ) ;
#8102=ORIENTED_EDGE ( 'NONE', *, *, #16946, .T. ) ;
#8104=EDGE_CURVE ( 'NONE', #12986, #15683, #4044, .T. ) ;
#8105=DIRECTION ( 'NONE',  ( -0.9876526153536341335, -0.1566598588826327021, 0.000000000000000000 ) ) ;
#8106=CARTESIAN_POINT ( 'NONE',  ( -14.23798483801550674, -17.44568311369805969, 8.660254037844413944 ) ) ;
#8109=CIRCLE ( 'NONE', #18753, 1.500000000000001332 ) ;
#8110=CARTESIAN_POINT ( 'NONE',  ( -37.94164760650263446, -21.20551972688121722, -4.330127018922180326 ) ) ;
#8111=ORIENTED_EDGE ( 'NONE', *, *, #17511, .F. ) ;
#8112=ORIENTED_EDGE ( 'NONE', *, *, #1298, .T. ) ;
#8113=DIRECTION ( 'NONE',  ( -0.1566598588826321192, 0.9876526153536342445, 7.798540720466730171E-17 ) ) ;
#8114=DIRECTION ( 'NONE',  ( -0.1566598588826321747, 0.9876526153536343555, 0.000000000000000000 ) ) ;
#8116=DIRECTION ( 'NONE',  ( -0.9876526153536336894, -0.1566598588826349503, 0.000000000000000000 ) ) ;
#8117=CARTESIAN_POINT ( 'NONE',  ( -62.13913668266656032, -25.04368626950569166, -17.32050807568878170 ) ) ;
#8118=EDGE_CURVE ( 'NONE', #5059, #5250, #2635, .T. ) ;
#8119=AXIS2_PLACEMENT_3D ( 'NONE', #2355, #6743, #8148 ) ;
#8120=ORIENTED_EDGE ( 'NONE', *, *, #5322, .F. ) ;
#8121=EDGE_CURVE ( 'NONE', #1541, #18619, #17356, .T. ) ;
#8122=CYLINDRICAL_SURFACE ( 'NONE', #6678, 1.500000000000001554 ) ;
#8123=VERTEX_POINT ( 'NONE', #11612 ) ;
#8125=DIRECTION ( 'NONE',  ( -0.9876526153536336894, -0.1566598588826350336, 0.000000000000000000 ) ) ;
#8126=CARTESIAN_POINT ( 'NONE',  ( -48.97054468615519340, -85.72288254658904805, -8.660254037844385522 ) ) ;
#8127=CIRCLE ( 'NONE', #18145, 1.500000000000000444 ) ;
#8128=DIRECTION ( 'NONE',  ( -0.1566598588826321192, 0.9876526153536342445, 7.798540720466730171E-17 ) ) ;
#8130=CARTESIAN_POINT ( 'NONE',  ( -4.565812005419673802, -20.97400746052251108, 21.65063509461101177 ) ) ;
#8132=CIRCLE ( 'NONE', #7241, 1.500000000000000888 ) ;
#8133=DIRECTION ( 'NONE',  ( -0.9876526153536344665, -0.1566598588826304539, 0.000000000000000000 ) ) ;
#8134=VERTEX_POINT ( 'NONE', #15712 ) ;
#8135=CARTESIAN_POINT ( 'NONE',  ( -33.20773785067495254, -25.51714336811882688, 1.869203119972154228E-14 ) ) ;
#8136=CARTESIAN_POINT ( 'NONE',  ( -41.56315007100297265, -84.54793360496931598, -21.65063509461098690 ) ) ;
#8138=ORIENTED_EDGE ( 'NONE', *, *, #2111, .F. ) ;
#8140=AXIS2_PLACEMENT_3D ( 'NONE', #14244, #9966, #12812 ) ;
#8141=CARTESIAN_POINT ( 'NONE',  ( -13.45468554360235203, -22.38394619046619383, 17.32050807568881012 ) ) ;
#8142=AXIS2_PLACEMENT_3D ( 'NONE', #5405, #5308, #16891 ) ;
#8143=FACE_OUTER_BOUND ( 'NONE', #497, .T. ) ;
#8144=DIRECTION ( 'NONE',  ( -0.1566598588826321747, 0.9876526153536343555, 0.000000000000000000 ) ) ;
#8145=CIRCLE ( 'NONE', #7556, 1.500000000000000888 ) ;
#8146=ORIENTED_EDGE ( 'NONE', *, *, #1580, .F. ) ;
#8148=DIRECTION ( 'NONE',  ( -0.9876526153536336894, -0.1566598588826350336, 0.000000000000000000 ) ) ;
#8149=CYLINDRICAL_SURFACE ( 'NONE', #889, 1.500000000000001554 ) ;
#8150=DIRECTION ( 'NONE',  ( -0.1566598588826321192, 0.9876526153536342445, 7.798540720466730171E-17 ) ) ;
#8152=CARTESIAN_POINT ( 'NONE',  ( -27.57129514528951120, -19.56059120861359446, 8.660254037844417496 ) ) ;
#8153=ORIENTED_EDGE ( 'NONE', *, *, #6391, .F. ) ;
#8154=EDGE_CURVE ( 'NONE', #999, #334, #7619, .T. ) ;
#8155=CIRCLE ( 'NONE', #11165, 1.500000000000000888 ) ;
#8158=CARTESIAN_POINT ( 'NONE',  ( -63.62061560569699736, -25.27867605782964944, 17.32050807568882078 ) ) ;
#8159=VECTOR ( 'NONE', #18348, 1000.000000000000000 ) ;
#8160=VECTOR ( 'NONE', #6135, 1000.000000000000000 ) ;
#8164=EDGE_LOOP ( 'NONE', ( #5141, #16798 ) ) ;
#8166=DIRECTION ( 'NONE',  ( -0.1566598588826321192, 0.9876526153536342445, 7.798540720466730171E-17 ) ) ;
#8167=FACE_BOUND ( 'NONE', #12601, .T. ) ;
#8168=AXIS2_PLACEMENT_3D ( 'NONE', #14055, #14154, #1196 ) ;
#8170=EDGE_LOOP ( 'NONE', ( #6969, #11492, #1562, #3336 ) ) ;
#8173=CARTESIAN_POINT ( 'NONE',  ( -13.45468554360235203, -22.38394619046619383, 8.660254037844413944 ) ) ;
#8175=EDGE_LOOP ( 'NONE', ( #6041, #184, #1929, #15160 ) ) ;
#8176=DIRECTION ( 'NONE',  ( -0.9876526153536341335, -0.1566598588826327021, 0.000000000000000000 ) ) ;
#8179=DIRECTION ( 'NONE',  ( 0.000000000000000000, 0.000000000000000000, 1.000000000000000000 ) ) ;
#8180=DIRECTION ( 'NONE',  ( -0.1566598588826321192, 0.9876526153536342445, 7.798540720466730171E-17 ) ) ;
#8181=DIRECTION ( 'NONE',  ( -0.9876526153536336894, -0.1566598588826349503, 0.000000000000000000 ) ) ;
#8182=ORIENTED_EDGE ( 'NONE', *, *, #5810, .F. ) ;
#8183=DIRECTION ( 'NONE',  ( -0.1566598588826321192, 0.9876526153536342445, 7.798540720466730171E-17 ) ) ;
#8184=EDGE_CURVE ( 'NONE', #8789, #5011, #11699, .T. ) ;
#8185=CARTESIAN_POINT ( 'NONE',  ( -67.77557938805200877, -31.00023842901093118, 8.660254037844417496 ) ) ;
#8186=AXIS2_PLACEMENT_3D ( 'NONE', #7020, #18516, #6624 ) ;
#8187=DIRECTION ( 'NONE',  ( -0.9876526153536341335, -0.1566598588826327021, 0.000000000000000000 ) ) ;
#8188=ORIENTED_EDGE ( 'NONE', *, *, #2521, .F. ) ;
#8189=ORIENTED_EDGE ( 'NONE', *, *, #1377, .F. ) ;
#8190=AXIS2_PLACEMENT_3D ( 'NONE', #10993, #6675, #12518 ) ;
#8191=DIRECTION ( 'NONE',  ( -0.1566598588826321192, 0.9876526153536342445, 7.798540720466730171E-17 ) ) ;
#8192=CYLINDRICAL_SURFACE ( 'NONE', #666, 1.500000000000001554 ) ;
#8193=EDGE_CURVE ( 'NONE', #1545, #4233, #13052, .T. ) ;
#8194=DIRECTION ( 'NONE',  ( -0.9876526153536341335, -0.1566598588826327021, 0.000000000000000000 ) ) ;
#8195=VECTOR ( 'NONE', #3620, 1000.000000000000000 ) ;
#8196=CARTESIAN_POINT ( 'NONE',  ( -52.75643683680708307, -23.55541761012069202, -4.330127018922180326 ) ) ;
#8197=AXIS2_PLACEMENT_3D ( 'NONE', #6141, #10469, #16266 ) ;
#8198=LINE ( 'NONE', #13967, #8483 ) ;
#8199=DIRECTION ( 'NONE',  ( -0.9876526153536341335, -0.1566598588826327021, 0.000000000000000000 ) ) ;
#8202=CARTESIAN_POINT ( 'NONE',  ( -15.22563745336913144, -17.60234297258068636, -21.65063509461098334 ) ) ;
#8204=AXIS2_PLACEMENT_3D ( 'NONE', #10942, #6606, #15312 ) ;
#8205=DIRECTION ( 'NONE',  ( -0.1566598588826321192, 0.9876526153536342445, 7.798540720466731404E-17 ) ) ;
#8206=ORIENTED_EDGE ( 'NONE', *, *, #6482, .T. ) ;
#8207=VERTEX_POINT ( 'NONE', #10199 ) ;
#8208=DIRECTION ( 'NONE',  ( -0.9876526153536341335, -0.1566598588826327021, 0.000000000000000000 ) ) ;
#8209=EDGE_CURVE ( 'NONE', #5983, #3731, #7337, .T. ) ;
#8211=VECTOR ( 'NONE', #11480, 1000.000000000000000 ) ;
#8212=ORIENTED_EDGE ( 'NONE', *, *, #17684, .T. ) ;
#8213=AXIS2_PLACEMENT_3D ( 'NONE', #11220, #12254, #18203 ) ;
#8214=VERTEX_POINT ( 'NONE', #545 ) ;
#8215=DIRECTION ( 'NONE',  ( -0.9876526153536341335, -0.1566598588826327021, 0.000000000000000000 ) ) ;
#8217=AXIS2_PLACEMENT_3D ( 'NONE', #12645, #18505, #8316 ) ;
#8218=DIRECTION ( 'NONE',  ( -0.9876526153536336894, -0.1566598588826350336, 0.000000000000000000 ) ) ;
#8220=DIRECTION ( 'NONE',  ( -0.9876526153536336894, -0.1566598588826349503, 0.000000000000000000 ) ) ;
#8221=DIRECTION ( 'NONE',  ( -0.9876526153536341335, -0.1566598588826327576, 0.000000000000000000 ) ) ;
#8224=AXIS2_PLACEMENT_3D ( 'NONE', #5497, #15820, #9844 ) ;
#8226=ORIENTED_EDGE ( 'NONE', *, *, #6239, .F. ) ;
#8227=CIRCLE ( 'NONE', #12127, 1.500000000000001332 ) ;
#8229=DIRECTION ( 'NONE',  ( -0.9876526153536341335, -0.1566598588826327021, 0.000000000000000000 ) ) ;
#8230=VERTEX_POINT ( 'NONE', #11795 ) ;
#8231=EDGE_CURVE ( 'NONE', #10127, #6097, #527, .T. ) ;
#8232=CYLINDRICAL_SURFACE ( 'NONE', #18090, 1.500000000000001554 ) ;
#8234=ORIENTED_EDGE ( 'NONE', *, *, #18226, .F. ) ;
#8237=CARTESIAN_POINT ( 'NONE',  ( -6.007655918272284623, -78.90817868519457079, 1.424741226644455312E-14 ) ) ;
#8238=ORIENTED_EDGE ( 'NONE', *, *, #11575, .T. ) ;
#8239=AXIS2_PLACEMENT_3D ( 'NONE', #2846, #15633, #17093 ) ;
#8240=EDGE_CURVE ( 'NONE', #5485, #3473, #6898, .T. ) ;
#8242=EDGE_CURVE ( 'NONE', #4549, #12880, #4612, .T. ) ;
#8243=CARTESIAN_POINT ( 'NONE',  ( -11.93357161039406300, -79.84813783849035929, -21.65063509461098690 ) ) ;
#8244=ORIENTED_EDGE ( 'NONE', *, *, #9562, .T. ) ;
#8245=EDGE_CURVE ( 'NONE', #442, #6801, #11690, .T. ) ;
#8246=VERTEX_POINT ( 'NONE', #13138 ) ;
#8247=CIRCLE ( 'NONE', #4307, 1.500000000000000888 ) ;
#8248=CARTESIAN_POINT ( 'NONE',  ( 0.3724510713484854851, -20.19070816610934926, 4.330127018922212301 ) ) ;
#8249=CARTESIAN_POINT ( 'NONE',  ( -46.50141314777111745, -85.33123289938247069, -12.99038105676658539 ) ) ;
#8250=EDGE_CURVE ( 'NONE', #10116, #13151, #216, .T. ) ;
#8251=VERTEX_POINT ( 'NONE', #168 ) ;
#8252=DIRECTION ( 'NONE',  ( -1.000000000000000000, 0.000000000000000000, 0.000000000000000000 ) ) ;
#8254=DIRECTION ( 'NONE',  ( -0.1566598588826321192, 0.9876526153536342445, 7.798540720466731404E-17 ) ) ;
#8255=DIRECTION ( 'NONE',  ( -0.1566598588826321747, 0.9876526153536343555, 0.000000000000000000 ) ) ;
#8256=CARTESIAN_POINT ( 'NONE',  ( -40.61513246582718750, -26.69209230973856251, -12.99038105676658006 ) ) ;
#8257=EDGE_LOOP ( 'NONE', ( #7606, #13871 ) ) ;
#8258=DIRECTION ( 'NONE',  ( -0.1566598588826321192, 0.9876526153536342445, 7.798540720466730171E-17 ) ) ;
#8259=AXIS2_PLACEMENT_3D ( 'NONE', #14318, #12787, #5600 ) ;
#8261=CARTESIAN_POINT ( 'NONE',  ( -79.13358446461874962, -32.80182680616118773, -8.660254037844380193 ) ) ;
#8262=EDGE_CURVE ( 'NONE', #1456, #2063, #7663, .T. ) ;
#8264=EDGE_LOOP ( 'NONE', ( #15990, #13116, #14199, #7694 ) ) ;
#8265=CARTESIAN_POINT ( 'NONE',  ( -53.94844277310118486, -28.80700040465408662, -12.99038105676658006 ) ) ;
#8266=AXIS2_PLACEMENT_3D ( 'NONE', #12978, #5976, #14233 ) ;
#8268=ORIENTED_EDGE ( 'NONE', *, *, #5792, .F. ) ;
#8269=CARTESIAN_POINT ( 'NONE',  ( -72.50948914387967648, -26.68861478777332508, -4.330127018922180326 ) ) ;
#8270=EDGE_CURVE ( 'NONE', #13292, #7705, #12072, .T. ) ;
#8271=EDGE_CURVE ( 'NONE', #2601, #7195, #10385, .T. ) ;
#8272=FACE_BOUND ( 'NONE', #5043, .T. ) ;
#8275=VERTEX_POINT ( 'NONE', #4518 ) ;
#8276=AXIS2_PLACEMENT_3D ( 'NONE', #5211, #18433, #10966 ) ;
#8278=VERTEX_POINT ( 'NONE', #16098 ) ;
#8280=DIRECTION ( 'NONE',  ( -0.1566598588826321747, 0.9876526153536343555, 0.000000000000000000 ) ) ;
#8281=CARTESIAN_POINT ( 'NONE',  ( 10.28861223506262412, -76.32329101363113466, 9.043241838514131834E-15 ) ) ;
#8282=DIRECTION ( 'NONE',  ( -0.9876526153536341335, -0.1566598588826327021, 0.000000000000000000 ) ) ;
#8283=VERTEX_POINT ( 'NONE', #1959 ) ;
#8285=DIRECTION ( 'NONE',  ( -0.1566598588826321192, 0.9876526153536342445, 7.798540720466730171E-17 ) ) ;
#8286=VERTEX_POINT ( 'NONE', #3174 ) ;
#8287=VERTEX_POINT ( 'NONE', #13497 ) ;
#8288=CARTESIAN_POINT ( 'NONE',  ( -3.538524379888208227, -78.51652903798800764, 21.65063509461100821 ) ) ;
#8289=CIRCLE ( 'NONE', #110, 1.499999999999999556 ) ;
#8291=LINE ( 'NONE', #16743, #11522 ) ;
#8293=CARTESIAN_POINT ( 'NONE',  ( -54.89646037827696290, -86.66284169988485075, 12.99038105676661203 ) ) ;
#8296=EDGE_CURVE ( 'NONE', #8123, #1233, #11885, .T. ) ;
#8299=CARTESIAN_POINT ( 'NONE',  ( 3.231158466157554976, 19.73726462726228092, -24.99999999999998934 ) ) ;
#8300=CARTESIAN_POINT ( 'NONE',  ( -12.92122422574768592, -80.00479769737299307, 1.443110928631665584E-14 ) ) ;
#8301=EDGE_LOOP ( 'NONE', ( #17859, #11855, #4162, #8528 ) ) ;
#8302=DIRECTION ( 'NONE',  ( -0.1566598588826321192, 0.9876526153536342445, 7.798540720466730171E-17 ) ) ;
#8303=ORIENTED_EDGE ( 'NONE', *, *, #15529, .F. ) ;
#8304=VERTEX_POINT ( 'NONE', #2237 ) ;
#8305=FACE_BOUND ( 'NONE', #3711, .T. ) ;
#8307=EDGE_LOOP ( 'NONE', ( #15793, #11818, #8387, #13130 ) ) ;
#8310=VERTEX_POINT ( 'NONE', #1041 ) ;
#8311=EDGE_LOOP ( 'NONE', ( #11322, #5901 ) ) ;
#8312=LINE ( 'NONE', #2323, #1844 ) ;
#8313=DIRECTION ( 'NONE',  ( 0.000000000000000000, 0.000000000000000000, 1.000000000000000000 ) ) ;
#8315=ADVANCED_FACE ( 'NONE', ( #17919 ), #13779, .F. ) ;
#8316=DIRECTION ( 'NONE',  ( -0.9876526153536336894, -0.1566598588826349503, 0.000000000000000000 ) ) ;
#8317=DIRECTION ( 'NONE',  ( -0.9876526153536341335, -0.1566598588826327021, 0.000000000000000000 ) ) ;
#8318=( LENGTH_UNIT ( ) NAMED_UNIT ( * ) SI_UNIT ( .MILLI., .METRE. ) );
#8319=FACE_OUTER_BOUND ( 'NONE', #10266, .T. ) ;
#8320=EDGE_LOOP ( 'NONE', ( #2845, #6481, #15057, #1163 ) ) ;
#8321=DIRECTION ( 'NONE',  ( 0.000000000000000000, 0.000000000000000000, 1.000000000000000000 ) ) ;
#8322=EDGE_CURVE ( 'NONE', #6756, #17136, #16886, .T. ) ;
#8325=DIRECTION ( 'NONE',  ( -0.1566598588826321192, 0.9876526153536342445, 7.798540720466731404E-17 ) ) ;
#8326=DIRECTION ( 'NONE',  ( -0.1566598588826321747, 0.9876526153536343555, 0.000000000000000000 ) ) ;
#8327=VERTEX_POINT ( 'NONE', #18213 ) ;
#8329=AXIS2_PLACEMENT_3D ( 'NONE', #17677, #6279, #399 ) ;
#8331=ORIENTED_EDGE ( 'NONE', *, *, #16368, .F. ) ;
#8333=VERTEX_POINT ( 'NONE', #8017 ) ;
#8334=CARTESIAN_POINT ( 'NONE',  ( -32.67427653282028643, -83.13799487502562613, -17.32050807568878525 ) ) ;
#8336=CARTESIAN_POINT ( 'NONE',  ( -66.08974714408108753, -25.67032570503621258, -21.65063509461097979 ) ) ;
#8337=CARTESIAN_POINT ( 'NONE',  ( -42.87991068327077926, -21.98881902129438259, 12.99038105676661736 ) ) ;
#8338=EDGE_LOOP ( 'NONE', ( #5724, #3369, #12215, #17806 ) ) ;
#8339=CARTESIAN_POINT ( 'NONE',  ( -6.995308533625909320, -79.06483854407721878, 12.99038105676660848 ) ) ;
#8341=EDGE_CURVE ( 'NONE', #16044, #15425, #14140, .T. ) ;
#8342=EDGE_CURVE ( 'NONE', #4043, #7702, #11390, .T. ) ;
#8343=DIRECTION ( 'NONE',  ( -0.1566598588826321747, 0.9876526153536343555, 0.000000000000000000 ) ) ;
#8344=AXIS2_PLACEMENT_3D ( 'NONE', #10933, #6992, #16940 ) ;
#8345=DIRECTION ( 'NONE',  ( 0.000000000000000000, 0.000000000000000000, 1.000000000000000000 ) ) ;
#8346=EDGE_CURVE ( 'NONE', #16242, #1233, #10485, .T. ) ;
#8347=DIRECTION ( 'NONE',  ( -0.000000000000000000, -0.000000000000000000, -1.000000000000000000 ) ) ;
#8348=VERTEX_POINT ( 'NONE', #11032 ) ;
#8349=VERTEX_POINT ( 'NONE', #10672 ) ;
#8350=CARTESIAN_POINT ( 'NONE',  ( -13.25033222266188915, -17.28902325481541880, -21.65063509461098334 ) ) ;
#8352=FACE_BOUND ( 'NONE', #9553, .T. ) ;
#8353=ADVANCED_FACE ( 'NONE', ( #6521 ), #5067, .F. ) ;
#8354=DIRECTION ( 'NONE',  ( -0.1566598588826321192, 0.9876526153536342445, 7.798540720466730171E-17 ) ) ;
#8355=EDGE_CURVE ( 'NONE', #15832, #5613, #13603, .T. ) ;
#8356=EDGE_CURVE ( 'NONE', #405, #16739, #18727, .T. ) ;
#8357=AXIS2_PLACEMENT_3D ( 'NONE', #3764, #5220, #9569 ) ;
#8359=FACE_OUTER_BOUND ( 'NONE', #10029, .T. ) ;
#8360=CARTESIAN_POINT ( 'NONE',  ( -70.20507591625822386, -89.09106951256563889, -17.32050807568878525 ) ) ;
#8361=VECTOR ( 'NONE', #3765, 1000.000000000000000 ) ;
#8362=CYLINDRICAL_SURFACE ( 'NONE', #14234, 1.500000000000001554 ) ;
#8363=DIRECTION ( 'NONE',  ( 0.000000000000000000, 0.000000000000000000, 1.000000000000000000 ) ) ;
#8364=VERTEX_POINT ( 'NONE', #12473 ) ;
#8366=DIRECTION ( 'NONE',  ( -0.1566598588826321192, 0.9876526153536342445, 7.798540720466731404E-17 ) ) ;
#8367=ORIENTED_EDGE ( 'NONE', *, *, #15094, .F. ) ;
#8368=VERTEX_POINT ( 'NONE', #10841 ) ;
#8369=ORIENTED_EDGE ( 'NONE', *, *, #2582, .F. ) ;
#8370=DIRECTION ( 'NONE',  ( -0.1566598588826321747, 0.9876526153536343555, 0.000000000000000000 ) ) ;
#8371=AXIS2_PLACEMENT_3D ( 'NONE', #15260, #882, #3497 ) ;
#8373=FACE_OUTER_BOUND ( 'NONE', #13560, .T. ) ;
#8374=CARTESIAN_POINT ( 'NONE',  ( -79.13358446461874962, -32.80182680616118773, 17.32050807568881723 ) ) ;
#8375=VECTOR ( 'NONE', #4119, 1000.000000000000000 ) ;
#8376=CARTESIAN_POINT ( 'NONE',  ( 1.893565004556770903, -77.65489981413351472, 17.32050807568880657 ) ) ;
#8378=CARTESIAN_POINT ( 'NONE',  ( -61.31620237807555895, -87.68113078262196325, 21.65063509461101532 ) ) ;
#8379=AXIS2_PLACEMENT_3D ( 'NONE', #15002, #2018, #423 ) ;
#8381=DIRECTION ( 'NONE',  ( -1.000000000000000000, 0.000000000000000000, -3.208277787129350839E-17 ) ) ;
#8382=EDGE_CURVE ( 'NONE', #1532, #14684, #3819, .T. ) ;
#8383=FACE_OUTER_BOUND ( 'NONE', #351, .T. ) ;
#8384=DIRECTION ( 'NONE',  ( 0.000000000000000000, 0.000000000000000000, 1.000000000000000000 ) ) ;
#8385=ORIENTED_EDGE ( 'NONE', *, *, #3380, .T. ) ;
#8386=EDGE_CURVE ( 'NONE', #2695, #15443, #4218, .T. ) ;
#8387=ORIENTED_EDGE ( 'NONE', *, *, #219, .T. ) ;
#8388=FACE_OUTER_BOUND ( 'NONE', #1261, .T. ) ;
#8389=CARTESIAN_POINT ( 'NONE',  ( -50.28730529842301422, -23.16376796291411466, 1.908195823574487804E-14 ) ) ;
#8390=ORIENTED_EDGE ( 'NONE', *, *, #12216, .T. ) ;
#8391=AXIS2_PLACEMENT_3D ( 'NONE', #4983, #7952, #15049 ) ;
#8392=ADVANCED_FACE ( 'NONE', ( #15219 ), #16772, .F. ) ;
#8393=CYLINDRICAL_SURFACE ( 'NONE', #9994, 1.500000000000001554 ) ;
#8394=AXIS2_PLACEMENT_3D ( 'NONE', #6339, #3002, #4790 ) ;
#8395=ORIENTED_EDGE ( 'NONE', *, *, #5322, .T. ) ;
#8397=AXIS2_PLACEMENT_3D ( 'NONE', #17151, #9758, #2541 ) ;
#8398=CARTESIAN_POINT ( 'NONE',  ( -61.15148406731292852, -24.88702641062307208, 21.65063509461102242 ) ) ;
#8399=VERTEX_POINT ( 'NONE', #8117 ) ;
#8400=DIRECTION ( 'NONE',  ( -0.1566598588826321747, 0.9876526153536343555, 0.000000000000000000 ) ) ;
#8401=CARTESIAN_POINT ( 'NONE',  ( -8.516422466834198346, -21.60064689605303911, -8.660254037844380193 ) ) ;
#8403=CARTESIAN_POINT ( 'NONE',  ( -9.464440072009985272, -79.45648819128378193, 1.424741226644455312E-14 ) ) ;
#8405=CIRCLE ( 'NONE', #13519, 1.499999999999999556 ) ;
#8406=DIRECTION ( 'NONE',  ( -0.9876526153536336894, -0.1566598588826350336, 0.000000000000000000 ) ) ;
#8408=DIRECTION ( 'NONE',  ( 0.000000000000000000, 0.000000000000000000, 1.000000000000000000 ) ) ;
#8409=DIRECTION ( 'NONE',  ( -0.1566598588826321747, 0.9876526153536343555, 0.000000000000000000 ) ) ;
#8411=ORIENTED_EDGE ( 'NONE', *, *, #10984, .F. ) ;
#8412=LINE ( 'NONE', #12764, #18212 ) ;
#8414=CARTESIAN_POINT ( 'NONE',  ( -60.16383145195931803, -24.73036655174042764, -8.660254037844380193 ) ) ;
#8415=VERTEX_POINT ( 'NONE', #9343 ) ;
#8416=ADVANCED_FACE ( 'NONE', ( #15411 ), #2435, .F. ) ;
#8417=CARTESIAN_POINT ( 'NONE',  ( -20.32861884089991023, -81.17974663899273935, 21.65063509461101532 ) ) ;
#8418=ORIENTED_EDGE ( 'NONE', *, *, #5996, .T. ) ;
#8419=ORIENTED_EDGE ( 'NONE', *, *, #7149, .F. ) ;
#8421=ORIENTED_EDGE ( 'NONE', *, *, #13028, .F. ) ;
#8422=CYLINDRICAL_SURFACE ( 'NONE', #4877, 1.500000000000001554 ) ;
#8425=DIRECTION ( 'NONE',  ( -0.1566598588826321747, 0.9876526153536343555, 0.000000000000000000 ) ) ;
#8426=CARTESIAN_POINT ( 'NONE',  ( -31.52190560670403841, -20.18723064414410828, -12.99038105676658006 ) ) ;
#8427=EDGE_CURVE ( 'NONE', #11472, #6385, #3298, .T. ) ;
#8428=AXIS2_PLACEMENT_3D ( 'NONE', #9419, #12523, #12324 ) ;
#8430=FACE_OUTER_BOUND ( 'NONE', #3753, .T. ) ;
#8431=CYLINDRICAL_SURFACE ( 'NONE', #16907, 1.500000000000001554 ) ;
#8432=AXIS2_PLACEMENT_3D ( 'NONE', #810, #11209, #6592 ) ;
#8433=AXIS2_PLACEMENT_3D ( 'NONE', #9623, #8490, #2513 ) ;
#8434=CARTESIAN_POINT ( 'NONE',  ( 2.881217619910392269, -77.49823995525089515, 12.99038105676660493 ) ) ;
#8435=DIRECTION ( 'NONE',  ( -0.9876526153536341335, -0.1566598588826327021, 0.000000000000000000 ) ) ;
#8436=CARTESIAN_POINT ( 'NONE',  ( -66.25446545484369665, -88.46443007703510375, -21.65063509461098690 ) ) ;
#8437=ORIENTED_EDGE ( 'NONE', *, *, #13564, .T. ) ;
#8439=CARTESIAN_POINT ( 'NONE',  ( -42.87991068327077926, -21.98881902129438615, 21.65063509461101887 ) ) ;
#8440=DIRECTION ( 'NONE',  ( 0.000000000000000000, 0.000000000000000000, 1.000000000000000000 ) ) ;
#8441=EDGE_LOOP ( 'NONE', ( #11840, #1120, #6191, #3114 ) ) ;
#8442=EDGE_CURVE ( 'NONE', #15648, #12551, #16561, .T. ) ;
#8444=DIRECTION ( 'NONE',  ( -0.9876526153536341335, -0.1566598588826327021, 0.000000000000000000 ) ) ;
#8445=ADVANCED_FACE ( 'NONE', ( #5761 ), #16147, .F. ) ;
#8446=CIRCLE ( 'NONE', #18778, 1.500000000000000000 ) ;
#8447=VERTEX_POINT ( 'NONE', #3139 ) ;
#8448=ORIENTED_EDGE ( 'NONE', *, *, #18655, .T. ) ;
#8449=CARTESIAN_POINT ( 'NONE',  ( -66.29410046502155751, -30.76524864068697696, 8.660254037844417496 ) ) ;
#8450=CIRCLE ( 'NONE', #4195, 1.500000000000000888 ) ;
#8451=AXIS2_PLACEMENT_3D ( 'NONE', #13288, #323, #16337 ) ;
#8452=FACE_BOUND ( 'NONE', #18668, .T. ) ;
#8453=EDGE_CURVE ( 'NONE', #5884, #14364, #8474, .T. ) ;
#8455=AXIS2_PLACEMENT_3D ( 'NONE', #9499, #15266, #6673 ) ;
#8456=VECTOR ( 'NONE', #14324, 1000.000000000000000 ) ;
#8458=AXIS2_PLACEMENT_3D ( 'NONE', #8876, #14562, #10099 ) ;
#8460=DIRECTION ( 'NONE',  ( -0.1566598588826321192, 0.9876526153536342445, 7.798540720466730171E-17 ) ) ;
#8461=AXIS2_PLACEMENT_3D ( 'NONE', #1666, #10005, #5932 ) ;
#8462=AXIS2_PLACEMENT_3D ( 'NONE', #1433, #12966, #7 ) ;
#8463=AXIS2_PLACEMENT_3D ( 'NONE', #4323, #17242, #4221 ) ;
#8464=CARTESIAN_POINT ( 'NONE',  ( -52.96079015774754595, -28.65034054577145994, 17.32050807568881723 ) ) ;
#8465=EDGE_CURVE ( 'NONE', #14662, #10352, #9973, .T. ) ;
#8466=DIRECTION ( 'NONE',  ( -0.1566598588826321747, 0.9876526153536343555, 0.000000000000000000 ) ) ;
#8467=EDGE_CURVE ( 'NONE', #1369, #12170, #14816, .T. ) ;
#8468=ORIENTED_EDGE ( 'NONE', *, *, #5749, .F. ) ;
#8469=VERTEX_POINT ( 'NONE', #11503 ) ;
#8470=AXIS2_PLACEMENT_3D ( 'NONE', #15947, #9978, #5633 ) ;
#8471=ORIENTED_EDGE ( 'NONE', *, *, #12545, .T. ) ;
#8472=CARTESIAN_POINT ( 'NONE',  ( 9.300959619709004755, -76.47995087251376845, -12.99038105676658894 ) ) ;
#8473=EDGE_CURVE ( 'NONE', #10566, #3641, #15687, .T. ) ;
#8474=CIRCLE ( 'NONE', #13906, 1.500000000000000888 ) ;
#8475=EDGE_CURVE ( 'NONE', #3563, #3927, #6665, .T. ) ;
#8476=ORIENTED_EDGE ( 'NONE', *, *, #2168, .T. ) ;
#8477=CIRCLE ( 'NONE', #8771, 1.500000000000000444 ) ;
#8478=VERTEX_POINT ( 'NONE', #1313 ) ;
#8479=CARTESIAN_POINT ( 'NONE',  ( -2.057045456857756971, -78.28153924966404986, 4.330127018922209636 ) ) ;
#8480=DIRECTION ( 'NONE',  ( -0.9876526153536336894, -0.1566598588826349503, 0.000000000000000000 ) ) ;
#8482=EDGE_LOOP ( 'NONE', ( #2980, #3115, #11059, #8013 ) ) ;
#8483=VECTOR ( 'NONE', #6786, 1000.000000000000000 ) ;
#8484=DIRECTION ( 'NONE',  ( -0.1566598588826321192, 0.9876526153536342445, 7.798540720466731404E-17 ) ) ;
#8487=DIRECTION ( 'NONE',  ( 0.000000000000000000, 0.000000000000000000, 1.000000000000000000 ) ) ;
#8489=CARTESIAN_POINT ( 'NONE',  ( -53.90880776292333820, -86.50618184100221697, 1.424741226644455312E-14 ) ) ;
#8490=DIRECTION ( 'NONE',  ( -0.1566598588826321747, 0.9876526153536343555, 0.000000000000000000 ) ) ;
#8492=ORIENTED_EDGE ( 'NONE', *, *, #5114, .T. ) ;
#8493=ORIENTED_EDGE ( 'NONE', *, *, #5812, .T. ) ;
#8494=DIRECTION ( 'NONE',  ( -0.1566598588826321192, 0.9876526153536342445, 7.798540720466731404E-17 ) ) ;
#8496=AXIS2_PLACEMENT_3D ( 'NONE', #5948, #17642, #17438 ) ;
#8499=DIRECTION ( 'NONE',  ( -0.1566598588826321192, 0.9876526153536342445, 7.798540720466731404E-17 ) ) ;
#8500=ORIENTED_EDGE ( 'NONE', *, *, #10970, .T. ) ;
#8501=AXIS2_PLACEMENT_3D ( 'NONE', #2701, #8494, #14277 ) ;
#8502=DIRECTION ( 'NONE',  ( -0.1566598588826321192, 0.9876526153536342445, 7.798540720466731404E-17 ) ) ;
#8503=EDGE_CURVE ( 'NONE', #1233, #16242, #11474, .T. ) ;
#8504=ORIENTED_EDGE ( 'NONE', *, *, #9567, .F. ) ;
#8506=EDGE_CURVE ( 'NONE', #5893, #13704, #17609, .T. ) ;
#8507=DIRECTION ( 'NONE',  ( -0.1566598588826321747, 0.9876526153536343555, 0.000000000000000000 ) ) ;
#8508=AXIS2_PLACEMENT_3D ( 'NONE', #8185, #13954, #5338 ) ;
#8509=CARTESIAN_POINT ( 'NONE',  ( -62.63296299034339398, -25.12201619894700499, -12.99038105676658006 ) ) ;
#8510=CARTESIAN_POINT ( 'NONE',  ( -7.528769851480577202, -21.44398703717040888, -12.99038105676658006 ) ) ;
#8513=EDGE_LOOP ( 'NONE', ( #11635, #2840, #2788, #15265 ) ) ;
#8514=DIRECTION ( 'NONE',  ( -0.1566598588826321192, 0.9876526153536342445, 7.798540720466730171E-17 ) ) ;
#8515=FACE_OUTER_BOUND ( 'NONE', #4572, .T. ) ;
#8517=LINE ( 'NONE', #6652, #1082 ) ;
#8518=CARTESIAN_POINT ( 'NONE',  ( -9.299721761247353058, -16.66238381928489787, 8.660254037844413944 ) ) ;
#8520=DIRECTION ( 'NONE',  ( 0.000000000000000000, 0.000000000000000000, 1.000000000000000000 ) ) ;
#8521=AXIS2_PLACEMENT_3D ( 'NONE', #17043, #10834, #13980 ) ;
#8522=CARTESIAN_POINT ( 'NONE',  ( -15.22563745336913144, -17.60234297258069347, 4.330127018922218518 ) ) ;
#8523=ORIENTED_EDGE ( 'NONE', *, *, #11659, .T. ) ;
#8525=DIRECTION ( 'NONE',  ( -0.1566598588826321192, 0.9876526153536342445, 7.798540720466730171E-17 ) ) ;
#8526=CARTESIAN_POINT ( 'NONE',  ( -46.33669483700847280, -22.53712852738359729, 21.65063509461102242 ) ) ;
#8527=VERTEX_POINT ( 'NONE', #15589 ) ;
#8528=ORIENTED_EDGE ( 'NONE', *, *, #17143, .T. ) ;
#8530=EDGE_CURVE ( 'NONE', #8287, #4436, #2812, .T. ) ;
#8531=VECTOR ( 'NONE', #15899, 1000.000000000000000 ) ;
#8533=CIRCLE ( 'NONE', #3345, 20.00000000000001066 ) ;
#8534=CARTESIAN_POINT ( 'NONE',  ( -48.02252708097940825, -27.86704125135829813, -8.660254037844380193 ) ) ;
#8536=DIRECTION ( 'NONE',  ( -0.1566598588826321192, 0.9876526153536342445, 7.798540720466731404E-17 ) ) ;
#8537=CARTESIAN_POINT ( 'NONE',  ( -69.54653129781877396, -26.21863521112544504, 21.65063509461101887 ) ) ;
#8539=EDGE_CURVE ( 'NONE', #10405, #11588, #4571, .T. ) ;
#8541=ORIENTED_EDGE ( 'NONE', *, *, #15274, .F. ) ;
#8542=DIRECTION ( 'NONE',  ( -0.9876526153536336894, -0.1566598588826349503, 0.000000000000000000 ) ) ;
#8543=FACE_BOUND ( 'NONE', #16828, .T. ) ;
#8544=EDGE_LOOP ( 'NONE', ( #15353, #6649, #6585, #5151, #17544, #4176, #10727, #953 ) ) ;
#8545=DIRECTION ( 'NONE',  ( -0.1566598588826321192, 0.9876526153536342445, 7.798540720466731404E-17 ) ) ;
#8546=ORIENTED_EDGE ( 'NONE', *, *, #2134, .F. ) ;
#8547=VECTOR ( 'NONE', #16054, 1000.000000000000000 ) ;
#8549=CYLINDRICAL_SURFACE ( 'NONE', #17568, 1.500000000000001554 ) ;
#8550=VERTEX_POINT ( 'NONE', #10348 ) ;
#8551=EDGE_LOOP ( 'NONE', ( #16604, #13987 ) ) ;
#8552=DIRECTION ( 'NONE',  ( -0.1566598588826321192, 0.9876526153536342445, 7.798540720466731404E-17 ) ) ;
#8553=CIRCLE ( 'NONE', #996, 1.500000000000001332 ) ;
#8554=CARTESIAN_POINT ( 'NONE',  ( -35.47251606811855851, -20.81387007967463632, -8.660254037844380193 ) ) ;
#8555=CIRCLE ( 'NONE', #375, 1.499999999999999556 ) ;
#8557=CIRCLE ( 'NONE', #14883, 1.500000000000001332 ) ;
#8558=ADVANCED_FACE ( 'NONE', ( #6902 ), #14372, .F. ) ;
#8560=ORIENTED_EDGE ( 'NONE', *, *, #11008, .T. ) ;
#8561=ORIENTED_EDGE ( 'NONE', *, *, #7682, .F. ) ;
#8562=AXIS2_PLACEMENT_3D ( 'NONE', #312, #3500, #13459 ) ;
#8563=FACE_OUTER_BOUND ( 'NONE', #849, .T. ) ;
#8564=DIRECTION ( 'NONE',  ( -0.1566598588826321192, 0.9876526153536342445, 7.798540720466730171E-17 ) ) ;
#8565=DIRECTION ( 'NONE',  ( -0.9876526153536336894, -0.1566598588826350336, 0.000000000000000000 ) ) ;
#8567=VERTEX_POINT ( 'NONE', #2613 ) ;
#8568=CARTESIAN_POINT ( 'NONE',  ( -70.24471092643608472, -31.39188807621751209, -21.65063509461098334 ) ) ;
#8569=EDGE_CURVE ( 'NONE', #15025, #2420, #7893, .T. ) ;
#8570=ORIENTED_EDGE ( 'NONE', *, *, #3353, .T. ) ;
#8571=ORIENTED_EDGE ( 'NONE', *, *, #3852, .T. ) ;
#8573=DIRECTION ( 'NONE',  ( -0.1566598588826321192, 0.9876526153536342445, 7.798540720466731404E-17 ) ) ;
#8576=FACE_BOUND ( 'NONE', #7652, .T. ) ;
#8577=CARTESIAN_POINT ( 'NONE',  ( -16.87183468716221313, -80.63143713290354242, 12.99038105676661203 ) ) ;
#8578=ORIENTED_EDGE ( 'NONE', *, *, #8066, .T. ) ;
#8579=CIRCLE ( 'NONE', #398, 1.500000000000000000 ) ;
#8580=CARTESIAN_POINT ( 'NONE',  ( -49.95819730150879678, -85.87954240547168183, 21.65063509461101532 ) ) ;
#8581=CARTESIAN_POINT ( 'NONE',  ( -71.72618984946653597, -31.62687786454144856, 4.330127018922217630 ) ) ;
#8582=DIRECTION ( 'NONE',  ( -0.1566598588826321192, 0.9876526153536342445, 7.798540720466730171E-17 ) ) ;
#8583=EDGE_LOOP ( 'NONE', ( #6870, #7019 ) ) ;
#8585=EDGE_CURVE ( 'NONE', #14458, #4359, #17239, .T. ) ;
#8586=DIRECTION ( 'NONE',  ( -0.1566598588826321192, 0.9876526153536342445, 7.798540720466730171E-17 ) ) ;
#8587=EDGE_CURVE ( 'NONE', #4058, #16216, #4554, .T. ) ;
#8588=CARTESIAN_POINT ( 'NONE',  ( -72.50948914387967648, -26.68861478777332152, -12.99038105676658006 ) ) ;
#8590=ORIENTED_EDGE ( 'NONE', *, *, #16052, .T. ) ;
#8593=DIRECTION ( 'NONE',  ( -0.1566598588826321192, 0.9876526153536342445, 7.798540720466730171E-17 ) ) ;
#8595=CARTESIAN_POINT ( 'NONE',  ( -76.66445292623467367, -32.41017715895461038, 21.65063509461101887 ) ) ;
#8596=VERTEX_POINT ( 'NONE', #18771 ) ;
#8597=EDGE_LOOP ( 'NONE', ( #2340, #108 ) ) ;
#8598=CARTESIAN_POINT ( 'NONE',  ( -53.74408945216070776, -23.71207746900332580, 1.908195823574487804E-14 ) ) ;
#8599=DIRECTION ( 'NONE',  ( -0.1566598588826321192, 0.9876526153536342445, 7.798540720466731404E-17 ) ) ;
#8600=CARTESIAN_POINT ( 'NONE',  ( -60.36818477289978091, -29.82528948739120267, 4.330127018922217630 ) ) ;
#8602=AXIS2_PLACEMENT_3D ( 'NONE', #5282, #3828, #8221 ) ;
#8604=DIRECTION ( 'NONE',  ( -0.1566598588826321192, 0.9876526153536342445, 7.798540720466731404E-17 ) ) ;
#8605=VERTEX_POINT ( 'NONE', #6480 ) ;
#8606=EDGE_CURVE ( 'NONE', #12283, #8278, #13277, .T. ) ;
#8607=LINE ( 'NONE', #4227, #5424 ) ;
#8608=EDGE_LOOP ( 'NONE', ( #14117, #770 ) ) ;
#8609=DIRECTION ( 'NONE',  ( -0.1566598588826321192, 0.9876526153536342445, 7.798540720466731404E-17 ) ) ;
#8610=DIRECTION ( 'NONE',  ( -0.9876526153536344665, -0.1566598588826304539, 0.000000000000000000 ) ) ;
#8611=CARTESIAN_POINT ( 'NONE',  ( -76.17062661855784711, -32.33184722951329348, 17.32050807568881723 ) ) ;
#8613=ADVANCED_FACE ( 'NONE', ( #7514 ), #3414, .F. ) ;
#8615=ORIENTED_EDGE ( 'NONE', *, *, #2282, .T. ) ;
#8616=DIRECTION ( 'NONE',  ( -0.1566598588826321192, 0.9876526153536342445, 7.798540720466730171E-17 ) ) ;
#8617=EDGE_LOOP ( 'NONE', ( #16283, #5256 ) ) ;
#8618=ORIENTED_EDGE ( 'NONE', *, *, #9241, .T. ) ;
#8620=CARTESIAN_POINT ( 'NONE',  ( -59.67000514428247016, -24.65203662229912496, 12.99038105676661736 ) ) ;
#8621=DIRECTION ( 'NONE',  ( -0.1566598588826321747, 0.9876526153536343555, 0.000000000000000000 ) ) ;
#8622=DIRECTION ( 'NONE',  ( 0.000000000000000000, 0.000000000000000000, 1.000000000000000000 ) ) ;
#8623=DIRECTION ( 'NONE',  ( -0.1566598588826321192, 0.9876526153536342445, 7.798540720466730171E-17 ) ) ;
#8627=EDGE_CURVE ( 'NONE', #8447, #11204, #4908, .T. ) ;
#8628=( NAMED_UNIT ( * ) PLANE_ANGLE_UNIT ( ) SI_UNIT ( $, .RADIAN. ) );
#8629=DIRECTION ( 'NONE',  ( -0.9876526153536341335, -0.1566598588826327021, 0.000000000000000000 ) ) ;
#8630=AXIS2_PLACEMENT_3D ( 'NONE', #4832, #17762, #487 ) ;
#8631=ORIENTED_EDGE ( 'NONE', *, *, #484, .T. ) ;
#8632=ADVANCED_FACE ( 'NONE', ( #11850 ), #500, .F. ) ;
#8633=EDGE_CURVE ( 'NONE', #18092, #16165, #12479, .T. ) ;
#8634=DIRECTION ( 'NONE',  ( -0.1566598588826321747, 0.9876526153536343555, 0.000000000000000000 ) ) ;
#8635=ORIENTED_EDGE ( 'NONE', *, *, #2540, .T. ) ;
#8636=ORIENTED_EDGE ( 'NONE', *, *, #15257, .F. ) ;
#8637=DIRECTION ( 'NONE',  ( -0.9876526153536336894, -0.1566598588826350336, 0.000000000000000000 ) ) ;
#8638=EDGE_CURVE ( 'NONE', #2916, #4611, #10436, .T. ) ;
#8640=DIRECTION ( 'NONE',  ( -0.9876526153536336894, -0.1566598588826350336, 0.000000000000000000 ) ) ;
#8641=AXIS2_PLACEMENT_3D ( 'NONE', #6327, #9237, #3358 ) ;
#8643=FACE_OUTER_BOUND ( 'NONE', #4542, .T. ) ;
#8644=VERTEX_POINT ( 'NONE', #17965 ) ;
#8645=DIRECTION ( 'NONE',  ( -0.9876526153536336894, -0.1566598588826350336, 0.000000000000000000 ) ) ;
#8646=ORIENTED_EDGE ( 'NONE', *, *, #8931, .F. ) ;
#8647=CARTESIAN_POINT ( 'NONE',  ( -38.92930022185625205, -21.36217958576383680, 1.214306433183764966E-14 ) ) ;
#8649=DIRECTION ( 'NONE',  ( -0.1566598588826321192, 0.9876526153536342445, 7.798540720466731404E-17 ) ) ;
#8652=DIRECTION ( 'NONE',  ( 0.000000000000000000, 0.000000000000000000, 1.000000000000000000 ) ) ;
#8653=EDGE_LOOP ( 'NONE', ( #838, #1117, #8476, #3776 ) ) ;
#8654=ORIENTED_EDGE ( 'NONE', *, *, #23, .T. ) ;
#8655=ORIENTED_EDGE ( 'NONE', *, *, #18581, .T. ) ;
#8656=CARTESIAN_POINT ( 'NONE',  ( -9.299721761247353058, -16.66238381928489787, 17.32050807568881368 ) ) ;
#8657=ADVANCED_FACE ( 'NONE', ( #9215 ), #9300, .F. ) ;
#8658=EDGE_LOOP ( 'NONE', ( #15874, #904 ) ) ;
#8660=CARTESIAN_POINT ( 'NONE',  ( 55.85952145814821534, 6.938893903907228378E-15, 24.99999999999998224 ) ) ;
#8661=VECTOR ( 'NONE', #14605, 1000.000000000000000 ) ;
#8662=EDGE_CURVE ( 'NONE', #2455, #9953, #4316, .T. ) ;
#8665=CARTESIAN_POINT ( 'NONE',  ( -62.83731631128386397, -30.21693913459777647, 8.660254037844417496 ) ) ;
#8668=CARTESIAN_POINT ( 'NONE',  ( -7.818242838216901802, -16.42739403096095074, 1.579620830366336657E-14 ) ) ;
#8671=ORIENTED_EDGE ( 'NONE', *, *, #9393, .T. ) ;
#8672=DIRECTION ( 'NONE',  ( -1.000000000000000000, 0.000000000000000000, 0.000000000000000000 ) ) ;
#8673=CIRCLE ( 'NONE', #15316, 1.500000000000000888 ) ;
#8674=DIRECTION ( 'NONE',  ( 0.000000000000000000, 0.000000000000000000, 1.000000000000000000 ) ) ;
#8675=VERTEX_POINT ( 'NONE', #7616 ) ;
#8676=EDGE_CURVE ( 'NONE', #17125, #9211, #10364, .T. ) ;
#8677=AXIS2_PLACEMENT_3D ( 'NONE', #16479, #11805, #12183 ) ;
#8678=VERTEX_POINT ( 'NONE', #3596 ) ;
#8680=ADVANCED_FACE ( 'NONE', ( #13379 ), #16326, .F. ) ;
#8681=ADVANCED_FACE ( 'NONE', ( #10710 ), #16511, .F. ) ;
#8682=DIRECTION ( 'NONE',  ( -0.1566598588826321192, 0.9876526153536342445, 7.798540720466730171E-17 ) ) ;
#8683=CARTESIAN_POINT ( 'NONE',  ( -81.73462711737164454, 33.01666666666666572, 35.00000000000000000 ) ) ;
#8684=CARTESIAN_POINT ( 'NONE',  ( -38.14600092744310444, -26.30044266253198160, 8.660254037844417496 ) ) ;
#8685=CIRCLE ( 'NONE', #11682, 1.500000000000000888 ) ;
#8687=CIRCLE ( 'NONE', #523, 1.500000000000001332 ) ;
#8688=DIRECTION ( 'NONE',  ( -0.1566598588826321747, 0.9876526153536343555, 0.000000000000000000 ) ) ;
#8690=ORIENTED_EDGE ( 'NONE', *, *, #10923, .F. ) ;
#8691=DIRECTION ( 'NONE',  ( -0.1566598588826321192, 0.9876526153536342445, 7.798540720466730171E-17 ) ) ;
#8692=ORIENTED_EDGE ( 'NONE', *, *, #489, .F. ) ;
#8694=DIRECTION ( 'NONE',  ( -0.9876526153536336894, -0.1566598588826349503, 0.000000000000000000 ) ) ;
#8697=EDGE_CURVE ( 'NONE', #10816, #9211, #2376, .T. ) ;
#8698=ADVANCED_FACE ( 'NONE', ( #14033 ), #18551, .F. ) ;
#8699=CIRCLE ( 'NONE', #17801, 1.500000000000001332 ) ;
#8701=AXIS2_PLACEMENT_3D ( 'NONE', #18172, #9420, #5146 ) ;
#8702=CARTESIAN_POINT ( 'NONE',  ( -19.17624791478365864, -18.22898240811121440, -17.32050807568878170 ) ) ;
#8703=EDGE_CURVE ( 'NONE', #14223, #12256, #2809, .T. ) ;
#8704=CARTESIAN_POINT ( 'NONE',  ( -74.97862068226375243, -27.08026443497989888, -17.32050807568878170 ) ) ;
#8706=CARTESIAN_POINT ( 'NONE',  ( -35.67686938905902849, -25.90879301532540779, 12.99038105676661736 ) ) ;
#8707=CARTESIAN_POINT ( 'NONE',  ( -17.85948730251583783, -80.78809699178616199, 8.660254037844412167 ) ) ;
#8709=AXIS2_PLACEMENT_3D ( 'NONE', #14817, #16518, #617 ) ;
#8710=DIRECTION ( 'NONE',  ( 0.000000000000000000, 0.000000000000000000, 1.000000000000000000 ) ) ;
#8712=CARTESIAN_POINT ( 'NONE',  ( -5.059638313096497697, -21.05233738996382797, 1.522258424776792809E-14 ) ) ;
#8713=CYLINDRICAL_SURFACE ( 'NONE', #14470, 1.500000000000000888 ) ;
#8715=ORIENTED_EDGE ( 'NONE', *, *, #3450, .T. ) ;
#8716=CIRCLE ( 'NONE', #12326, 1.500000000000001332 ) ;
#8717=ORIENTED_EDGE ( 'NONE', *, *, #7777, .T. ) ;
#8718=LINE ( 'NONE', #2562, #17559 ) ;
#8719=VERTEX_POINT ( 'NONE', #13937 ) ;
#8720=EDGE_LOOP ( 'NONE', ( #16017, #16788, #2918, #2929 ) ) ;
#8721=ORIENTED_EDGE ( 'NONE', *, *, #10407, .T. ) ;
#8725=DIRECTION ( 'NONE',  ( -0.1566598588826321192, 0.9876526153536342445, 7.798540720466731404E-17 ) ) ;
#8726=VECTOR ( 'NONE', #16416, 1000.000000000000000 ) ;
#8727=AXIS2_PLACEMENT_3D ( 'NONE', #18537, #12788, #15729 ) ;
#8729=EDGE_CURVE ( 'NONE', #3731, #5152, #991, .T. ) ;
#8730=EDGE_CURVE ( 'NONE', #6631, #13791, #15824, .T. ) ;
#8731=DIRECTION ( 'NONE',  ( 0.000000000000000000, 0.000000000000000000, 1.000000000000000000 ) ) ;
#8733=CARTESIAN_POINT ( 'NONE',  ( -40.08167114797249297, -84.31294381664535820, 12.99038105676661203 ) ) ;
#8734=CYLINDRICAL_SURFACE ( 'NONE', #12713, 1.500000000000001554 ) ;
#8735=CARTESIAN_POINT ( 'NONE',  ( -66.29410046502155751, -30.76524864068697696, -8.660254037844380193 ) ) ;
#8736=DIRECTION ( 'NONE',  ( -0.1566598588826321747, 0.9876526153536343555, 0.000000000000000000 ) ) ;
#8737=AXIS2_PLACEMENT_3D ( 'NONE', #4429, #2836, #1781 ) ;
#8741=ORIENTED_EDGE ( 'NONE', *, *, #17635, .F. ) ;
#8742=ORIENTED_EDGE ( 'NONE', *, *, #596, .F. ) ;
#8743=LINE ( 'NONE', #8472, #3348 ) ;
#8744=ORIENTED_EDGE ( 'NONE', *, *, #18077, .T. ) ;
#8745=DIRECTION ( 'NONE',  ( -0.9876526153536336894, -0.1566598588826350336, 0.000000000000000000 ) ) ;
#8747=DIRECTION ( 'NONE',  ( -1.000000000000000000, 0.000000000000000000, 0.000000000000000000 ) ) ;
#8748=AXIS2_PLACEMENT_3D ( 'NONE', #4563, #14793, #1639 ) ;
#8749=CARTESIAN_POINT ( 'NONE',  ( -75.18297400320422241, -32.17518737063066681, -4.330127018922181215 ) ) ;
#8751=CARTESIAN_POINT ( 'NONE',  ( -37.94164760650263446, -21.20551972688121367, -12.99038105676658006 ) ) ;
#8752=CARTESIAN_POINT ( 'NONE',  ( 2.881217619910392269, -77.49823995525089515, 21.65063509461100821 ) ) ;
#8753=DIRECTION ( 'NONE',  ( -0.000000000000000000, -0.000000000000000000, -1.000000000000000000 ) ) ;
#8754=DIRECTION ( 'NONE',  ( 0.000000000000000000, 0.000000000000000000, 1.000000000000000000 ) ) ;
#8755=AXIS2_PLACEMENT_3D ( 'NONE', #11478, #17314, #11203 ) ;
#8758=ORIENTED_EDGE ( 'NONE', *, *, #15969, .T. ) ;
#8759=DIRECTION ( 'NONE',  ( -0.9876526153536341335, -0.1566598588826327021, 0.000000000000000000 ) ) ;
#8760=DIRECTION ( 'NONE',  ( 0.000000000000000000, 0.000000000000000000, 1.000000000000000000 ) ) ;
#8761=EDGE_CURVE ( 'NONE', #14798, #17742, #13838, .T. ) ;
#8762=FACE_OUTER_BOUND ( 'NONE', #4690, .T. ) ;
#8763=VECTOR ( 'NONE', #2226, 1000.000000000000000 ) ;
#8764=CIRCLE ( 'NONE', #15423, 1.500000000000000888 ) ;
#8770=DIRECTION ( 'NONE',  ( -0.1566598588826321192, 0.9876526153536342445, 7.798540720466731404E-17 ) ) ;
#8771=AXIS2_PLACEMENT_3D ( 'NONE', #8938, #14716, #17881 ) ;
#8772=CARTESIAN_POINT ( 'NONE',  ( -84.16561914167408531, -33.59999999999994458, 30.00000000000000000 ) ) ;
#8774=ORIENTED_EDGE ( 'NONE', *, *, #14007, .F. ) ;
#8776=ADVANCED_FACE ( 'NONE', ( #5813 ), #5523, .F. ) ;
#8778=CIRCLE ( 'NONE', #3628, 1.499999999999999556 ) ;
#8779=CARTESIAN_POINT ( 'NONE',  ( -33.16810284049710589, -83.21632480446696434, 21.65063509461101532 ) ) ;
#8780=CARTESIAN_POINT ( 'NONE',  ( -7.818242838216901802, -16.42739403096095074, -8.660254037844380193 ) ) ;
#8784=LINE ( 'NONE', #5938, #17002 ) ;
#8785=ORIENTED_EDGE ( 'NONE', *, *, #16543, .F. ) ;
#8786=EDGE_CURVE ( 'NONE', #12053, #16372, #17566, .T. ) ;
#8787=AXIS2_PLACEMENT_3D ( 'NONE', #4336, #11520, #17533 ) ;
#8788=VECTOR ( 'NONE', #4900, 1000.000000000000000 ) ;
#8789=VERTEX_POINT ( 'NONE', #189 ) ;
#8794=CARTESIAN_POINT ( 'NONE',  ( -17.69476899175320739, -17.99399261978727083, -8.660254037844380193 ) ) ;
#8796=EDGE_CURVE ( 'NONE', #450, #3169, #1014, .T. ) ;
#8797=ORIENTED_EDGE ( 'NONE', *, *, #10923, .T. ) ;
#8798=CARTESIAN_POINT ( 'NONE',  ( -45.51376053241749986, -85.17457304049983691, -17.32050807568878525 ) ) ;
#8799=CYLINDRICAL_SURFACE ( 'NONE', #1768, 1.500000000000001554 ) ;
#8801=DIRECTION ( 'NONE',  ( -0.9876526153536341335, -0.1566598588826327021, 0.000000000000000000 ) ) ;
#8802=ORIENTED_EDGE ( 'NONE', *, *, #14862, .T. ) ;
#8803=CIRCLE ( 'NONE', #1835, 1.499999999999999556 ) ;
#8805=EDGE_CURVE ( 'NONE', #8207, #7506, #5846, .T. ) ;
#8806=EDGE_CURVE ( 'NONE', #14356, #1673, #2507, .T. ) ;
#8807=CARTESIAN_POINT ( 'NONE',  ( -6.995308533625909320, -79.06483854407721878, 4.330127018922213189 ) ) ;
#8808=DIRECTION ( 'NONE',  ( 0.1566598588826321470, -0.9876526153536342445, 5.026083453879674093E-18 ) ) ;
#8809=EDGE_CURVE ( 'NONE', #4130, #8275, #2215, .T. ) ;
#8810=VERTEX_POINT ( 'NONE', #4450 ) ;
#8811=EDGE_CURVE ( 'NONE', #10439, #14890, #15530, .T. ) ;
#8812=CIRCLE ( 'NONE', #17921, 1.500000000000000888 ) ;
#8813=VERTEX_POINT ( 'NONE', #1271 ) ;
#8814=DIRECTION ( 'NONE',  ( -0.1566598588826321747, 0.9876526153536343555, 0.000000000000000000 ) ) ;
#8815=EDGE_CURVE ( 'NONE', #7859, #4208, #9173, .T. ) ;
#8817=EDGE_CURVE ( 'NONE', #8822, #9530, #5237, .T. ) ;
#8818=ORIENTED_EDGE ( 'NONE', *, *, #13305, .F. ) ;
#8819=CIRCLE ( 'NONE', #45, 1.500000000000000000 ) ;
#8820=CARTESIAN_POINT ( 'NONE',  ( -79.30363509306917535, 32.43333333333333002, -24.99999999999999289 ) ) ;
#8821=DIRECTION ( 'NONE',  ( 0.000000000000000000, 0.000000000000000000, 1.000000000000000000 ) ) ;
#8822=VERTEX_POINT ( 'NONE', #2662 ) ;
#8823=CIRCLE ( 'NONE', #7656, 1.499999999999999556 ) ;
#8824=DIRECTION ( 'NONE',  ( -0.1566598588826321192, 0.9876526153536342445, 7.798540720466731404E-17 ) ) ;
#8825=CIRCLE ( 'NONE', #11231, 1.500000000000000888 ) ;
#8828=ORIENTED_EDGE ( 'NONE', *, *, #5760, .F. ) ;
#8829=VECTOR ( 'NONE', #14395, 1000.000000000000000 ) ;
#8830=AXIS2_PLACEMENT_3D ( 'NONE', #14441, #13104, #135 ) ;
#8831=EDGE_CURVE ( 'NONE', #16655, #7156, #3113, .T. ) ;
#8832=ORIENTED_EDGE ( 'NONE', *, *, #12362, .T. ) ;
#8833=FACE_OUTER_BOUND ( 'NONE', #11116, .T. ) ;
#8834=DIRECTION ( 'NONE',  ( -0.1566598588826321192, 0.9876526153536342445, 7.798540720466730171E-17 ) ) ;
#8836=CARTESIAN_POINT ( 'NONE',  ( -72.01566283620284992, -26.61028485833200818, -17.32050807568878170 ) ) ;
#8837=EDGE_CURVE ( 'NONE', #10533, #11499, #13392, .T. ) ;
#8838=AXIS2_PLACEMENT_3D ( 'NONE', #1985, #2178, #9475 ) ;
#8839=EDGE_LOOP ( 'NONE', ( #3417, #18407, #7087, #5630 ) ) ;
#8841=EDGE_CURVE ( 'NONE', #17674, #8596, #4921, .T. ) ;
#8843=CARTESIAN_POINT ( 'NONE',  ( -5.513829610595458064, -78.82984875575326100, 21.65063509461100821 ) ) ;
#8844=EDGE_LOOP ( 'NONE', ( #16859, #16203, #1711, #4537 ) ) ;
#8845=ORIENTED_EDGE ( 'NONE', *, *, #11598, .F. ) ;
#8846=CARTESIAN_POINT ( 'NONE',  ( -11.76885329963143079, -17.05403346649147878, 21.65063509461101532 ) ) ;
#8847=ORIENTED_EDGE ( 'NONE', *, *, #16796, .F. ) ;
#8848=CARTESIAN_POINT ( 'NONE',  ( -66.08974714408108753, -25.67032570503622679, 12.99038105676661736 ) ) ;
#8850=CARTESIAN_POINT ( 'NONE',  ( -58.68235252892886678, -24.49537676341648407, 1.908195823574487804E-14 ) ) ;
#8851=EDGE_LOOP ( 'NONE', ( #4513, #706 ) ) ;
#8852=ORIENTED_EDGE ( 'NONE', *, *, #12246, .T. ) ;
#8853=AXIS2_PLACEMENT_3D ( 'NONE', #14183, #2333, #8125 ) ;
#8854=ORIENTED_EDGE ( 'NONE', *, *, #9492, .T. ) ;
#8855=CARTESIAN_POINT ( 'NONE',  ( -49.95819730150881099, -85.87954240547168183, 4.330127018922213189 ) ) ;
#8856=DIRECTION ( 'NONE',  ( 0.000000000000000000, 0.000000000000000000, 1.000000000000000000 ) ) ;
#8857=DIRECTION ( 'NONE',  ( -0.1566598588826321747, 0.9876526153536343555, 0.000000000000000000 ) ) ;
#8858=CARTESIAN_POINT ( 'NONE',  ( -84.16561914167411373, 33.60000000000000142, 30.00000000000000000 ) ) ;
#8860=EDGE_LOOP ( 'NONE', ( #10110, #6598, #16429, #4060 ) ) ;
#8861=ORIENTED_EDGE ( 'NONE', *, *, #10748, .F. ) ;
#8862=DIRECTION ( 'NONE',  ( -0.1566598588826321192, 0.9876526153536342445, 7.798540720466730171E-17 ) ) ;
#8863=CARTESIAN_POINT ( 'NONE',  ( -59.67000514428248437, -24.65203662229912140, 4.330127018922218518 ) ) ;
#8865=DIRECTION ( 'NONE',  ( -0.1566598588826321747, 0.9876526153536343555, 0.000000000000000000 ) ) ;
#8868=DIRECTION ( 'NONE',  ( -0.1566598588826321192, 0.9876526153536342445, 7.798540720466731404E-17 ) ) ;
#8869=DIRECTION ( 'NONE',  ( -0.1566598588826321192, 0.9876526153536342445, 7.798540720466730171E-17 ) ) ;
#8871=LINE ( 'NONE', #10368, #5793 ) ;
#8872=DIRECTION ( 'NONE',  ( 0.000000000000000000, 0.000000000000000000, 1.000000000000000000 ) ) ;
#8875=AXIS2_PLACEMENT_3D ( 'NONE', #9098, #8994, #674 ) ;
#8876=CARTESIAN_POINT ( 'NONE',  ( -3.578159390066044665, -20.81734760163988440, 8.660254037844412167 ) ) ;
#8878=DIRECTION ( 'NONE',  ( -0.9876526153536336894, -0.1566598588826349503, 0.000000000000000000 ) ) ;
#8879=DIRECTION ( 'NONE',  ( -0.1566598588826321192, 0.9876526153536342445, 7.798540720466730171E-17 ) ) ;
#8881=ORIENTED_EDGE ( 'NONE', *, *, #945, .T. ) ;
#8883=ORIENTED_EDGE ( 'NONE', *, *, #14862, .F. ) ;
#8884=CYLINDRICAL_SURFACE ( 'NONE', #3922, 1.500000000000001554 ) ;
#8885=VERTEX_POINT ( 'NONE', #4820 ) ;
#8886=AXIS2_PLACEMENT_3D ( 'NONE', #14756, #2053, #4793 ) ;
#8887=EDGE_CURVE ( 'NONE', #15855, #9188, #7088, .T. ) ;
#8888=CARTESIAN_POINT ( 'NONE',  ( -40.08167114797252140, -84.31294381664535820, -12.99038105676658539 ) ) ;
#8889=DIRECTION ( 'NONE',  ( -1.000000000000000000, 0.000000000000000000, 0.000000000000000000 ) ) ;
#8890=FACE_OUTER_BOUND ( 'NONE', #15837, .T. ) ;
#8891=DIRECTION ( 'NONE',  ( -0.1566598588826321192, 0.9876526153536342445, 7.798540720466731404E-17 ) ) ;
#8892=DIRECTION ( 'NONE',  ( -0.1566598588826321192, 0.9876526153536342445, 7.798540720466730171E-17 ) ) ;
#8893=DIRECTION ( 'NONE',  ( -0.9876526153536336894, -0.1566598588826349503, 0.000000000000000000 ) ) ;
#8894=ADVANCED_FACE ( 'NONE', ( #14873 ), #392, .F. ) ;
#8895=CARTESIAN_POINT ( 'NONE',  ( -4.565812005419673802, -20.97400746052251108, 4.330127018922214077 ) ) ;
#8896=DIRECTION ( 'NONE',  ( -0.9876526153536344665, -0.1566598588826304539, 0.000000000000000000 ) ) ;
#8897=FACE_BOUND ( 'NONE', #13098, .T. ) ;
#8898=DIRECTION ( 'NONE',  ( -0.9876526153536341335, -0.1566598588826327021, 0.000000000000000000 ) ) ;
#8900=VERTEX_POINT ( 'NONE', #16129 ) ;
#8901=VERTEX_POINT ( 'NONE', #7685 ) ;
#8904=ORIENTED_EDGE ( 'NONE', *, *, #17436, .F. ) ;
#8905=DIRECTION ( 'NONE',  ( -0.1566598588826321192, 0.9876526153536342445, 7.798540720466731404E-17 ) ) ;
#8906=DIRECTION ( 'NONE',  ( -0.9876526153536341335, -0.1566598588826327021, 0.000000000000000000 ) ) ;
#8907=VERTEX_POINT ( 'NONE', #1981 ) ;
#8908=EDGE_CURVE ( 'NONE', #16999, #1829, #12805, .T. ) ;
#8909=EDGE_CURVE ( 'NONE', #10566, #1820, #1320, .T. ) ;
#8910=CARTESIAN_POINT ( 'NONE',  ( 11.77009115809307715, -76.08830122530719109, 9.226938858386234556E-15 ) ) ;
#8911=EDGE_CURVE ( 'NONE', #8822, #16032, #12196, .T. ) ;
#8914=AXIS2_PLACEMENT_3D ( 'NONE', #11876, #6137, #17628 ) ;
#8915=EDGE_LOOP ( 'NONE', ( #2321, #2538 ) ) ;
#8916=DIRECTION ( 'NONE',  ( 1.000000000000000000, 0.000000000000000000, 0.000000000000000000 ) ) ;
#8917=ORIENTED_EDGE ( 'NONE', *, *, #15843, .T. ) ;
#8918=DIRECTION ( 'NONE',  ( -0.1566598588826321747, 0.9876526153536343555, 0.000000000000000000 ) ) ;
#8919=CARTESIAN_POINT ( 'NONE',  ( -46.54104815794897121, -27.63205146303434390, -17.32050807568878170 ) ) ;
#8921=ORIENTED_EDGE ( 'NONE', *, *, #11384, .F. ) ;
#8922=ORIENTED_EDGE ( 'NONE', *, *, #5614, .F. ) ;
#8923=ORIENTED_EDGE ( 'NONE', *, *, #270, .F. ) ;
#8924=DIRECTION ( 'NONE',  ( -0.1566598588826321747, 0.9876526153536343555, 0.000000000000000000 ) ) ;
#8925=EDGE_LOOP ( 'NONE', ( #6216, #3576, #1176, #586 ) ) ;
#8926=AXIS2_PLACEMENT_3D ( 'NONE', #11685, #14654, #8610 ) ;
#8927=FACE_BOUND ( 'NONE', #14248, .T. ) ;
#8928=EDGE_CURVE ( 'NONE', #7859, #11927, #7766, .T. ) ;
#8929=ORIENTED_EDGE ( 'NONE', *, *, #572, .F. ) ;
#8930=CARTESIAN_POINT ( 'NONE',  ( 2.058283315319403783, -14.86079544213463066, -8.660254037844383745 ) ) ;
#8931=EDGE_CURVE ( 'NONE', #5315, #6912, #17072, .T. ) ;
#8934=FACE_BOUND ( 'NONE', #15571, .T. ) ;
#8935=EDGE_CURVE ( 'NONE', #5645, #3917, #3387, .T. ) ;
#8936=CARTESIAN_POINT ( 'NONE',  ( -15.39035576413176187, -80.39644734457957043, -21.65063509461098690 ) ) ;
#8937=AXIS2_PLACEMENT_3D ( 'NONE', #16623, #422, #509 ) ;
#8938=CARTESIAN_POINT ( 'NONE',  ( -31.52190560670403841, -20.18723064414411539, 4.330127018922218518 ) ) ;
#8940=DIRECTION ( 'NONE',  ( -0.9876526153536341335, -0.1566598588826327021, 0.000000000000000000 ) ) ;
#8942=ORIENTED_EDGE ( 'NONE', *, *, #13395, .T. ) ;
#8943=FACE_BOUND ( 'NONE', #2997, .T. ) ;
#8945=DIRECTION ( 'NONE',  ( -0.1566598588826321192, 0.9876526153536342445, 7.798540720466731404E-17 ) ) ;
#8946=ORIENTED_EDGE ( 'NONE', *, *, #16346, .F. ) ;
#8947=CARTESIAN_POINT ( 'NONE',  ( -26.58364252993588650, -19.40393134973095002, -21.65063509461097979 ) ) ;
#8948=ORIENTED_EDGE ( 'NONE', *, *, #5639, .F. ) ;
#8951=DIRECTION ( 'NONE',  ( -0.9876526153536336894, -0.1566598588826349503, 0.000000000000000000 ) ) ;
#8953=EDGE_CURVE ( 'NONE', #299, #14468, #18621, .T. ) ;
#8954=CARTESIAN_POINT ( 'NONE',  ( -18.39294862037050393, -23.16724548487935564, 8.660254037844417496 ) ) ;
#8956=DIRECTION ( 'NONE',  ( -0.1566598588826321192, 0.9876526153536342445, 7.798540720466730171E-17 ) ) ;
#8957=ORIENTED_EDGE ( 'NONE', *, *, #12842, .F. ) ;
#8959=EDGE_CURVE ( 'NONE', #1993, #14599, #14916, .T. ) ;
#8960=CIRCLE ( 'NONE', #806, 1.500000000000000888 ) ;
#8961=ORIENTED_EDGE ( 'NONE', *, *, #4092, .T. ) ;
#8962=ORIENTED_EDGE ( 'NONE', *, *, #7331, .T. ) ;
#8963=AXIS2_PLACEMENT_3D ( 'NONE', #7135, #11361, #1439 ) ;
#8965=EDGE_LOOP ( 'NONE', ( #8828, #13645, #16545, #2460 ) ) ;
#8967=CARTESIAN_POINT ( 'NONE',  ( -38.14600092744310444, -26.30044266253198160, 17.32050807568881723 ) ) ;
#8968=AXIS2_PLACEMENT_3D ( 'NONE', #14089, #1133, #12651 ) ;
#8969=LINE ( 'NONE', #15903, #17031 ) ;
#8970=DIRECTION ( 'NONE',  ( -0.9876526153536341335, -0.1566598588826327021, 0.000000000000000000 ) ) ;
#8971=EDGE_CURVE ( 'NONE', #898, #7429, #15215, .T. ) ;
#8972=DIRECTION ( 'NONE',  ( -0.1566598588826321192, 0.9876526153536342445, 7.798540720466730171E-17 ) ) ;
#8973=EDGE_LOOP ( 'NONE', ( #9559, #7164 ) ) ;
#8974=CARTESIAN_POINT ( 'NONE',  ( -59.38053215754615621, -29.66862962850855823, 8.660254037844417496 ) ) ;
#8975=VECTOR ( 'NONE', #2048, 1000.000000000000000 ) ;
#8977=DIRECTION ( 'NONE',  ( -0.9876526153536341335, -0.1566598588826327576, 0.000000000000000000 ) ) ;
#8978=DIRECTION ( 'NONE',  ( 0.000000000000000000, 0.000000000000000000, 1.000000000000000000 ) ) ;
#8980=CARTESIAN_POINT ( 'NONE',  ( -48.02252708097939404, -27.86704125135830523, 17.32050807568881723 ) ) ;
#8981=ORIENTED_EDGE ( 'NONE', *, *, #7635, .T. ) ;
#8982=ORIENTED_EDGE ( 'NONE', *, *, #8453, .F. ) ;
#8983=CYLINDRICAL_SURFACE ( 'NONE', #14740, 1.500000000000001554 ) ;
#8986=VERTEX_POINT ( 'NONE', #15056 ) ;
#8987=ADVANCED_FACE ( 'NONE', ( #7493 ), #1708, .F. ) ;
#8988=CIRCLE ( 'NONE', #4736, 1.500000000000000888 ) ;
#8989=EDGE_LOOP ( 'NONE', ( #17085, #14663, #7630, #18618 ) ) ;
#8990=DIRECTION ( 'NONE',  ( -0.1566598588826321192, 0.9876526153536342445, 7.798540720466730171E-17 ) ) ;
#8994=DIRECTION ( 'NONE',  ( -0.1566598588826321747, 0.9876526153536343555, 0.000000000000000000 ) ) ;
#8998=ADVANCED_FACE ( 'NONE', ( #17670 ), #4639, .F. ) ;
#9000=CARTESIAN_POINT ( 'NONE',  ( -30.73860631229088725, -25.12549372091224598, 12.99038105676661736 ) ) ;
#9002=CIRCLE ( 'NONE', #3241, 1.499999999999999556 ) ;
#9004=EDGE_LOOP ( 'NONE', ( #18214, #3807, #1697, #11052 ) ) ;
#9005=EDGE_CURVE ( 'NONE', #10290, #18222, #1620, .T. ) ;
#9007=CARTESIAN_POINT ( 'NONE',  ( -26.74836084069850983, -82.19803572172985184, -12.99038105676658539 ) ) ;
#9008=AXIS2_PLACEMENT_3D ( 'NONE', #7218, #10397, #12962 ) ;
#9009=EDGE_LOOP ( 'NONE', ( #2717, #12509 ) ) ;
#9010=EDGE_LOOP ( 'NONE', ( #13450, #8671, #12348, #15986 ) ) ;
#9011=EDGE_CURVE ( 'NONE', #12973, #6731, #5100, .T. ) ;
#9014=DIRECTION ( 'NONE',  ( -0.9876526153536336894, -0.1566598588826349503, 0.000000000000000000 ) ) ;
#9015=CIRCLE ( 'NONE', #10569, 1.500000000000000444 ) ;
#9016=EDGE_LOOP ( 'NONE', ( #12204, #11639, #14702, #2116 ) ) ;
#9017=FACE_BOUND ( 'NONE', #9443, .T. ) ;
#9018=AXIS2_PLACEMENT_3D ( 'NONE', #583, #1809, #7598 ) ;
#9019=ORIENTED_EDGE ( 'NONE', *, *, #2037, .T. ) ;
#9020=DIRECTION ( 'NONE',  ( -0.9876526153536336894, -0.1566598588826350336, 0.000000000000000000 ) ) ;
#9021=EDGE_LOOP ( 'NONE', ( #11958, #1038 ) ) ;
#9022=EDGE_LOOP ( 'NONE', ( #12260, #13854, #16773, #13366 ) ) ;
#9023=EDGE_CURVE ( 'NONE', #8348, #18596, #6153, .T. ) ;
#9024=AXIS2_PLACEMENT_3D ( 'NONE', #4311, #17227, #15788 ) ;
#9025=ORIENTED_EDGE ( 'NONE', *, *, #5488, .T. ) ;
#9026=VECTOR ( 'NONE', #15492, 1000.000000000000000 ) ;
#9027=LINE ( 'NONE', #14997, #310 ) ;
#9028=AXIS2_PLACEMENT_3D ( 'NONE', #14164, #17123, #15669 ) ;
#9029=CARTESIAN_POINT ( 'NONE',  ( -27.28182215855319015, -24.57718421482303484, 12.99038105676661736 ) ) ;
#9030=EDGE_CURVE ( 'NONE', #13292, #2965, #2517, .T. ) ;
#9031=DIRECTION ( 'NONE',  ( -0.9876526153536336894, -0.1566598588826349503, 0.000000000000000000 ) ) ;
#9032=CARTESIAN_POINT ( 'NONE',  ( -55.39028668595378946, -86.74117162932616054, 8.660254037844412167 ) ) ;
#9033=EDGE_CURVE ( 'NONE', #10329, #5781, #16758, .T. ) ;
#9034=CARTESIAN_POINT ( 'NONE',  ( -31.72625892764450839, -25.28215357979487266, 17.32050807568881723 ) ) ;
#9035=ORIENTED_EDGE ( 'NONE', *, *, #6582, .T. ) ;
#9037=CARTESIAN_POINT ( 'NONE',  ( -20.86208015875458344, -23.55889513208593655, 4.330127018922217630 ) ) ;
#9038=EDGE_CURVE ( 'NONE', #7926, #7658, #16885, .T. ) ;
#9039=ADVANCED_FACE ( 'NONE', ( #18336 ), #5304, .F. ) ;
#9040=CARTESIAN_POINT ( 'NONE',  ( -50.28730529842300001, -23.16376796291412177, 17.32050807568881723 ) ) ;
#9041=AXIS2_PLACEMENT_3D ( 'NONE', #12806, #17463, #4069 ) ;
#9042=AXIS2_PLACEMENT_3D ( 'NONE', #6092, #17473, #13172 ) ;
#9043=EDGE_LOOP ( 'NONE', ( #2857, #4442, #15314, #12970 ) ) ;
#9044=CARTESIAN_POINT ( 'NONE',  ( -24.27922930231443743, -81.80638607452327449, 17.32050807568881368 ) ) ;
#9045=AXIS2_PLACEMENT_3D ( 'NONE', #15538, #1158, #15723 ) ;
#9046=AXIS2_PLACEMENT_3D ( 'NONE', #4981, #15233, #10758 ) ;
#9047=CARTESIAN_POINT ( 'NONE',  ( -19.38060123572412863, -23.32390534376198232, -12.99038105676658006 ) ) ;
#9048=DIRECTION ( 'NONE',  ( -0.1566598588826321192, 0.9876526153536342445, 7.798540720466731404E-17 ) ) ;
#9051=CIRCLE ( 'NONE', #8470, 1.500000000000000888 ) ;
#9052=DIRECTION ( 'NONE',  ( -0.9876526153536341335, -0.1566598588826327576, 0.000000000000000000 ) ) ;
#9053=AXIS2_PLACEMENT_3D ( 'NONE', #9858, #3112, #1530 ) ;
#9056=EDGE_CURVE ( 'NONE', #2319, #5366, #1907, .T. ) ;
#9057=ORIENTED_EDGE ( 'NONE', *, *, #807, .F. ) ;
#9059=DIRECTION ( 'NONE',  ( -0.1566598588826321747, 0.9876526153536343555, 0.000000000000000000 ) ) ;
#9060=VECTOR ( 'NONE', #5581, 1000.000000000000000 ) ;
#9061=AXIS2_PLACEMENT_3D ( 'NONE', #2128, #13677, #4872 ) ;
#9062=EDGE_LOOP ( 'NONE', ( #8421, #16531 ) ) ;
#9063=DIRECTION ( 'NONE',  ( 0.9876526153536342445, 0.1566598588826321192, -2.851797552515346363E-16 ) ) ;
#9064=ORIENTED_EDGE ( 'NONE', *, *, #18134, .F. ) ;
#9065=ORIENTED_EDGE ( 'NONE', *, *, #2240, .T. ) ;
#9066=EDGE_CURVE ( 'NONE', #2189, #3917, #8579, .T. ) ;
#9067=ORIENTED_EDGE ( 'NONE', *, *, #14539, .F. ) ;
#9068=CIRCLE ( 'NONE', #9697, 1.500000000000000888 ) ;
#9069=DIRECTION ( 'NONE',  ( -0.1566598588826321192, 0.9876526153536342445, 7.798540720466730171E-17 ) ) ;
#9071=CIRCLE ( 'NONE', #15119, 1.500000000000000444 ) ;
#9072=DIRECTION ( 'NONE',  ( -0.1566598588826321192, 0.9876526153536342445, 7.798540720466730171E-17 ) ) ;
#9075=LINE ( 'NONE', #14758, #11546 ) ;
#9077=DIRECTION ( 'NONE',  ( -0.1566598588826321747, 0.9876526153536343555, 0.000000000000000000 ) ) ;
#9078=DIRECTION ( 'NONE',  ( 0.000000000000000000, 0.000000000000000000, 1.000000000000000000 ) ) ;
#9079=AXIS2_PLACEMENT_3D ( 'NONE', #6439, #15030, #5070 ) ;
#9080=FACE_OUTER_BOUND ( 'NONE', #8844, .T. ) ;
#9081=VECTOR ( 'NONE', #12991, 1000.000000000000000 ) ;
#9082=DIRECTION ( 'NONE',  ( -0.000000000000000000, -0.000000000000000000, -1.000000000000000000 ) ) ;
#9083=ORIENTED_EDGE ( 'NONE', *, *, #8427, .T. ) ;
#9084=VECTOR ( 'NONE', #320, 1000.000000000000000 ) ;
#9085=ORIENTED_EDGE ( 'NONE', *, *, #9203, .F. ) ;
#9086=DIRECTION ( 'NONE',  ( 0.000000000000000000, 0.000000000000000000, 1.000000000000000000 ) ) ;
#9088=VERTEX_POINT ( 'NONE', #2175 ) ;
#9089=EDGE_CURVE ( 'NONE', #7880, #2300, #4010, .T. ) ;
#9090=EDGE_LOOP ( 'NONE', ( #8120, #5666 ) ) ;
#9092=ADVANCED_FACE ( 'NONE', ( #12288 ), #2352, .F. ) ;
#9093=ORIENTED_EDGE ( 'NONE', *, *, #3482, .F. ) ;
#9095=ORIENTED_EDGE ( 'NONE', *, *, #17417, .T. ) ;
#9096=CIRCLE ( 'NONE', #643, 20.00000000000001066 ) ;
#9097=EDGE_CURVE ( 'NONE', #13575, #18385, #11577, .T. ) ;
#9098=CARTESIAN_POINT ( 'NONE',  ( -23.33121169713865584, -23.95054477929251036, 17.32050807568881723 ) ) ;
#9099=AXIS2_PLACEMENT_3D ( 'NONE', #6428, #18002, #1953 ) ;
#9100=CARTESIAN_POINT ( 'NONE',  ( -63.62061560569701157, -25.27867605782963878, -8.660254037844380193 ) ) ;
#9102=AXIS2_PLACEMENT_3D ( 'NONE', #1491, #7184, #17514 ) ;
#9103=CARTESIAN_POINT ( 'NONE',  ( -62.30385499342917655, -87.83779064150456861, 1.443110928631665584E-14 ) ) ;
#9104=DIRECTION ( 'NONE',  ( 0.000000000000000000, 0.000000000000000000, 1.000000000000000000 ) ) ;
#9106=FACE_BOUND ( 'NONE', #8164, .T. ) ;
#9107=CIRCLE ( 'NONE', #961, 1.500000000000000888 ) ;
#9108=CARTESIAN_POINT ( 'NONE',  ( -39.91695283720987675, -21.51883944464648835, 4.330127018922218518 ) ) ;
#9109=VERTEX_POINT ( 'NONE', #3672 ) ;
#9110=DIRECTION ( 'NONE',  ( -0.9876526153536341335, -0.1566598588826327021, 0.000000000000000000 ) ) ;
#9111=VECTOR ( 'NONE', #10073, 1000.000000000000000 ) ;
#9112=LINE ( 'NONE', #14980, #9945 ) ;
#9113=EDGE_LOOP ( 'NONE', ( #10847, #17255 ) ) ;
#9114=CIRCLE ( 'NONE', #337, 1.500000000000000888 ) ;
#9116=EDGE_LOOP ( 'NONE', ( #8852, #5207 ) ) ;
#9118=ORIENTED_EDGE ( 'NONE', *, *, #8971, .F. ) ;
#9119=DIRECTION ( 'NONE',  ( -0.9876526153536336894, -0.1566598588826349503, 0.000000000000000000 ) ) ;
#9120=VECTOR ( 'NONE', #15565, 1000.000000000000000 ) ;
#9121=VERTEX_POINT ( 'NONE', #5398 ) ;
#9122=FACE_BOUND ( 'NONE', #705, .T. ) ;
#9124=EDGE_CURVE ( 'NONE', #6916, #17944, #13103, .T. ) ;
#9126=ORIENTED_EDGE ( 'NONE', *, *, #14049, .F. ) ;
#9127=CIRCLE ( 'NONE', #10920, 1.500000000000001332 ) ;
#9128=AXIS2_PLACEMENT_3D ( 'NONE', #5422, #12314, #3781 ) ;
#9131=EDGE_CURVE ( 'NONE', #14764, #7636, #3714, .T. ) ;
#9132=CIRCLE ( 'NONE', #6108, 1.499999999999999556 ) ;
#9133=CARTESIAN_POINT ( 'NONE',  ( 6.338001773648100468, -76.94993044916168401, -12.99038105676658894 ) ) ;
#9134=ADVANCED_FACE ( 'NONE', ( #15243 ), #13914, .F. ) ;
#9135=DIRECTION ( 'NONE',  ( -0.1566598588826321747, 0.9876526153536343555, 0.000000000000000000 ) ) ;
#9138=CARTESIAN_POINT ( 'NONE',  ( -52.42732883989288695, -86.27119205267825919, 8.660254037844412167 ) ) ;
#9139=CARTESIAN_POINT ( 'NONE',  ( -13.41505053342451426, -80.08312762681433128, 21.65063509461100821 ) ) ;
#9140=ORIENTED_EDGE ( 'NONE', *, *, #4314, .T. ) ;
#9142=CARTESIAN_POINT ( 'NONE',  ( -36.66452200441265319, -26.06545287420802737, 8.660254037844417496 ) ) ;
#9144=DIRECTION ( 'NONE',  ( -0.9876526153536336894, -0.1566598588826349503, 0.000000000000000000 ) ) ;
#9145=VECTOR ( 'NONE', #11752, 1000.000000000000000 ) ;
#9146=VERTEX_POINT ( 'NONE', #8337 ) ;
#9147=ORIENTED_EDGE ( 'NONE', *, *, #9539, .T. ) ;
#9148=VERTEX_POINT ( 'NONE', #966 ) ;
#9149=DIRECTION ( 'NONE',  ( -0.1566598588826321192, 0.9876526153536342445, 7.798540720466730171E-17 ) ) ;
#9150=VECTOR ( 'NONE', #3550, 1000.000000000000000 ) ;
#9151=FACE_BOUND ( 'NONE', #6352, .T. ) ;
#9152=EDGE_CURVE ( 'NONE', #4488, #7880, #3954, .T. ) ;
#9153=EDGE_CURVE ( 'NONE', #15836, #14096, #1631, .T. ) ;
#9154=CARTESIAN_POINT ( 'NONE',  ( -13.45468554360235203, -22.38394619046619383, -17.32050807568878170 ) ) ;
#9155=LINE ( 'NONE', #14926, #9352 ) ;
#9157=ORIENTED_EDGE ( 'NONE', *, *, #8271, .T. ) ;
#9159=DIRECTION ( 'NONE',  ( -0.1566598588826321192, 0.9876526153536342445, 7.798540720466731404E-17 ) ) ;
#9160=CYLINDRICAL_SURFACE ( 'NONE', #11083, 1.500000000000001554 ) ;
#9161=CARTESIAN_POINT ( 'NONE',  ( -51.43967622453926936, -86.11453219379563961, 4.330127018922213189 ) ) ;
#9162=VERTEX_POINT ( 'NONE', #7304 ) ;
#9163=ORIENTED_EDGE ( 'NONE', *, *, #4777, .F. ) ;
#9164=AXIS2_PLACEMENT_3D ( 'NONE', #11634, #2848, #8640 ) ;
#9165=DIRECTION ( 'NONE',  ( -0.9876526153536336894, -0.1566598588826350336, 0.000000000000000000 ) ) ;
#9166=AXIS2_PLACEMENT_3D ( 'NONE', #15853, #14431, #13000 ) ;
#9171=ADVANCED_FACE ( 'NONE', ( #10115 ), #4344, .F. ) ;
#9172=CARTESIAN_POINT ( 'NONE',  ( -68.72359699322777260, -88.85607972424169532, 8.660254037844412167 ) ) ;
#9173=CIRCLE ( 'NONE', #11279, 1.500000000000000888 ) ;
#9174=CARTESIAN_POINT ( 'NONE',  ( -14.40270314877813895, -80.23978748569695085, 8.660254037844412167 ) ) ;
#9175=DIRECTION ( 'NONE',  ( -0.1566598588826321747, 0.9876526153536343555, 0.000000000000000000 ) ) ;
#9176=CARTESIAN_POINT ( 'NONE',  ( -8.516422466834198346, -21.60064689605303911, 17.32050807568881012 ) ) ;
#9179=DIRECTION ( 'NONE',  ( -0.1566598588826321192, 0.9876526153536342445, 7.798540720466730171E-17 ) ) ;
#9180=ORIENTED_EDGE ( 'NONE', *, *, #1740, .T. ) ;
#9181=CARTESIAN_POINT ( 'NONE',  ( -29.25712738926043244, -24.89050393258829175, 21.65063509461101887 ) ) ;
#9182=CARTESIAN_POINT ( 'NONE',  ( -23.29157668696081629, -81.64972621564062649, -21.65063509461098690 ) ) ;
#9184=VERTEX_POINT ( 'NONE', #4046 ) ;
#9186=AXIS2_PLACEMENT_3D ( 'NONE', #8426, #5592, #14206 ) ;
#9187=DIRECTION ( 'NONE',  ( -0.1566598588826321192, 0.9876526153536342445, 7.798540720466730171E-17 ) ) ;
#9188=VERTEX_POINT ( 'NONE', #7388 ) ;
#9189=ORIENTED_EDGE ( 'NONE', *, *, #14593, .F. ) ;
#9190=DIRECTION ( 'NONE',  ( -0.1566598588826321192, 0.9876526153536342445, 7.798540720466730171E-17 ) ) ;
#9192=CARTESIAN_POINT ( 'NONE',  ( -0.1213752363283457369, -20.26903809555066616, -17.32050807568878170 ) ) ;
#9193=VERTEX_POINT ( 'NONE', #11431 ) ;
#9194=CARTESIAN_POINT ( 'NONE',  ( 0.4120860815263194254, -77.88988960245745830, -17.32050807568878525 ) ) ;
#9195=DIRECTION ( 'NONE',  ( -0.1566598588826321747, 0.9876526153536343555, 0.000000000000000000 ) ) ;
#9196=DIRECTION ( 'NONE',  ( -0.1566598588826321192, 0.9876526153536342445, 7.798540720466731404E-17 ) ) ;
#9197=CARTESIAN_POINT ( 'NONE',  ( -38.92930022185625205, -21.36217958576385811, 17.32050807568882078 ) ) ;
#9198=CARTESIAN_POINT ( 'NONE',  ( -47.98289207080156160, -85.56622268770642847, 4.330127018922213189 ) ) ;
#9200=CARTESIAN_POINT ( 'NONE',  ( -14.40270314877813895, -80.23978748569693664, -17.32050807568878525 ) ) ;
#9201=VERTEX_POINT ( 'NONE', #1423 ) ;
#9202=EDGE_CURVE ( 'NONE', #6188, #10331, #11616, .T. ) ;
#9203=EDGE_CURVE ( 'NONE', #2224, #7658, #18310, .T. ) ;
#9205=EDGE_LOOP ( 'NONE', ( #16180, #17720, #17148, #763 ) ) ;
#9207=DIRECTION ( 'NONE',  ( -0.1566598588826321192, 0.9876526153536342445, 7.798540720466730171E-17 ) ) ;
#9208=EDGE_CURVE ( 'NONE', #8349, #10706, #3124, .T. ) ;
#9209=ORIENTED_EDGE ( 'NONE', *, *, #4393, .T. ) ;
#9210=VERTEX_POINT ( 'NONE', #2905 ) ;
#9211=VERTEX_POINT ( 'NONE', #8704 ) ;
#9212=CARTESIAN_POINT ( 'NONE',  ( -31.68662391746665463, -82.98133501614299234, -4.330127018922185655 ) ) ;
#9213=EDGE_LOOP ( 'NONE', ( #665, #15147, #15100, #10859 ) ) ;
#9214=FACE_BOUND ( 'NONE', #17041, .T. ) ;
#9215=FACE_OUTER_BOUND ( 'NONE', #15630, .T. ) ;
#9216=ORIENTED_EDGE ( 'NONE', *, *, #14755, .F. ) ;
#9218=DIRECTION ( 'NONE',  ( -0.1566598588826321747, 0.9876526153536343555, 0.000000000000000000 ) ) ;
#9219=CARTESIAN_POINT ( 'NONE',  ( -26.74836084069850983, -82.19803572172985184, -4.330127018922185655 ) ) ;
#9221=VERTEX_POINT ( 'NONE', #5685 ) ;
#9222=ORIENTED_EDGE ( 'NONE', *, *, #13123, .F. ) ;
#9225=AXIS2_PLACEMENT_3D ( 'NONE', #13367, #11916, #7780 ) ;
#9226=DIRECTION ( 'NONE',  ( -0.1566598588826321192, 0.9876526153536342445, 7.798540720466731404E-17 ) ) ;
#9227=ORIENTED_EDGE ( 'NONE', *, *, #13764, .T. ) ;
#9228=DIRECTION ( 'NONE',  ( -0.1566598588826321192, 0.9876526153536342445, 7.798540720466730171E-17 ) ) ;
#9229=EDGE_CURVE ( 'NONE', #17343, #6767, #17440, .T. ) ;
#9230=ORIENTED_EDGE ( 'NONE', *, *, #4906, .T. ) ;
#9233=DIRECTION ( 'NONE',  ( -0.1566598588826321192, 0.9876526153536342445, 7.798540720466731404E-17 ) ) ;
#9234=EDGE_LOOP ( 'NONE', ( #9528, #13158, #11750, #5536 ) ) ;
#9235=CARTESIAN_POINT ( 'NONE',  ( -36.66452200441266029, -26.06545287420802737, -17.32050807568878170 ) ) ;
#9237=DIRECTION ( 'NONE',  ( -0.1566598588826321192, 0.9876526153536342445, 7.798540720466730171E-17 ) ) ;
#9238=EDGE_LOOP ( 'NONE', ( #16145, #9661 ) ) ;
#9239=VERTEX_POINT ( 'NONE', #12951 ) ;
#9240=DIRECTION ( 'NONE',  ( -0.1566598588826321192, 0.9876526153536342445, 7.798540720466730171E-17 ) ) ;
#9241=EDGE_CURVE ( 'NONE', #3908, #12253, #5500, .T. ) ;
#9243=ORIENTED_EDGE ( 'NONE', *, *, #14100, .F. ) ;
#9245=EDGE_LOOP ( 'NONE', ( #16704, #13961, #15649, #15577 ) ) ;
#9246=VECTOR ( 'NONE', #616, 1000.000000000000000 ) ;
#9247=EDGE_LOOP ( 'NONE', ( #17639, #10975, #3404, #8929 ) ) ;
#9249=VERTEX_POINT ( 'NONE', #14581 ) ;
#9250=CARTESIAN_POINT ( 'NONE',  ( -2.879979761448749009, -15.64409473654778893, 1.579620830366336657E-14 ) ) ;
#9251=CARTESIAN_POINT ( 'NONE',  ( -65.30644784966793281, -30.60858878180435738, 4.330127018922217630 ) ) ;
#9252=ORIENTED_EDGE ( 'NONE', *, *, #17170, .F. ) ;
#9253=CARTESIAN_POINT ( 'NONE',  ( -4.565812005419673802, -20.97400746052251108, -21.65063509461098334 ) ) ;
#9254=AXIS2_PLACEMENT_3D ( 'NONE', #12964, #8545, #14320 ) ;
#9257=CARTESIAN_POINT ( 'NONE',  ( 1.399738696879940791, -77.73322974357483872, -21.65063509461098690 ) ) ;
#9258=CIRCLE ( 'NONE', #3183, 1.499999999999999556 ) ;
#9260=FACE_OUTER_BOUND ( 'NONE', #11120, .T. ) ;
#9263=DIRECTION ( 'NONE',  ( -0.1566598588826321747, 0.9876526153536343555, 0.000000000000000000 ) ) ;
#9265=EDGE_CURVE ( 'NONE', #2699, #10382, #9496, .T. ) ;
#9268=DIRECTION ( 'NONE',  ( -0.000000000000000000, -0.000000000000000000, -1.000000000000000000 ) ) ;
#9269=ORIENTED_EDGE ( 'NONE', *, *, #16212, .F. ) ;
#9270=EDGE_LOOP ( 'NONE', ( #4079, #18147 ) ) ;
#9271=VERTEX_POINT ( 'NONE', #18625 ) ;
#9272=CIRCLE ( 'NONE', #14728, 1.500000000000000444 ) ;
#9273=CARTESIAN_POINT ( 'NONE',  ( -62.83731631128384976, -30.21693913459777647, 17.32050807568881723 ) ) ;
#9275=DIRECTION ( 'NONE',  ( -0.9876526153536341335, -0.1566598588826327021, 0.000000000000000000 ) ) ;
#9276=CARTESIAN_POINT ( 'NONE',  ( -34.97868976044174616, -20.73554015023331942, -21.65063509461098334 ) ) ;
#9278=UNCERTAINTY_MEASURE_WITH_UNIT (LENGTH_MEASURE( 1.000000000000000082E-05 ), #681, 'distance_accuracy_value', 'NONE');
#9279=AXIS2_PLACEMENT_3D ( 'NONE', #3535, #13485, #17909 ) ;
#9281=DIRECTION ( 'NONE',  ( 0.9876526153536341335, -0.1566598588826326743, 0.000000000000000000 ) ) ;
#9284=ORIENTED_EDGE ( 'NONE', *, *, #6966, .T. ) ;
#9285=PRESENTATION_STYLE_ASSIGNMENT (( #3489 ) ) ;
#9286=CARTESIAN_POINT ( 'NONE',  ( -77.65210554158829837, -32.56683701783724416, -8.660254037844380193 ) ) ;
#9289=LINE ( 'NONE', #2186, #8159 ) ;
#9290=ORIENTED_EDGE ( 'NONE', *, *, #8245, .F. ) ;
#9291=ORIENTED_EDGE ( 'NONE', *, *, #8676, .F. ) ;
#9292=ORIENTED_EDGE ( 'NONE', *, *, #5420, .T. ) ;
#9293=ORIENTED_EDGE ( 'NONE', *, *, #11202, .F. ) ;
#9294=CARTESIAN_POINT ( 'NONE',  ( -13.41505053342451426, -80.08312762681431707, -12.99038105676658539 ) ) ;
#9295=AXIS2_PLACEMENT_3D ( 'NONE', #14723, #8760, #10088 ) ;
#9296=FACE_BOUND ( 'NONE', #14895, .T. ) ;
#9297=EDGE_CURVE ( 'NONE', #15897, #17878, #11342, .T. ) ;
#9299=DIRECTION ( 'NONE',  ( -0.1566598588826321192, 0.9876526153536342445, 7.798540720466731404E-17 ) ) ;
#9300=CYLINDRICAL_SURFACE ( 'NONE', #1892, 1.500000000000000666 ) ;
#9302=CIRCLE ( 'NONE', #11412, 1.500000000000000888 ) ;
#9303=AXIS2_PLACEMENT_3D ( 'NONE', #143, #4401, #2968 ) ;
#9304=EDGE_LOOP ( 'NONE', ( #17488, #11030, #4778, #11414 ) ) ;
#9305=LINE ( 'NONE', #8936, #14235 ) ;
#9306=CARTESIAN_POINT ( 'NONE',  ( -63.62061560569701157, -25.27867605782963878, -8.660254037844380193 ) ) ;
#9307=CARTESIAN_POINT ( 'NONE',  ( -7.034943543803747090, -21.36565710772908488, 17.32050807568881012 ) ) ;
#9311=ORIENTED_EDGE ( 'NONE', *, *, #7468, .F. ) ;
#9312=DIRECTION ( 'NONE',  ( -0.1566598588826321192, 0.9876526153536342445, 7.798540720466730171E-17 ) ) ;
#9313=CARTESIAN_POINT ( 'NONE',  ( -35.63723437888119605, -83.60797445167352748, -8.660254037844385522 ) ) ;
#9315=DIRECTION ( 'NONE',  ( -0.1566598588826321192, 0.9876526153536342445, 7.798540720466730171E-17 ) ) ;
#9316=ORIENTED_EDGE ( 'NONE', *, *, #16826, .F. ) ;
#9317=ORIENTED_EDGE ( 'NONE', *, *, #270, .T. ) ;
#9318=DIRECTION ( 'NONE',  ( -0.1566598588826321470, 0.9876526153536342445, 0.000000000000000000 ) ) ;
#9321=CIRCLE ( 'NONE', #6928, 1.500000000000000888 ) ;
#9322=VECTOR ( 'NONE', #6492, 1000.000000000000000 ) ;
#9325=AXIS2_PLACEMENT_3D ( 'NONE', #3808, #11113, #8098 ) ;
#9326=ADVANCED_FACE ( 'NONE', ( #8890 ), #13330, .F. ) ;
#9328=DIRECTION ( 'NONE',  ( -0.1566598588826321192, 0.9876526153536342445, 7.798540720466731404E-17 ) ) ;
#9329=ORIENTED_EDGE ( 'NONE', *, *, #11598, .T. ) ;
#9330=CYLINDRICAL_SURFACE ( 'NONE', #292, 1.500000000000001554 ) ;
#9331=DIRECTION ( 'NONE',  ( -0.1566598588826321192, 0.9876526153536342445, 7.798540720466730171E-17 ) ) ;
#9332=CARTESIAN_POINT ( 'NONE',  ( -72.71384246482016067, -31.78353772342409300, 17.32050807568881723 ) ) ;
#9333=ORIENTED_EDGE ( 'NONE', *, *, #8386, .F. ) ;
#9334=ORIENTED_EDGE ( 'NONE', *, *, #8386, .T. ) ;
#9335=CYLINDRICAL_SURFACE ( 'NONE', #8197, 1.500000000000001554 ) ;
#9338=ORIENTED_EDGE ( 'NONE', *, *, #3122, .T. ) ;
#9340=AXIS2_PLACEMENT_3D ( 'NONE', #9219, #15000, #9031 ) ;
#9341=VERTEX_POINT ( 'NONE', #17539 ) ;
#9342=ORIENTED_EDGE ( 'NONE', *, *, #7118, .T. ) ;
#9343=CARTESIAN_POINT ( 'NONE',  ( -56.41757431148526081, -29.19865005186066753, -8.660254037844380193 ) ) ;
#9345=CARTESIAN_POINT ( 'NONE',  ( -20.86208015875458344, -23.55889513208593655, 12.99038105676661736 ) ) ;
#9346=DIRECTION ( 'NONE',  ( 1.000000000000000000, 0.000000000000000000, 0.000000000000000000 ) ) ;
#9349=CARTESIAN_POINT ( 'NONE',  ( -1.109027851681966492, -20.42569795443330349, 21.65063509461101177 ) ) ;
#9351=AXIS2_PLACEMENT_3D ( 'NONE', #11681, #14737, #4327 ) ;
#9352=VECTOR ( 'NONE', #343, 1000.000000000000000 ) ;
#9353=DIRECTION ( 'NONE',  ( -0.1566598588826321747, 0.9876526153536343555, 0.000000000000000000 ) ) ;
#9355=CYLINDRICAL_SURFACE ( 'NONE', #17179, 1.500000000000000888 ) ;
#9356=FACE_BOUND ( 'NONE', #13476, .T. ) ;
#9357=ADVANCED_FACE ( 'NONE', ( #17925 ), #6343, .F. ) ;
#9358=DIRECTION ( 'NONE',  ( -0.1566598588826321192, 0.9876526153536342445, 7.798540720466730171E-17 ) ) ;
#9359=DIRECTION ( 'NONE',  ( -0.1566598588826321192, 0.9876526153536342445, 7.798540720466731404E-17 ) ) ;
#9360=CYLINDRICAL_SURFACE ( 'NONE', #4145, 1.500000000000000666 ) ;
#9361=DIRECTION ( 'NONE',  ( 0.000000000000000000, 0.000000000000000000, 1.000000000000000000 ) ) ;
#9362=ORIENTED_EDGE ( 'NONE', *, *, #7889, .T. ) ;
#9363=AXIS2_PLACEMENT_3D ( 'NONE', #6101, #4656, #1725 ) ;
#9364=DIRECTION ( 'NONE',  ( -0.1566598588826321747, 0.9876526153536343555, 0.000000000000000000 ) ) ;
#9365=ORIENTED_EDGE ( 'NONE', *, *, #1767, .T. ) ;
#9366=AXIS2_PLACEMENT_3D ( 'NONE', #9774, #6945, #2655 ) ;
#9369=CIRCLE ( 'NONE', #1528, 1.500000000000000888 ) ;
#9370=CIRCLE ( 'NONE', #13283, 1.500000000000001332 ) ;
#9371=EDGE_CURVE ( 'NONE', #9146, #18003, #8289, .T. ) ;
#9372=CARTESIAN_POINT ( 'NONE',  ( -28.06512145296634486, -19.63892113805490069, -4.330127018922180326 ) ) ;
#9373=CARTESIAN_POINT ( 'NONE',  ( -9.464440072009985272, -79.45648819128378193, -8.660254037844385522 ) ) ;
#9375=AXIS2_PLACEMENT_3D ( 'NONE', #1427, #3181, #4618 ) ;
#9376=EDGE_CURVE ( 'NONE', #8333, #4400, #7384, .T. ) ;
#9378=EDGE_CURVE ( 'NONE', #8719, #10299, #7976, .T. ) ;
#9380=CARTESIAN_POINT ( 'NONE',  ( 9.300959619708997650, -76.47995087251376845, -21.65063509461098690 ) ) ;
#9381=AXIS2_PLACEMENT_3D ( 'NONE', #18585, #7083, #17121 ) ;
#9382=DIRECTION ( 'NONE',  ( -0.1566598588826321192, 0.9876526153536342445, 7.798540720466730171E-17 ) ) ;
#9383=EDGE_LOOP ( 'NONE', ( #14714, #16583 ) ) ;
#9384=DIRECTION ( 'NONE',  ( -0.1566598588826321192, 0.9876526153536342445, 7.798540720466731404E-17 ) ) ;
#9385=ORIENTED_EDGE ( 'NONE', *, *, #9265, .T. ) ;
#9386=FACE_BOUND ( 'NONE', #9942, .T. ) ;
#9389=DIRECTION ( 'NONE',  ( -0.9876526153536341335, -0.1566598588826327021, 0.000000000000000000 ) ) ;
#9391=CARTESIAN_POINT ( 'NONE',  ( -53.94844277310116354, -28.80700040465408662, 21.65063509461101887 ) ) ;
#9393=EDGE_CURVE ( 'NONE', #5203, #9088, #3178, .T. ) ;
#9394=ORIENTED_EDGE ( 'NONE', *, *, #13623, .T. ) ;
#9396=EDGE_LOOP ( 'NONE', ( #11695, #565 ) ) ;
#9397=VERTEX_POINT ( 'NONE', #13232 ) ;
#9398=CIRCLE ( 'NONE', #3316, 1.500000000000000444 ) ;
#9399=EDGE_LOOP ( 'NONE', ( #18572, #5430 ) ) ;
#9400=DIRECTION ( 'NONE',  ( -0.1566598588826321192, 0.9876526153536342445, 7.798540720466731404E-17 ) ) ;
#9401=VECTOR ( 'NONE', #16972, 1000.000000000000000 ) ;
#9402=FACE_BOUND ( 'NONE', #4108, .T. ) ;
#9405=CIRCLE ( 'NONE', #4846, 1.500000000000000888 ) ;
#9406=AXIS2_PLACEMENT_3D ( 'NONE', #11407, #15797, #17052 ) ;
#9407=ADVANCED_FACE ( 'NONE', ( #3270 ), #6154, .F. ) ;
#9408=EDGE_CURVE ( 'NONE', #1267, #9967, #10384, .T. ) ;
#9409=DIRECTION ( 'NONE',  ( 0.000000000000000000, 0.000000000000000000, 1.000000000000000000 ) ) ;
#9410=AXIS2_PLACEMENT_3D ( 'NONE', #3649, #16562, #8220 ) ;
#9413=CARTESIAN_POINT ( 'NONE',  ( 4.362696542940843081, -77.26325016692693737, 4.330127018922209636 ) ) ;
#9414=PRODUCT_DEFINITION ( 'UNKNOWN', '', #10218, #11298 ) ;
#9415=ADVANCED_FACE ( 'NONE', ( #7743 ), #14851, .F. ) ;
#9416=DIRECTION ( 'NONE',  ( -0.9876526153536341335, -0.1566598588826327021, 0.000000000000000000 ) ) ;
#9417=ORIENTED_EDGE ( 'NONE', *, *, #11966, .F. ) ;
#9418=ORIENTED_EDGE ( 'NONE', *, *, #7425, .F. ) ;
#9419=CARTESIAN_POINT ( 'NONE',  ( -21.81009776393036503, -81.41473642731668292, 4.330127018922213189 ) ) ;
#9420=DIRECTION ( 'NONE',  ( -0.1566598588826321192, 0.9876526153536342445, 7.798540720466731404E-17 ) ) ;
#9421=AXIS2_PLACEMENT_3D ( 'NONE', #3617, #13394, #6217 ) ;
#9422=ORIENTED_EDGE ( 'NONE', *, *, #1524, .T. ) ;
#9423=DIRECTION ( 'NONE',  ( -0.1566598588826321747, 0.9876526153536343555, 0.000000000000000000 ) ) ;
#9424=ORIENTED_EDGE ( 'NONE', *, *, #3668, .F. ) ;
#9425=DIRECTION ( 'NONE',  ( -0.1566598588826321747, 0.9876526153536343555, 0.000000000000000000 ) ) ;
#9427=VECTOR ( 'NONE', #1017, 1000.000000000000000 ) ;
#9428=CYLINDRICAL_SURFACE ( 'NONE', #7590, 1.500000000000001554 ) ;
#9429=CIRCLE ( 'NONE', #1284, 1.500000000000000888 ) ;
#9433=DIRECTION ( 'NONE',  ( 0.000000000000000000, 0.000000000000000000, 1.000000000000000000 ) ) ;
#9435=EDGE_CURVE ( 'NONE', #1456, #11968, #5252, .T. ) ;
#9436=CIRCLE ( 'NONE', #10330, 1.500000000000000888 ) ;
#9437=CARTESIAN_POINT ( 'NONE',  ( -46.33669483700850122, -22.53712852738357952, -21.65063509461097979 ) ) ;
#9438=EDGE_LOOP ( 'NONE', ( #14254, #14295 ) ) ;
#9439=EDGE_CURVE ( 'NONE', #3971, #4926, #10085, .T. ) ;
#9440=ORIENTED_EDGE ( 'NONE', *, *, #3902, .F. ) ;
#9442=CARTESIAN_POINT ( 'NONE',  ( -50.49165861936349131, -28.25869089856488614, -12.99038105676658006 ) ) ;
#9443=EDGE_LOOP ( 'NONE', ( #9064, #3549 ) ) ;
#9444=VECTOR ( 'NONE', #1777, 1000.000000000000000 ) ;
#9446=DIRECTION ( 'NONE',  ( -0.1566598588826321747, 0.9876526153536343555, 0.000000000000000000 ) ) ;
#9447=EDGE_LOOP ( 'NONE', ( #298, #15458, #11152, #4985 ) ) ;
#9448=VERTEX_POINT ( 'NONE', #9643 ) ;
#9449=VECTOR ( 'NONE', #10606, 1000.000000000000000 ) ;
#9450=DIRECTION ( 'NONE',  ( -0.9876526153536341335, -0.1566598588826327021, 0.000000000000000000 ) ) ;
#9452=CARTESIAN_POINT ( 'NONE',  ( -18.18859529943003750, -18.07232254922858417, -4.330127018922180326 ) ) ;
#9453=CARTESIAN_POINT ( 'NONE',  ( -79.13358446461874962, -32.80182680616118773, 8.660254037844417496 ) ) ;
#9454=DIRECTION ( 'NONE',  ( -3.208277787129350839E-17, -0.000000000000000000, 1.000000000000000000 ) ) ;
#9455=VECTOR ( 'NONE', #9698, 1000.000000000000000 ) ;
#9456=CARTESIAN_POINT ( 'NONE',  ( -15.71946376104596155, -17.68067290202200326, 17.32050807568881012 ) ) ;
#9457=CYLINDRICAL_SURFACE ( 'NONE', #13787, 1.500000000000001554 ) ;
#9458=LINE ( 'NONE', #15230, #4164 ) ;
#9459=CARTESIAN_POINT ( 'NONE',  ( -48.80582637539254875, -22.92877817459017464, 17.32050807568882078 ) ) ;
#9460=DIRECTION ( 'NONE',  ( -0.1566598588826321192, 0.9876526153536342445, 7.798540720466730171E-17 ) ) ;
#9461=VERTEX_POINT ( 'NONE', #15317 ) ;
#9462=ORIENTED_EDGE ( 'NONE', *, *, #2145, .F. ) ;
#9463=DIRECTION ( 'NONE',  ( -0.1566598588826321192, 0.9876526153536342445, 7.798540720466730171E-17 ) ) ;
#9465=ORIENTED_EDGE ( 'NONE', *, *, #9575, .F. ) ;
#9466=ORIENTED_EDGE ( 'NONE', *, *, #3564, .T. ) ;
#9467=VECTOR ( 'NONE', #9668, 1000.000000000000000 ) ;
#9468=FACE_OUTER_BOUND ( 'NONE', #18143, .T. ) ;
#9470=ORIENTED_EDGE ( 'NONE', *, *, #16946, .F. ) ;
#9471=ORIENTED_EDGE ( 'NONE', *, *, #7495, .T. ) ;
#9472=DIRECTION ( 'NONE',  ( -0.1566598588826321747, 0.9876526153536343555, 0.000000000000000000 ) ) ;
#9473=ORIENTED_EDGE ( 'NONE', *, *, #15531, .T. ) ;
#9474=DIRECTION ( 'NONE',  ( -0.9876526153536341335, -0.1566598588826327021, 0.000000000000000000 ) ) ;
#9475=DIRECTION ( 'NONE',  ( 1.000000000000000000, 0.000000000000000000, -0.000000000000000000 ) ) ;
#9476=CARTESIAN_POINT ( 'NONE',  ( -26.58364252993588650, -19.40393134973096068, 21.65063509461102242 ) ) ;
#9479=VERTEX_POINT ( 'NONE', #10845 ) ;
#9481=AXIS2_PLACEMENT_3D ( 'NONE', #10028, #1608, #8622 ) ;
#9482=CARTESIAN_POINT ( 'NONE',  ( -62.83731631128384976, -30.21693913459777647, 17.32050807568881723 ) ) ;
#9483=ORIENTED_EDGE ( 'NONE', *, *, #3150, .T. ) ;
#9485=ORIENTED_EDGE ( 'NONE', *, *, #9030, .T. ) ;
#9486=ORIENTED_EDGE ( 'NONE', *, *, #13124, .T. ) ;
#9487=DIRECTION ( 'NONE',  ( -0.1566598588826321192, 0.9876526153536342445, 7.798540720466730171E-17 ) ) ;
#9488=ORIENTED_EDGE ( 'NONE', *, *, #2307, .T. ) ;
#9489=ORIENTED_EDGE ( 'NONE', *, *, #1246, .F. ) ;
#9491=EDGE_CURVE ( 'NONE', #1168, #8810, #17688, .T. ) ;
#9492=EDGE_CURVE ( 'NONE', #6188, #7482, #2838, .T. ) ;
#9493=VERTEX_POINT ( 'NONE', #11034 ) ;
#9494=FACE_BOUND ( 'NONE', #17874, .T. ) ;
#9495=EDGE_CURVE ( 'NONE', #14919, #4926, #15418, .T. ) ;
#9496=CIRCLE ( 'NONE', #9186, 1.499999999999999556 ) ;
#9498=ORIENTED_EDGE ( 'NONE', *, *, #9598, .T. ) ;
#9499=CARTESIAN_POINT ( 'NONE',  ( -26.74836084069852404, -82.19803572172983763, -21.65063509461098690 ) ) ;
#9500=FACE_BOUND ( 'NONE', #1880, .T. ) ;
#9501=DIRECTION ( 'NONE',  ( -0.9876526153536336894, -0.1566598588826349503, 0.000000000000000000 ) ) ;
#9502=DIRECTION ( 'NONE',  ( -0.1566598588826321192, 0.9876526153536342445, 7.798540720466731404E-17 ) ) ;
#9503=DIRECTION ( 'NONE',  ( -0.1566598588826321192, 0.9876526153536342445, 7.798540720466731404E-17 ) ) ;
#9504=DIRECTION ( 'NONE',  ( 0.000000000000000000, 0.000000000000000000, 1.000000000000000000 ) ) ;
#9506=ORIENTED_EDGE ( 'NONE', *, *, #9852, .F. ) ;
#9510=DIRECTION ( 'NONE',  ( -0.1566598588826321192, 0.9876526153536342445, 7.798540720466730171E-17 ) ) ;
#9511=EDGE_LOOP ( 'NONE', ( #13619, #11517, #9466, #13166 ) ) ;
#9513=VERTEX_POINT ( 'NONE', #16670 ) ;
#9514=LINE ( 'NONE', #2585, #9120 ) ;
#9516=ORIENTED_EDGE ( 'NONE', *, *, #3274, .F. ) ;
#9517=CARTESIAN_POINT ( 'NONE',  ( -19.34096622554629263, -81.02308678011010556, 8.660254037844412167 ) ) ;
#9519=CARTESIAN_POINT ( 'NONE',  ( -52.92115514756972061, -86.34952198211959740, 4.330127018922213189 ) ) ;
#9520=FACE_OUTER_BOUND ( 'NONE', #14827, .T. ) ;
#9522=DIRECTION ( 'NONE',  ( -0.1566598588826321192, 0.9876526153536342445, 7.798540720466730171E-17 ) ) ;
#9523=DIRECTION ( 'NONE',  ( -0.1566598588826321192, 0.9876526153536342445, 7.798540720466731404E-17 ) ) ;
#9524=CARTESIAN_POINT ( 'NONE',  ( -36.46016868347218320, -20.97052993855727365, 4.330127018922218518 ) ) ;
#9525=DIRECTION ( 'NONE',  ( 0.000000000000000000, 0.000000000000000000, 1.000000000000000000 ) ) ;
#9526=CARTESIAN_POINT ( 'NONE',  ( -68.72359699322777260, -88.85607972424168111, 1.424741226644455312E-14 ) ) ;
#9527=VERTEX_POINT ( 'NONE', #4971 ) ;
#9528=ORIENTED_EDGE ( 'NONE', *, *, #14034, .F. ) ;
#9529=DIRECTION ( 'NONE',  ( -0.1566598588826321192, 0.9876526153536342445, 7.798540720466731404E-17 ) ) ;
#9530=VERTEX_POINT ( 'NONE', #13993 ) ;
#9531=ORIENTED_EDGE ( 'NONE', *, *, #4297, .F. ) ;
#9532=DIRECTION ( 'NONE',  ( -0.9876526153536336894, -0.1566598588826350336, 0.000000000000000000 ) ) ;
#9533=ORIENTED_EDGE ( 'NONE', *, *, #8831, .F. ) ;
#9534=VERTEX_POINT ( 'NONE', #16564 ) ;
#9535=CARTESIAN_POINT ( 'NONE',  ( -6.830590222863280658, -16.27073417207831696, 21.65063509461101532 ) ) ;
#9536=VERTEX_POINT ( 'NONE', #1046 ) ;
#9537=AXIS2_PLACEMENT_3D ( 'NONE', #11781, #8956, #8878 ) ;
#9538=DIRECTION ( 'NONE',  ( -0.1566598588826321192, 0.9876526153536342445, 7.798540720466730171E-17 ) ) ;
#9539=EDGE_CURVE ( 'NONE', #272, #1095, #8020, .T. ) ;
#9541=CARTESIAN_POINT ( 'NONE',  ( -72.71384246482016067, -31.78353772342409300, -8.660254037844380193 ) ) ;
#9542=EDGE_CURVE ( 'NONE', #17453, #16580, #3548, .T. ) ;
#9543=CARTESIAN_POINT ( 'NONE',  ( -64.60826822105063627, -25.43533591671228322, 12.99038105676661736 ) ) ;
#9546=DIRECTION ( 'NONE',  ( -0.9876526153536336894, -0.1566598588826349503, 0.000000000000000000 ) ) ;
#9547=DIRECTION ( 'NONE',  ( -0.9876526153536336894, -0.1566598588826349503, 0.000000000000000000 ) ) ;
#9548=ORIENTED_EDGE ( 'NONE', *, *, #7054, .T. ) ;
#9549=CARTESIAN_POINT ( 'NONE',  ( -56.21322099054477661, -24.10372711620991026, 12.99038105676661736 ) ) ;
#9550=CARTESIAN_POINT ( 'NONE',  ( -0.1213752363283457369, -20.26903809555066616, 17.32050807568881012 ) ) ;
#9551=AXIS2_PLACEMENT_3D ( 'NONE', #10906, #13950, #3884 ) ;
#9552=CYLINDRICAL_SURFACE ( 'NONE', #14142, 1.500000000000000666 ) ;
#9553=EDGE_LOOP ( 'NONE', ( #15602, #16434 ) ) ;
#9554=ORIENTED_EDGE ( 'NONE', *, *, #8121, .F. ) ;
#9555=CYLINDRICAL_SURFACE ( 'NONE', #12301, 1.500000000000001554 ) ;
#9557=DIRECTION ( 'NONE',  ( -0.9876526153536341335, -0.1566598588826327021, 0.000000000000000000 ) ) ;
#9558=ORIENTED_EDGE ( 'NONE', *, *, #14153, .T. ) ;
#9559=ORIENTED_EDGE ( 'NONE', *, *, #5834, .F. ) ;
#9561=DIRECTION ( 'NONE',  ( -0.1566598588826321192, 0.9876526153536342445, 7.798540720466730171E-17 ) ) ;
#9562=EDGE_CURVE ( 'NONE', #7482, #6188, #18327, .T. ) ;
#9563=CARTESIAN_POINT ( 'NONE',  ( -55.42992169613161479, -29.04199019297804085, 21.65063509461101887 ) ) ;
#9564=AXIS2_PLACEMENT_3D ( 'NONE', #556, #6350, #264 ) ;
#9565=DIRECTION ( 'NONE',  ( -0.9876526153536336894, -0.1566598588826349503, 0.000000000000000000 ) ) ;
#9566=DIRECTION ( 'NONE',  ( 0.000000000000000000, 0.000000000000000000, 1.000000000000000000 ) ) ;
#9567=EDGE_CURVE ( 'NONE', #11513, #893, #5190, .T. ) ;
#9569=DIRECTION ( 'NONE',  ( -0.9876526153536336894, -0.1566598588826350336, 0.000000000000000000 ) ) ;
#9570=DIRECTION ( 'NONE',  ( -0.9876526153536336894, -0.1566598588826349503, 0.000000000000000000 ) ) ;
#9571=VERTEX_POINT ( 'NONE', #9543 ) ;
#9572=DIRECTION ( 'NONE',  ( -0.1566598588826321747, 0.9876526153536343555, 0.000000000000000000 ) ) ;
#9573=DIRECTION ( 'NONE',  ( 0.000000000000000000, 0.000000000000000000, 1.000000000000000000 ) ) ;
#9574=AXIS2_PLACEMENT_3D ( 'NONE', #6661, #9400, #10791 ) ;
#9575=EDGE_CURVE ( 'NONE', #2965, #9461, #16961, .T. ) ;
#9576=CYLINDRICAL_SURFACE ( 'NONE', #17868, 1.500000000000000666 ) ;
#9578=ORIENTED_EDGE ( 'NONE', *, *, #8908, .F. ) ;
#9579=EDGE_LOOP ( 'NONE', ( #7056, #14903, #4185, #7932 ) ) ;
#9580=FACE_OUTER_BOUND ( 'NONE', #10437, .T. ) ;
#9581=FACE_BOUND ( 'NONE', #10196, .T. ) ;
#9583=VERTEX_POINT ( 'NONE', #10950 ) ;
#9585=AXIS2_PLACEMENT_3D ( 'NONE', #11780, #13214, #4683 ) ;
#9586=ORIENTED_EDGE ( 'NONE', *, *, #6582, .F. ) ;
#9589=VERTEX_POINT ( 'NONE', #9453 ) ;
#9590=CARTESIAN_POINT ( 'NONE',  ( -57.85941822433786541, -87.13282127653273790, -21.65063509461098690 ) ) ;
#9592=FACE_OUTER_BOUND ( 'NONE', #11002, .T. ) ;
#9594=CARTESIAN_POINT ( 'NONE',  ( -28.26947477390680774, -24.73384407370567217, -8.660254037844380193 ) ) ;
#9595=AXIS2_PLACEMENT_3D ( 'NONE', #18696, #11046, #11141 ) ;
#9596=ORIENTED_EDGE ( 'NONE', *, *, #7179, .T. ) ;
#9597=DIRECTION ( 'NONE',  ( 0.000000000000000000, 0.000000000000000000, 1.000000000000000000 ) ) ;
#9598=EDGE_CURVE ( 'NONE', #334, #999, #10094, .T. ) ;
#9600=DIRECTION ( 'NONE',  ( -0.9876526153536336894, -0.1566598588826349503, 0.000000000000000000 ) ) ;
#9601=ORIENTED_EDGE ( 'NONE', *, *, #8817, .T. ) ;
#9602=EDGE_LOOP ( 'NONE', ( #16467, #12569, #17140, #7660 ) ) ;
#9603=CARTESIAN_POINT ( 'NONE',  ( -40.08167114797250719, -84.31294381664535820, 4.330127018922213189 ) ) ;
#9604=AXIS2_PLACEMENT_3D ( 'NONE', #7166, #14162, #2598 ) ;
#9606=ORIENTED_EDGE ( 'NONE', *, *, #12042, .T. ) ;
#9608=AXIS2_PLACEMENT_3D ( 'NONE', #6408, #9226, #2023 ) ;
#9609=CARTESIAN_POINT ( 'NONE',  ( -23.33121169713865584, -23.95054477929251036, 1.869203119972154228E-14 ) ) ;
#9610=ORIENTED_EDGE ( 'NONE', *, *, #11854, .T. ) ;
#9611=FACE_BOUND ( 'NONE', #10775, .T. ) ;
#9614=DIRECTION ( 'NONE',  ( -0.1566598588826321192, 0.9876526153536342445, 7.798540720466731404E-17 ) ) ;
#9618=EDGE_CURVE ( 'NONE', #18673, #14612, #12512, .T. ) ;
#9619=CARTESIAN_POINT ( 'NONE',  ( -56.37793930130741415, -86.89783148820880854, 12.99038105676661203 ) ) ;
#9622=CIRCLE ( 'NONE', #12007, 1.500000000000001332 ) ;
#9623=CARTESIAN_POINT ( 'NONE',  ( -72.71384246482016067, -31.78353772342409300, 1.869203119972154228E-14 ) ) ;
#9624=ADVANCED_FACE ( 'NONE', ( #12751 ), #6905, .F. ) ;
#9626=ORIENTED_EDGE ( 'NONE', *, *, #7093, .T. ) ;
#9629=CARTESIAN_POINT ( 'NONE',  ( 2.881217619910392269, -77.49823995525089515, 21.65063509461100821 ) ) ;
#9630=ORIENTED_EDGE ( 'NONE', *, *, #10314, .F. ) ;
#9631=ADVANCED_FACE ( 'NONE', ( #11236 ), #18604, .F. ) ;
#9632=VERTEX_POINT ( 'NONE', #17055 ) ;
#9634=CARTESIAN_POINT ( 'NONE',  ( -74.48479437458692587, -27.00193450553858909, -12.99038105676658006 ) ) ;
#9636=ORIENTED_EDGE ( 'NONE', *, *, #12142, .T. ) ;
#9637=LINE ( 'NONE', #16955, #10616 ) ;
#9638=AXIS2_PLACEMENT_3D ( 'NONE', #17034, #16747, #3718 ) ;
#9639=CARTESIAN_POINT ( 'NONE',  ( -72.71384246482016067, -31.78353772342409300, -17.32050807568878170 ) ) ;
#9640=CARTESIAN_POINT ( 'NONE',  ( -27.73601345605213098, -82.35469558061245721, 7.492215382409427462E-15 ) ) ;
#9642=DIRECTION ( 'NONE',  ( -0.1566598588826321192, 0.9876526153536342445, 7.798540720466730171E-17 ) ) ;
#9643=CARTESIAN_POINT ( 'NONE',  ( -56.41757431148524660, -29.19865005186066043, 8.660254037844417496 ) ) ;
#9644=FACE_OUTER_BOUND ( 'NONE', #18562, .T. ) ;
#9645=ADVANCED_FACE ( 'NONE', ( #2714 ), #5475, .F. ) ;
#9647=ORIENTED_EDGE ( 'NONE', *, *, #5975, .F. ) ;
#9648=AXIS2_PLACEMENT_3D ( 'NONE', #3728, #9529, #15302 ) ;
#9649=DIRECTION ( 'NONE',  ( -0.9876526153536341335, -0.1566598588826327576, 0.000000000000000000 ) ) ;
#9650=CIRCLE ( 'NONE', #16001, 1.500000000000000888 ) ;
#9651=DIRECTION ( 'NONE',  ( -0.1566598588826321192, 0.9876526153536342445, 7.798540720466730171E-17 ) ) ;
#9652=DIRECTION ( 'NONE',  ( -0.1566598588826321192, 0.9876526153536342445, 7.798540720466731404E-17 ) ) ;
#9653=CIRCLE ( 'NONE', #17548, 1.500000000000001332 ) ;
#9655=CARTESIAN_POINT ( 'NONE',  ( -30.20514499443620338, -82.74634522781904877, 12.99038105676661203 ) ) ;
#9660=CARTESIAN_POINT ( 'NONE',  ( -60.36818477289978091, -29.82528948739120267, -4.330127018922181215 ) ) ;
#9661=ORIENTED_EDGE ( 'NONE', *, *, #2973, .F. ) ;
#9662=ORIENTED_EDGE ( 'NONE', *, *, #9782, .F. ) ;
#9663=VECTOR ( 'NONE', #5526, 1000.000000000000000 ) ;
#9664=CIRCLE ( 'NONE', #15099, 1.499999999999999556 ) ;
#9666=EDGE_LOOP ( 'NONE', ( #17208, #9057 ) ) ;
#9667=CIRCLE ( 'NONE', #7271, 1.500000000000001332 ) ;
#9668=DIRECTION ( 'NONE',  ( -0.1566598588826321192, 0.9876526153536342445, 7.798540720466730171E-17 ) ) ;
#9669=AXIS2_PLACEMENT_3D ( 'NONE', #3281, #9082, #16396 ) ;
#9671=FACE_OUTER_BOUND ( 'NONE', #3811, .T. ) ;
#9672=DIRECTION ( 'NONE',  ( -0.1566598588826321192, 0.9876526153536342445, 7.798540720466730171E-17 ) ) ;
#9673=CARTESIAN_POINT ( 'NONE',  ( -51.27495791377664602, -23.32042782179673779, -21.65063509461097979 ) ) ;
#9674=CARTESIAN_POINT ( 'NONE',  ( 2.058283315319403783, -14.86079544213463066, 17.32050807568881012 ) ) ;
#9676=CARTESIAN_POINT ( 'NONE',  ( -79.24244631363546887, 32.81909429640987952, 25.00000000000001776 ) ) ;
#9677=CIRCLE ( 'NONE', #17567, 1.500000000000000000 ) ;
#9679=DIRECTION ( 'NONE',  ( 0.000000000000000000, 0.000000000000000000, 1.000000000000000000 ) ) ;
#9681=EDGE_CURVE ( 'NONE', #14889, #211, #48, .T. ) ;
#9682=AXIS2_PLACEMENT_3D ( 'NONE', #13508, #17930, #6348 ) ;
#9684=DIRECTION ( 'NONE',  ( -0.1566598588826321747, 0.9876526153536343555, 0.000000000000000000 ) ) ;
#9685=EDGE_CURVE ( 'NONE', #9589, #11379, #9514, .T. ) ;
#9686=EDGE_CURVE ( 'NONE', #3473, #5485, #3385, .T. ) ;
#9687=AXIS2_PLACEMENT_3D ( 'NONE', #16078, #10179, #13032 ) ;
#9688=CIRCLE ( 'NONE', #8433, 1.500000000000000444 ) ;
#9689=AXIS2_PLACEMENT_3D ( 'NONE', #1550, #17576, #10333 ) ;
#9691=ORIENTED_EDGE ( 'NONE', *, *, #10082, .F. ) ;
#9692=ORIENTED_EDGE ( 'NONE', *, *, #8209, .F. ) ;
#9693=DIRECTION ( 'NONE',  ( -0.9876526153536336894, -0.1566598588826349503, 0.000000000000000000 ) ) ;
#9694=ADVANCED_FACE ( 'NONE', ( #2298 ), #18282, .F. ) ;
#9695=ORIENTED_EDGE ( 'NONE', *, *, #3449, .F. ) ;
#9696=FACE_BOUND ( 'NONE', #11268, .T. ) ;
#9697=AXIS2_PLACEMENT_3D ( 'NONE', #16105, #5875, #7392 ) ;
#9698=DIRECTION ( 'NONE',  ( -0.1566598588826321192, 0.9876526153536342445, 7.798540720466730171E-17 ) ) ;
#9699=AXIS2_PLACEMENT_3D ( 'NONE', #322, #11754, #3421 ) ;
#9700=ORIENTED_EDGE ( 'NONE', *, *, #339, .T. ) ;
#9701=AXIS2_PLACEMENT_3D ( 'NONE', #7730, #6324, #2131 ) ;
#9702=AXIS2_PLACEMENT_3D ( 'NONE', #13637, #17845, #4823 ) ;
#9703=CARTESIAN_POINT ( 'NONE',  ( -56.91140061916208737, -29.27697998130198442, -21.65063509461098334 ) ) ;
#9707=DIRECTION ( 'NONE',  ( 0.000000000000000000, 0.000000000000000000, 1.000000000000000000 ) ) ;
#9708=DIRECTION ( 'NONE',  ( -0.1566598588826321192, 0.9876526153536342445, 7.798540720466731404E-17 ) ) ;
#9709=AXIS2_PLACEMENT_3D ( 'NONE', #8526, #18704, #82 ) ;
#9710=CARTESIAN_POINT ( 'NONE',  ( -50.49165861936347710, -28.25869089856488614, 4.330127018922217630 ) ) ;
#9711=CARTESIAN_POINT ( 'NONE',  ( -52.42732883989288695, -86.27119205267824498, -17.32050807568878525 ) ) ;
#9712=CIRCLE ( 'NONE', #6684, 1.500000000000000888 ) ;
#9713=LINE ( 'NONE', #15480, #17210 ) ;
#9714=ORIENTED_EDGE ( 'NONE', *, *, #5446, .F. ) ;
#9715=EDGE_LOOP ( 'NONE', ( #6228, #6917, #3826, #13079 ) ) ;
#9717=CYLINDRICAL_SURFACE ( 'NONE', #15780, 1.500000000000001554 ) ;
#9718=ADVANCED_FACE ( 'NONE', ( #12440 ), #9717, .F. ) ;
#9720=ORIENTED_EDGE ( 'NONE', *, *, #712, .F. ) ;
#9721=DIRECTION ( 'NONE',  ( -0.1566598588826321192, 0.9876526153536342445, 7.798540720466730171E-17 ) ) ;
#9723=CARTESIAN_POINT ( 'NONE',  ( -33.99103714508810725, -20.57888029135068919, -8.660254037844380193 ) ) ;
#9724=ADVANCED_FACE ( 'NONE', ( #12233 ), #10915, .F. ) ;
#9725=CIRCLE ( 'NONE', #7016, 1.500000000000001332 ) ;
#9726=EDGE_CURVE ( 'NONE', #14841, #777, #11518, .T. ) ;
#9727=CIRCLE ( 'NONE', #1554, 1.499999999999999556 ) ;
#9728=DIRECTION ( 'NONE',  ( -0.1566598588826321192, 0.9876526153536342445, 7.798540720466730171E-17 ) ) ;
#9729=CARTESIAN_POINT ( 'NONE',  ( -63.78533391645962780, -88.07278042982852639, -17.32050807568878525 ) ) ;
#9731=ORIENTED_EDGE ( 'NONE', *, *, #7989, .T. ) ;
#9733=VECTOR ( 'NONE', #5653, 1000.000000000000000 ) ;
#9734=CARTESIAN_POINT ( 'NONE',  ( -5.842937607509656850, -16.11407431319567962, 1.561251128379126385E-14 ) ) ;
#9735=ORIENTED_EDGE ( 'NONE', *, *, #11331, .F. ) ;
#9736=ORIENTED_EDGE ( 'NONE', *, *, #8270, .T. ) ;
#9737=CARTESIAN_POINT ( 'NONE',  ( -31.52190560670403841, -20.18723064414410828, -21.65063509461097979 ) ) ;
#9738=ORIENTED_EDGE ( 'NONE', *, *, #952, .T. ) ;
#9739=CIRCLE ( 'NONE', #1859, 1.500000000000000888 ) ;
#9740=VERTEX_POINT ( 'NONE', #13852 ) ;
#9741=DIRECTION ( 'NONE',  ( -0.9876526153536336894, -0.1566598588826349503, 0.000000000000000000 ) ) ;
#9742=EDGE_CURVE ( 'NONE', #13568, #14760, #10058, .T. ) ;
#9743=VECTOR ( 'NONE', #8191, 1000.000000000000000 ) ;
#9744=ADVANCED_FACE ( 'NONE', ( #3796 ), #2393, .F. ) ;
#9745=DIRECTION ( 'NONE',  ( -0.1566598588826321192, 0.9876526153536342445, 7.798540720466731404E-17 ) ) ;
#9746=EDGE_CURVE ( 'NONE', #8251, #1703, #18245, .T. ) ;
#9748=FACE_OUTER_BOUND ( 'NONE', #317, .T. ) ;
#9750=CARTESIAN_POINT ( 'NONE',  ( -62.79768130110601021, -87.91612057094590682, -4.330127018922185655 ) ) ;
#9751=CIRCLE ( 'NONE', #12126, 139.0000000000000000 ) ;
#9752=CARTESIAN_POINT ( 'NONE',  ( -78.43540483600145308, -27.62857394106911713, 1.908195823574487804E-14 ) ) ;
#9753=ORIENTED_EDGE ( 'NONE', *, *, #3899, .T. ) ;
#9754=CARTESIAN_POINT ( 'NONE',  ( -14.44233815895597672, -22.54060604934882051, -4.330127018922181215 ) ) ;
#9755=LINE ( 'NONE', #4123, #15634 ) ;
#9758=DIRECTION ( 'NONE',  ( -0.1566598588826321747, 0.9876526153536343555, 0.000000000000000000 ) ) ;
#9759=VERTEX_POINT ( 'NONE', #5343 ) ;
#9762=VERTEX_POINT ( 'NONE', #11197 ) ;
#9763=AXIS2_PLACEMENT_3D ( 'NONE', #6277, #6553, #12111 ) ;
#9765=DIRECTION ( 'NONE',  ( -0.9876526153536341335, -0.1566598588826327021, 0.000000000000000000 ) ) ;
#9766=CIRCLE ( 'NONE', #7354, 1.500000000000000888 ) ;
#9767=CARTESIAN_POINT ( 'NONE',  ( -18.35331361019266794, -80.86642692122747178, -4.330127018922185655 ) ) ;
#9768=CARTESIAN_POINT ( 'NONE',  ( -43.04462899403339549, -84.78292339329328797, 21.65063509461101532 ) ) ;
#9769=DIRECTION ( 'NONE',  ( -0.1566598588826321192, 0.9876526153536342445, 7.798540720466731404E-17 ) ) ;
#9770=FACE_OUTER_BOUND ( 'NONE', #17631, .T. ) ;
#9772=DIRECTION ( 'NONE',  ( -0.1566598588826321192, 0.9876526153536342445, 7.798540720466730171E-17 ) ) ;
#9773=DIRECTION ( 'NONE',  ( 1.000000000000000000, 0.000000000000000000, 0.000000000000000000 ) ) ;
#9774=CARTESIAN_POINT ( 'NONE',  ( -24.27922930231443743, -81.80638607452326028, -8.660254037844385522 ) ) ;
#9775=AXIS2_PLACEMENT_3D ( 'NONE', #18156, #885, #18355 ) ;
#9776=ORIENTED_EDGE ( 'NONE', *, *, #9033, .T. ) ;
#9778=DIRECTION ( 'NONE',  ( -0.9876526153536344665, -0.1566598588826304539, 0.000000000000000000 ) ) ;
#9779=FACE_BOUND ( 'NONE', #9270, .T. ) ;
#9782=EDGE_CURVE ( 'NONE', #16555, #3259, #2503, .T. ) ;
#9783=EDGE_CURVE ( 'NONE', #13246, #862, #15380, .T. ) ;
#9784=AXIS2_PLACEMENT_3D ( 'NONE', #12803, #1357, #20 ) ;
#9785=LINE ( 'NONE', #2379, #16309 ) ;
#9786=LINE ( 'NONE', #2571, #11833 ) ;
#9787=ORIENTED_EDGE ( 'NONE', *, *, #2090, .F. ) ;
#9788=ADVANCED_FACE ( 'NONE', ( #13959 ), #17020, .F. ) ;
#9789=CARTESIAN_POINT ( 'NONE',  ( -14.40270314877813895, -80.23978748569695085, -8.660254037844385522 ) ) ;
#9790=CARTESIAN_POINT ( 'NONE',  ( -49.50400600400985240, -28.10203103968224880, 17.32050807568881723 ) ) ;
#9792=DIRECTION ( 'NONE',  ( -0.1566598588826321747, 0.9876526153536343555, 0.000000000000000000 ) ) ;
#9793=ORIENTED_EDGE ( 'NONE', *, *, #4063, .T. ) ;
#9795=ORIENTED_EDGE ( 'NONE', *, *, #12756, .T. ) ;
#9797=DIRECTION ( 'NONE',  ( -0.1566598588826321192, 0.9876526153536342445, 7.798540720466731404E-17 ) ) ;
#9800=EDGE_LOOP ( 'NONE', ( #10618, #7458 ) ) ;
#9802=CARTESIAN_POINT ( 'NONE',  ( -10.28737437660098308, -16.81904367816752810, -21.65063509461098334 ) ) ;
#9803=CARTESIAN_POINT ( 'NONE',  ( -77.44775222064782838, -27.47191408218648334, -4.330127018922180326 ) ) ;
#9807=CARTESIAN_POINT ( 'NONE',  ( -15.39035576413176187, -80.39644734457958464, 12.99038105676661203 ) ) ;
#9808=DIRECTION ( 'NONE',  ( -0.1566598588826321192, 0.9876526153536342445, 7.798540720466731404E-17 ) ) ;
#9809=DIRECTION ( 'NONE',  ( 0.000000000000000000, 0.000000000000000000, 1.000000000000000000 ) ) ;
#9811=ORIENTED_EDGE ( 'NONE', *, *, #10711, .F. ) ;
#9812=CARTESIAN_POINT ( 'NONE',  ( -45.55339554259532520, -27.47539160415171722, 4.330127018922217630 ) ) ;
#9813=CARTESIAN_POINT ( 'NONE',  ( -51.47931123471710890, -28.41535075744750571, 8.660254037844417496 ) ) ;
#9814=EDGE_CURVE ( 'NONE', #10257, #2545, #16092, .T. ) ;
#9815=ORIENTED_EDGE ( 'NONE', *, *, #11791, .F. ) ;
#9818=VERTEX_POINT ( 'NONE', #10151 ) ;
#9820=VERTEX_POINT ( 'NONE', #15941 ) ;
#9822=EDGE_LOOP ( 'NONE', ( #964, #7200, #8758, #15631 ) ) ;
#9825=CIRCLE ( 'NONE', #2251, 1.500000000000000444 ) ;
#9826=CARTESIAN_POINT ( 'NONE',  ( 1.399738696879940791, -77.73322974357483872, -4.330127018922189208 ) ) ;
#9828=ORIENTED_EDGE ( 'NONE', *, *, #9542, .F. ) ;
#9829=ADVANCED_FACE ( 'NONE', ( #17478 ), #15652, .F. ) ;
#9830=EDGE_CURVE ( 'NONE', #11150, #10784, #341, .T. ) ;
#9831=CARTESIAN_POINT ( 'NONE',  ( -76.66445292623467367, -32.41017715895461038, 12.99038105676661736 ) ) ;
#9832=FACE_OUTER_BOUND ( 'NONE', #13372, .T. ) ;
#9833=DIRECTION ( 'NONE',  ( 0.000000000000000000, 0.000000000000000000, 1.000000000000000000 ) ) ;
#9835=ORIENTED_EDGE ( 'NONE', *, *, #9030, .F. ) ;
#9836=DIRECTION ( 'NONE',  ( 0.000000000000000000, 0.000000000000000000, 1.000000000000000000 ) ) ;
#9837=ORIENTED_EDGE ( 'NONE', *, *, #683, .T. ) ;
#9838=DIRECTION ( 'NONE',  ( -0.1566598588826321192, 0.9876526153536342445, 7.798540720466730171E-17 ) ) ;
#9839=ORIENTED_EDGE ( 'NONE', *, *, #15991, .F. ) ;
#9840=EDGE_CURVE ( 'NONE', #859, #3849, #5504, .T. ) ;
#9841=VECTOR ( 'NONE', #4879, 1000.000000000000000 ) ;
#9843=ORIENTED_EDGE ( 'NONE', *, *, #8817, .F. ) ;
#9844=DIRECTION ( 'NONE',  ( 0.000000000000000000, 0.000000000000000000, 1.000000000000000000 ) ) ;
#9847=LINE ( 'NONE', #9768, #4577 ) ;
#9849=DIRECTION ( 'NONE',  ( -0.1566598588826321192, 0.9876526153536342445, 7.798540720466730171E-17 ) ) ;
#9850=CIRCLE ( 'NONE', #8926, 1.500000000000000444 ) ;
#9852=EDGE_CURVE ( 'NONE', #11472, #13816, #8743, .T. ) ;
#9853=FACE_BOUND ( 'NONE', #9021, .T. ) ;
#9854=EDGE_CURVE ( 'NONE', #16090, #15832, #2769, .T. ) ;
#9855=CYLINDRICAL_SURFACE ( 'NONE', #4432, 1.500000000000001554 ) ;
#9856=EDGE_CURVE ( 'NONE', #17593, #11470, #14859, .T. ) ;
#9857=VERTEX_POINT ( 'NONE', #16043 ) ;
#9858=CARTESIAN_POINT ( 'NONE',  ( -31.68662391746665463, -82.98133501614300656, 4.330127018922213189 ) ) ;
#9860=ORIENTED_EDGE ( 'NONE', *, *, #2510, .F. ) ;
#9861=ORIENTED_EDGE ( 'NONE', *, *, #16081, .F. ) ;
#9862=CARTESIAN_POINT ( 'NONE',  ( -48.97054468615519340, -85.72288254658904805, 1.424741226644455312E-14 ) ) ;
#9864=FACE_BOUND ( 'NONE', #17828, .T. ) ;
#9867=ORIENTED_EDGE ( 'NONE', *, *, #3615, .F. ) ;
#9868=EDGE_LOOP ( 'NONE', ( #13108, #11358 ) ) ;
#9869=CYLINDRICAL_SURFACE ( 'NONE', #5296, 1.500000000000001554 ) ;
#9870=AXIS2_PLACEMENT_3D ( 'NONE', #14494, #1520, #7311 ) ;
#9871=CARTESIAN_POINT ( 'NONE',  ( -32.22008523532134205, -25.36048350923618955, -4.330127018922181215 ) ) ;
#9872=DIRECTION ( 'NONE',  ( -0.1566598588826321192, 0.9876526153536342445, 7.798540720466730171E-17 ) ) ;
#9873=CYLINDRICAL_SURFACE ( 'NONE', #14504, 1.500000000000001554 ) ;
#9876=ORIENTED_EDGE ( 'NONE', *, *, #18283, .T. ) ;
#9879=EDGE_CURVE ( 'NONE', #2139, #5465, #1561, .T. ) ;
#9880=ORIENTED_EDGE ( 'NONE', *, *, #4965, .F. ) ;
#9884=CARTESIAN_POINT ( 'NONE',  ( -56.37793930130741415, -86.89783148820879433, -21.65063509461098690 ) ) ;
#9885=DIRECTION ( 'NONE',  ( -0.9876526153536341335, -0.1566598588826327021, 0.000000000000000000 ) ) ;
#9887=CIRCLE ( 'NONE', #3836, 1.500000000000000888 ) ;
#9888=CIRCLE ( 'NONE', #1723, 1.500000000000000888 ) ;
#9889=DIRECTION ( 'NONE',  ( -0.1566598588826321192, 0.9876526153536342445, 7.798540720466731404E-17 ) ) ;
#9890=CARTESIAN_POINT ( 'NONE',  ( -10.98555400521827963, -21.99229654325962002, -12.99038105676658006 ) ) ;
#9891=ORIENTED_EDGE ( 'NONE', *, *, #18047, .T. ) ;
#9892=DIRECTION ( 'NONE',  ( -0.1566598588826321192, 0.9876526153536342445, 7.798540720466731404E-17 ) ) ;
#9895=VERTEX_POINT ( 'NONE', #5905 ) ;
#9898=EDGE_CURVE ( 'NONE', #11379, #18705, #8823, .T. ) ;
#9899=CIRCLE ( 'NONE', #11974, 1.500000000000000444 ) ;
#9900=ORIENTED_EDGE ( 'NONE', *, *, #17812, .T. ) ;
#9901=DIRECTION ( 'NONE',  ( -0.1566598588826321192, 0.9876526153536342445, 7.798540720466730171E-17 ) ) ;
#9902=AXIS2_PLACEMENT_3D ( 'NONE', #13297, #11864, #17703 ) ;
#9904=DIRECTION ( 'NONE',  ( -0.9876526153536336894, -0.1566598588826349503, 0.000000000000000000 ) ) ;
#9906=DIRECTION ( 'NONE',  ( 0.000000000000000000, 0.000000000000000000, 1.000000000000000000 ) ) ;
#9907=DIRECTION ( 'NONE',  ( -1.000000000000000000, 0.000000000000000000, 0.000000000000000000 ) ) ;
#9908=CYLINDRICAL_SURFACE ( 'NONE', #13844, 1.500000000000001554 ) ;
#9910=DIRECTION ( 'NONE',  ( -0.1566598588826321192, 0.9876526153536342445, 7.798540720466731404E-17 ) ) ;
#9911=CARTESIAN_POINT ( 'NONE',  ( -29.05277406831996245, -19.79558099693753093, -8.660254037844380193 ) ) ;
#9914=CARTESIAN_POINT ( 'NONE',  ( -17.69476899175320739, -17.99399261978727438, 1.926565525561698076E-14 ) ) ;
#9915=ORIENTED_EDGE ( 'NONE', *, *, #14727, .F. ) ;
#9916=CARTESIAN_POINT ( 'NONE',  ( -1.892327146095121204, -15.48743487766515337, 12.99038105676661026 ) ) ;
#9918=DIRECTION ( 'NONE',  ( 0.000000000000000000, 0.000000000000000000, 1.000000000000000000 ) ) ;
#9919=EDGE_LOOP ( 'NONE', ( #1717, #1650 ) ) ;
#9921=CARTESIAN_POINT ( 'NONE',  ( -8.516422466834198346, -21.60064689605303911, -8.660254037844380193 ) ) ;
#9922=ORIENTED_EDGE ( 'NONE', *, *, #9783, .T. ) ;
#9923=EDGE_LOOP ( 'NONE', ( #12433, #11354, #401, #2211 ) ) ;
#9924=CIRCLE ( 'NONE', #2952, 1.500000000000000000 ) ;
#9925=EDGE_CURVE ( 'NONE', #4082, #3282, #5811, .T. ) ;
#9926=DIRECTION ( 'NONE',  ( -0.1566598588826321747, 0.9876526153536343555, 0.000000000000000000 ) ) ;
#9928=DIRECTION ( 'NONE',  ( -0.1566598588826321192, 0.9876526153536342445, 7.798540720466730171E-17 ) ) ;
#9929=CIRCLE ( 'NONE', #11432, 1.499999999999999556 ) ;
#9930=CARTESIAN_POINT ( 'NONE',  ( -57.69469991357523497, -24.33871690453385384, 4.330127018922218518 ) ) ;
#9931=CARTESIAN_POINT ( 'NONE',  ( -65.10209452872746283, -25.51366584615358590, -8.660254037844380193 ) ) ;
#9932=ADVANCED_FACE ( 'NONE', ( #11291 ), #7246, .F. ) ;
#9935=AXIS2_PLACEMENT_3D ( 'NONE', #14040, #1089, #15272 ) ;
#9937=VECTOR ( 'NONE', #14584, 1000.000000000000000 ) ;
#9938=DIRECTION ( 'NONE',  ( -0.9876526153536336894, -0.1566598588826349503, 0.000000000000000000 ) ) ;
#9939=CYLINDRICAL_SURFACE ( 'NONE', #8727, 1.500000000000001554 ) ;
#9941=ORIENTED_EDGE ( 'NONE', *, *, #15550, .T. ) ;
#9942=EDGE_LOOP ( 'NONE', ( #11630, #8797 ) ) ;
#9943=DIRECTION ( 'NONE',  ( -0.1566598588826321192, 0.9876526153536342445, 7.798540720466730171E-17 ) ) ;
#9944=ORIENTED_EDGE ( 'NONE', *, *, #14379, .T. ) ;
#9945=VECTOR ( 'NONE', #3214, 1000.000000000000000 ) ;
#9946=EDGE_LOOP ( 'NONE', ( #2602, #6999 ) ) ;
#9947=EDGE_LOOP ( 'NONE', ( #13244, #1193 ) ) ;
#9948=DIRECTION ( 'NONE',  ( -0.1566598588826321747, 0.9876526153536343555, 0.000000000000000000 ) ) ;
#9949=CIRCLE ( 'NONE', #9046, 1.500000000000000444 ) ;
#9952=EDGE_CURVE ( 'NONE', #4233, #1545, #14902, .T. ) ;
#9953=VERTEX_POINT ( 'NONE', #4468 ) ;
#9958=AXIS2_PLACEMENT_3D ( 'NONE', #5662, #15978, #1402 ) ;
#9960=CARTESIAN_POINT ( 'NONE',  ( -63.78533391645962780, -88.07278042982854060, 8.660254037844412167 ) ) ;
#9961=AXIS2_PLACEMENT_3D ( 'NONE', #154, #7450, #5659 ) ;
#9962=AXIS2_PLACEMENT_3D ( 'NONE', #18116, #8326, #8133 ) ;
#9963=AXIS2_PLACEMENT_3D ( 'NONE', #18579, #5545, #15206 ) ;
#9964=DIRECTION ( 'NONE',  ( -0.9876526153536336894, -0.1566598588826349503, 0.000000000000000000 ) ) ;
#9965=CYLINDRICAL_SURFACE ( 'NONE', #12686, 1.500000000000001554 ) ;
#9966=DIRECTION ( 'NONE',  ( -0.1566598588826321192, 0.9876526153536342445, 7.798540720466730171E-17 ) ) ;
#9967=VERTEX_POINT ( 'NONE', #13528 ) ;
#9968=ORIENTED_EDGE ( 'NONE', *, *, #5442, .T. ) ;
#9969=ORIENTED_EDGE ( 'NONE', *, *, #6124, .T. ) ;
#9970=CIRCLE ( 'NONE', #17883, 1.499999999999999556 ) ;
#9972=DIRECTION ( 'NONE',  ( -0.9876526153536336894, -0.1566598588826349503, 0.000000000000000000 ) ) ;
#9973=CIRCLE ( 'NONE', #5127, 1.500000000000000888 ) ;
#9974=EDGE_LOOP ( 'NONE', ( #11448, #17174, #8618, #11040 ) ) ;
#9975=CIRCLE ( 'NONE', #1807, 1.500000000000000888 ) ;
#9976=ORIENTED_EDGE ( 'NONE', *, *, #7777, .F. ) ;
#9978=DIRECTION ( 'NONE',  ( -0.1566598588826321747, 0.9876526153536343555, 0.000000000000000000 ) ) ;
#9980=ADVANCED_FACE ( 'NONE', ( #7958 ), #578, .F. ) ;
#9981=ADVANCED_FACE ( 'NONE', ( #16415, #11906 ), #17750, .T. ) ;
#9982=CYLINDRICAL_SURFACE ( 'NONE', #11435, 144.0000000000000284 ) ;
#9984=EDGE_CURVE ( 'NONE', #893, #16941, #16106, .T. ) ;
#9985=AXIS2_PLACEMENT_3D ( 'NONE', #4512, #2996, #17259 ) ;
#9986=FACE_OUTER_BOUND ( 'NONE', #6517, .T. ) ;
#9987=AXIS2_PLACEMENT_3D ( 'NONE', #11562, #14139, #2852 ) ;
#9988=DIRECTION ( 'NONE',  ( -0.000000000000000000, -0.000000000000000000, -1.000000000000000000 ) ) ;
#9991=VERTEX_POINT ( 'NONE', #7687 ) ;
#9992=EDGE_LOOP ( 'NONE', ( #8188, #8845 ) ) ;
#9993=CYLINDRICAL_SURFACE ( 'NONE', #6930, 1.500000000000001554 ) ;
#9994=AXIS2_PLACEMENT_3D ( 'NONE', #11224, #11497, #14070 ) ;
#9995=CARTESIAN_POINT ( 'NONE',  ( -46.33669483700848701, -22.53712852738358663, -4.330127018922180326 ) ) ;
#9996=ORIENTED_EDGE ( 'NONE', *, *, #8342, .T. ) ;
#9997=CARTESIAN_POINT ( 'NONE',  ( -64.31879523431432233, -30.45192892292171294, 1.869203119972154228E-14 ) ) ;
#9998=VERTEX_POINT ( 'NONE', #18132 ) ;
#9999=CIRCLE ( 'NONE', #31, 1.500000000000000888 ) ;
#10000=CARTESIAN_POINT ( 'NONE',  ( -33.99103714508810725, -20.57888029135069985, 17.32050807568882078 ) ) ;
#10001=AXIS2_PLACEMENT_3D ( 'NONE', #15983, #14569, #2822 ) ;
#10002=DIRECTION ( 'NONE',  ( -0.1566598588826321192, 0.9876526153536342445, 7.798540720466730171E-17 ) ) ;
#10004=AXIS2_PLACEMENT_3D ( 'NONE', #11318, #1399, #16077 ) ;
#10005=DIRECTION ( 'NONE',  ( -0.1566598588826321747, 0.9876526153536343555, 0.000000000000000000 ) ) ;
#10007=VECTOR ( 'NONE', #12636, 1000.000000000000000 ) ;
#10008=EDGE_CURVE ( 'NONE', #18590, #4436, #9132, .T. ) ;
#10009=CARTESIAN_POINT ( 'NONE',  ( -66.25446545484369665, -88.46443007703511796, 21.65063509461101532 ) ) ;
#10010=DIRECTION ( 'NONE',  ( -0.1566598588826321192, 0.9876526153536342445, 7.798540720466730171E-17 ) ) ;
#10011=VECTOR ( 'NONE', #11430, 1000.000000000000000 ) ;
#10013=EDGE_LOOP ( 'NONE', ( #14493, #7575, #1728, #18208 ) ) ;
#10014=DIRECTION ( 'NONE',  ( -0.9876526153536341335, -0.1566598588826330907, 0.000000000000000000 ) ) ;
#10015=EDGE_CURVE ( 'NONE', #2063, #12573, #673, .T. ) ;
#10017=CARTESIAN_POINT ( 'NONE',  ( -29.05277406831996245, -19.79558099693753093, -17.32050807568878170 ) ) ;
#10018=VERTEX_POINT ( 'NONE', #1898 ) ;
#10019=AXIS2_PLACEMENT_3D ( 'NONE', #905, #16740, #15284 ) ;
#10020=LINE ( 'NONE', #15706, #11456 ) ;
#10023=AXIS2_PLACEMENT_3D ( 'NONE', #17113, #9721, #15286 ) ;
#10024=LINE ( 'NONE', #8334, #3356 ) ;
#10025=VECTOR ( 'NONE', #16584, 1000.000000000000000 ) ;
#10026=AXIS2_PLACEMENT_3D ( 'NONE', #8702, #14483, #14397 ) ;
#10027=CYLINDRICAL_SURFACE ( 'NONE', #17928, 1.500000000000001554 ) ;
#10028=CARTESIAN_POINT ( 'NONE',  ( -29.05277406831996245, -19.79558099693753448, 1.908195823574487804E-14 ) ) ;
#10029=EDGE_LOOP ( 'NONE', ( #1949, #12922, #9922, #8206 ) ) ;
#10030=FACE_OUTER_BOUND ( 'NONE', #11776, .T. ) ;
#10032=AXIS2_PLACEMENT_3D ( 'NONE', #8339, #5593, #9565 ) ;
#10033=DIRECTION ( 'NONE',  ( -0.1566598588826321192, 0.9876526153536342445, 7.798540720466730171E-17 ) ) ;
#10034=CARTESIAN_POINT ( 'NONE',  ( -10.98555400521827607, -21.99229654325962002, 21.65063509461101177 ) ) ;
#10035=FACE_BOUND ( 'NONE', #3630, .T. ) ;
#10036=CIRCLE ( 'NONE', #16716, 1.500000000000000000 ) ;
#10041=DIRECTION ( 'NONE',  ( -0.9876526153536336894, -0.1566598588826349503, 0.000000000000000000 ) ) ;
#10042=ORIENTED_EDGE ( 'NONE', *, *, #16638, .F. ) ;
#10043=ORIENTED_EDGE ( 'NONE', *, *, #8382, .T. ) ;
#10045=EDGE_LOOP ( 'NONE', ( #8982, #17477, #12278, #4009 ) ) ;
#10046=CYLINDRICAL_SURFACE ( 'NONE', #8963, 1.500000000000001554 ) ;
#10047=AXIS2_PLACEMENT_3D ( 'NONE', #18713, #172, #17542 ) ;
#10048=ADVANCED_FACE ( 'NONE', ( #764 ), #4993, .F. ) ;
#10049=ORIENTED_EDGE ( 'NONE', *, *, #8465, .F. ) ;
#10050=FACE_BOUND ( 'NONE', #8583, .T. ) ;
#10051=LINE ( 'NONE', #11551, #16862 ) ;
#10053=EDGE_LOOP ( 'NONE', ( #12894, #13726, #4350, #2384 ) ) ;
#10055=ORIENTED_EDGE ( 'NONE', *, *, #10944, .F. ) ;
#10057=CARTESIAN_POINT ( 'NONE',  ( -9.464440072009985272, -79.45648819128378193, 17.32050807568880657 ) ) ;
#10058=CIRCLE ( 'NONE', #7612, 1.500000000000000888 ) ;
#10059=DIRECTION ( 'NONE',  ( -0.9876526153536341335, -0.1566598588826327021, 0.000000000000000000 ) ) ;
#10060=DIRECTION ( 'NONE',  ( -0.1566598588826321192, 0.9876526153536342445, 7.798540720466731404E-17 ) ) ;
#10061=CARTESIAN_POINT ( 'NONE',  ( -29.05277406831996245, -19.79558099693753448, 1.908195823574487804E-14 ) ) ;
#10064=EDGE_LOOP ( 'NONE', ( #9795, #13755 ) ) ;
#10065=ADVANCED_FACE ( 'NONE', ( #10770 ), #13438, .F. ) ;
#10066=ORIENTED_EDGE ( 'NONE', *, *, #12856, .F. ) ;
#10068=DIRECTION ( 'NONE',  ( -0.1566598588826321192, 0.9876526153536342445, 7.798540720466730171E-17 ) ) ;
#10069=FACE_BOUND ( 'NONE', #15397, .T. ) ;
#10070=FACE_OUTER_BOUND ( 'NONE', #10165, .T. ) ;
#10072=DIRECTION ( 'NONE',  ( -0.9876526153536336894, -0.1566598588826349503, 0.000000000000000000 ) ) ;
#10073=DIRECTION ( 'NONE',  ( -0.1566598588826321192, 0.9876526153536342445, 7.798540720466730171E-17 ) ) ;
#10078=DIRECTION ( 'NONE',  ( -0.1566598588826321192, 0.9876526153536342445, 7.798540720466731404E-17 ) ) ;
#10079=DIRECTION ( 'NONE',  ( -0.1566598588826321747, 0.9876526153536343555, 0.000000000000000000 ) ) ;
#10082=EDGE_CURVE ( 'NONE', #3359, #7684, #3659, .T. ) ;
#10084=ORIENTED_EDGE ( 'NONE', *, *, #11096, .T. ) ;
#10085=CIRCLE ( 'NONE', #4640, 1.500000000000001332 ) ;
#10086=CARTESIAN_POINT ( 'NONE',  ( -20.16390053013728334, -18.38564226699384818, -12.99038105676658006 ) ) ;
#10087=EDGE_CURVE ( 'NONE', #9184, #13174, #4287, .T. ) ;
#10088=DIRECTION ( 'NONE',  ( 1.000000000000000000, 0.000000000000000000, 0.000000000000000000 ) ) ;
#10090=FACE_OUTER_BOUND ( 'NONE', #4769, .T. ) ;
#10092=EDGE_LOOP ( 'NONE', ( #7795, #5014 ) ) ;
#10094=CIRCLE ( 'NONE', #1931, 1.500000000000000888 ) ;
#10095=DIRECTION ( 'NONE',  ( -0.9876526153536341335, -0.1566598588826327021, 0.000000000000000000 ) ) ;
#10097=CYLINDRICAL_SURFACE ( 'NONE', #14806, 1.500000000000001554 ) ;
#10099=DIRECTION ( 'NONE',  ( -0.9876526153536341335, -0.1566598588826327021, 0.000000000000000000 ) ) ;
#10100=LINE ( 'NONE', #1322, #17161 ) ;
#10102=EDGE_LOOP ( 'NONE', ( #11758, #3377, #13984, #12758 ) ) ;
#10103=CARTESIAN_POINT ( 'NONE',  ( -30.73860631229088725, -25.12549372091224598, 21.65063509461101887 ) ) ;
#10104=EDGE_LOOP ( 'NONE', ( #327, #672, #3431, #17260 ) ) ;
#10105=CARTESIAN_POINT ( 'NONE',  ( -29.25712738926043244, -24.89050393258829175, 12.99038105676661736 ) ) ;
#10106=ORIENTED_EDGE ( 'NONE', *, *, #16598, .T. ) ;
#10107=ORIENTED_EDGE ( 'NONE', *, *, #11352, .T. ) ;
#10108=FACE_OUTER_BOUND ( 'NONE', #11249, .T. ) ;
#10109=DIRECTION ( 'NONE',  ( -0.9876526153536341335, -0.1566598588826327021, 0.000000000000000000 ) ) ;
#10110=ORIENTED_EDGE ( 'NONE', *, *, #13501, .F. ) ;
#10111=ADVANCED_FACE ( 'NONE', ( #6932 ), #12669, .F. ) ;
#10112=EDGE_CURVE ( 'NONE', #13905, #3440, #7931, .T. ) ;
#10113=CARTESIAN_POINT ( 'NONE',  ( -55.42992169613163611, -29.04199019297804085, -12.99038105676658006 ) ) ;
#10115=FACE_OUTER_BOUND ( 'NONE', #632, .T. ) ;
#10116=VERTEX_POINT ( 'NONE', #9930 ) ;
#10117=DIRECTION ( 'NONE',  ( -0.9876526153536336894, -0.1566598588826349503, 0.000000000000000000 ) ) ;
#10118=LINE ( 'NONE', #4616, #14586 ) ;
#10119=DIRECTION ( 'NONE',  ( -0.1566598588826321747, 0.9876526153536343555, 0.000000000000000000 ) ) ;
#10120=DIRECTION ( 'NONE',  ( -0.1566598588826321192, 0.9876526153536342445, 7.798540720466730171E-17 ) ) ;
#10121=EDGE_LOOP ( 'NONE', ( #11691, #3134, #6215, #1888 ) ) ;
#10122=CARTESIAN_POINT ( 'NONE',  ( -10.94591899504043830, -79.69147797960773971, 8.660254037844412167 ) ) ;
#10123=CARTESIAN_POINT ( 'NONE',  ( -63.82496892663746735, -30.37359899348040315, 4.330127018922217630 ) ) ;
#10124=DIRECTION ( 'NONE',  ( -0.1566598588826321192, 0.9876526153536342445, 7.798540720466731404E-17 ) ) ;
#10127=VERTEX_POINT ( 'NONE', #10968 ) ;
#10128=CARTESIAN_POINT ( 'NONE',  ( -6.047290928450125946, -21.20899724884646531, -21.65063509461098334 ) ) ;
#10129=ORIENTED_EDGE ( 'NONE', *, *, #15869, .F. ) ;
#10130=LINE ( 'NONE', #8843, #18392 ) ;
#10131=ORIENTED_EDGE ( 'NONE', *, *, #13938, .F. ) ;
#10132=CARTESIAN_POINT ( 'NONE',  ( -15.92381708198643153, -22.77559583767277473, 12.99038105676661381 ) ) ;
#10134=DIRECTION ( 'NONE',  ( 0.000000000000000000, 0.000000000000000000, 1.000000000000000000 ) ) ;
#10135=ADVANCED_FACE ( 'NONE', ( #4143 ), #17078, .F. ) ;
#10136=DIRECTION ( 'NONE',  ( -0.1566598588826321192, 0.9876526153536342445, 7.798540720466731404E-17 ) ) ;
#10137=AXIS2_PLACEMENT_3D ( 'NONE', #5456, #12458, #7085 ) ;
#10138=LINE ( 'NONE', #2934, #2981 ) ;
#10139=EDGE_LOOP ( 'NONE', ( #5517, #6119 ) ) ;
#10140=EDGE_CURVE ( 'NONE', #3470, #4130, #3759, .T. ) ;
#10143=CARTESIAN_POINT ( 'NONE',  ( 0.000000000000000000, 0.000000000000000000, -30.00000000000000000 ) ) ;
#10144=CYLINDRICAL_SURFACE ( 'NONE', #16347, 1.500000000000001554 ) ;
#10145=DIRECTION ( 'NONE',  ( -0.9876526153536336894, -0.1566598588826349503, 0.000000000000000000 ) ) ;
#10146=CARTESIAN_POINT ( 'NONE',  ( -78.43540483600145308, -27.62857394106911357, -8.660254037844380193 ) ) ;
#10147=AXIS2_PLACEMENT_3D ( 'NONE', #5140, #15273, #8282 ) ;
#10148=ORIENTED_EDGE ( 'NONE', *, *, #2033, .F. ) ;
#10149=EDGE_LOOP ( 'NONE', ( #5370, #18325 ) ) ;
#10150=VERTEX_POINT ( 'NONE', #2464 ) ;
#10151=CARTESIAN_POINT ( 'NONE',  ( -4.565812005419673802, -20.97400746052251108, -12.99038105676658006 ) ) ;
#10158=AXIS2_PLACEMENT_3D ( 'NONE', #6648, #11066, #15250 ) ;
#10160=LINE ( 'NONE', #17594, #6725 ) ;
#10161=EDGE_CURVE ( 'NONE', #15907, #491, #3363, .T. ) ;
#10165=EDGE_LOOP ( 'NONE', ( #13480, #12153, #4739, #5987 ) ) ;
#10166=ORIENTED_EDGE ( 'NONE', *, *, #7613, .T. ) ;
#10167=LINE ( 'NONE', #12917, #12650 ) ;
#10168=AXIS2_PLACEMENT_3D ( 'NONE', #13646, #12308, #12212 ) ;
#10169=DIRECTION ( 'NONE',  ( -0.1566598588826321192, 0.9876526153536342445, 7.798540720466731404E-17 ) ) ;
#10171=VERTEX_POINT ( 'NONE', #5399 ) ;
#10172=DIRECTION ( 'NONE',  ( -0.1566598588826321192, 0.9876526153536342445, 7.798540720466730171E-17 ) ) ;
#10173=EDGE_CURVE ( 'NONE', #10331, #14323, #10327, .T. ) ;
#10174=AXIS2_PLACEMENT_3D ( 'NONE', #7574, #13237, #376 ) ;
#10175=EDGE_CURVE ( 'NONE', #12283, #5678, #2163, .T. ) ;
#10176=DIRECTION ( 'NONE',  ( 0.000000000000000000, 0.000000000000000000, 1.000000000000000000 ) ) ;
#10177=EDGE_CURVE ( 'NONE', #12874, #14890, #9847, .T. ) ;
#10178=CIRCLE ( 'NONE', #5961, 1.499999999999999556 ) ;
#10179=DIRECTION ( 'NONE',  ( -0.1566598588826321192, 0.9876526153536342445, 7.798540720466731404E-17 ) ) ;
#10180=( NAMED_UNIT ( * ) PLANE_ANGLE_UNIT ( ) SI_UNIT ( $, .RADIAN. ) );
#10182=ADVANCED_FACE ( 'NONE', ( #8430 ), #2550, .F. ) ;
#10184=AXIS2_PLACEMENT_3D ( 'NONE', #18293, #5263, #15497 ) ;
#10185=DIRECTION ( 'NONE',  ( -0.1566598588826321192, 0.9876526153536342445, 7.798540720466730171E-17 ) ) ;
#10188=CARTESIAN_POINT ( 'NONE',  ( -73.70149508017377116, -31.94019758230671258, 21.65063509461101887 ) ) ;
#10189=ORIENTED_EDGE ( 'NONE', *, *, #10112, .T. ) ;
#10191=AXIS2_PLACEMENT_3D ( 'NONE', #17814, #10476, #14751 ) ;
#10193=ORIENTED_EDGE ( 'NONE', *, *, #12296, .F. ) ;
#10194=AXIS2_PLACEMENT_3D ( 'NONE', #10646, #3863, #14909 ) ;
#10195=ORIENTED_EDGE ( 'NONE', *, *, #17862, .F. ) ;
#10196=EDGE_LOOP ( 'NONE', ( #16591, #7672 ) ) ;
#10197=ORIENTED_EDGE ( 'NONE', *, *, #15308, .F. ) ;
#10199=CARTESIAN_POINT ( 'NONE',  ( -2.000000000000000000, 0.000000000000000000, 24.99999999999999289 ) ) ;
#10200=CIRCLE ( 'NONE', #4455, 1.499999999999999556 ) ;
#10201=EDGE_LOOP ( 'NONE', ( #8035, #7382, #15586, #680 ) ) ;
#10202=ADVANCED_FACE ( 'NONE', ( #1155 ), #14207, .F. ) ;
#10203=CARTESIAN_POINT ( 'NONE',  ( -11.97320662057189899, -22.14895640214223960, 8.660254037844413944 ) ) ;
#10206=DIRECTION ( 'NONE',  ( -0.1566598588826321192, 0.9876526153536342445, 7.798540720466730171E-17 ) ) ;
#10207=CARTESIAN_POINT ( 'NONE',  ( -3.044698072211382112, -78.43819910854666944, 1.443110928631665584E-14 ) ) ;
#10208=AXIS2_PLACEMENT_3D ( 'NONE', #1928, #13468, #6208 ) ;
#10209=EDGE_CURVE ( 'NONE', #4467, #93, #1865, .T. ) ;
#10211=ORIENTED_EDGE ( 'NONE', *, *, #11227, .T. ) ;
#10214=EDGE_CURVE ( 'NONE', #12208, #13656, #3974, .T. ) ;
#10215=EDGE_CURVE ( 'NONE', #4978, #1633, #10118, .T. ) ;
#10216=CYLINDRICAL_SURFACE ( 'NONE', #1178, 1.500000000000001554 ) ;
#10218=PRODUCT_DEFINITION_FORMATION_WITH_SPECIFIED_SOURCE ( 'ANY', '', #2590, .NOT_KNOWN. ) ;
#10219=CARTESIAN_POINT ( 'NONE',  ( -28.26947477390680774, -24.73384407370567217, 17.32050807568881723 ) ) ;
#10220=ORIENTED_EDGE ( 'NONE', *, *, #15412, .F. ) ;
#10221=ORIENTED_EDGE ( 'NONE', *, *, #8342, .F. ) ;
#10223=ORIENTED_EDGE ( 'NONE', *, *, #5923, .F. ) ;
#10225=CARTESIAN_POINT ( 'NONE',  ( -6.830590222863280658, -16.27073417207831696, -4.330127018922183879 ) ) ;
#10227=ORIENTED_EDGE ( 'NONE', *, *, #15847, .F. ) ;
#10228=FACE_BOUND ( 'NONE', #12556, .T. ) ;
#10229=VERTEX_POINT ( 'NONE', #11799 ) ;
#10231=DIRECTION ( 'NONE',  ( -0.1566598588826321747, 0.9876526153536343555, 0.000000000000000000 ) ) ;
#10233=CARTESIAN_POINT ( 'NONE',  ( -11.97320662057189899, -22.14895640214223960, -8.660254037844380193 ) ) ;
#10234=CARTESIAN_POINT ( 'NONE',  ( -27.57129514528951120, -19.56059120861358380, -17.32050807568878170 ) ) ;
#10235=ORIENTED_EDGE ( 'NONE', *, *, #2532, .T. ) ;
#10236=ADVANCED_FACE ( 'NONE', ( #2047 ), #11617, .F. ) ;
#10237=ORIENTED_EDGE ( 'NONE', *, *, #16457, .F. ) ;
#10238=EDGE_CURVE ( 'NONE', #8901, #4830, #8969, .T. ) ;
#10239=CARTESIAN_POINT ( 'NONE',  ( -71.23236354178970942, -31.54854793510013877, 8.660254037844417496 ) ) ;
#10240=LINE ( 'NONE', #17826, #2433 ) ;
#10242=AXIS2_PLACEMENT_3D ( 'NONE', #92, #1613, #7475 ) ;
#10243=CARTESIAN_POINT ( 'NONE',  ( -67.77557938805200877, -31.00023842901093118, 17.32050807568881723 ) ) ;
#10244=EDGE_CURVE ( 'NONE', #2879, #1265, #9429, .T. ) ;
#10245=VECTOR ( 'NONE', #8180, 1000.000000000000000 ) ;
#10246=ORIENTED_EDGE ( 'NONE', *, *, #15525, .T. ) ;
#10247=VERTEX_POINT ( 'NONE', #5790 ) ;
#10248=VERTEX_POINT ( 'NONE', #1610 ) ;
#10250=ORIENTED_EDGE ( 'NONE', *, *, #16123, .T. ) ;
#10251=FACE_BOUND ( 'NONE', #642, .T. ) ;
#10253=DIRECTION ( 'NONE',  ( -0.1566598588826321192, 0.9876526153536342445, 7.798540720466730171E-17 ) ) ;
#10254=EDGE_LOOP ( 'NONE', ( #14866, #8029, #9422, #10319 ) ) ;
#10255=CARTESIAN_POINT ( 'NONE',  ( -10.98555400521827963, -21.99229654325962002, -21.65063509461098334 ) ) ;
#10256=CIRCLE ( 'NONE', #6946, 1.499999999999999556 ) ;
#10257=VERTEX_POINT ( 'NONE', #14487 ) ;
#10258=CIRCLE ( 'NONE', #4814, 1.500000000000000888 ) ;
#10259=AXIS2_PLACEMENT_3D ( 'NONE', #11984, #17827, #11710 ) ;
#10261=DIRECTION ( 'NONE',  ( -0.9876526153536341335, -0.1566598588826327021, 0.000000000000000000 ) ) ;
#10266=EDGE_LOOP ( 'NONE', ( #7417, #6705, #18368, #18268 ) ) ;
#10267=EDGE_LOOP ( 'NONE', ( #16945, #14984 ) ) ;
#10269=ADVANCED_FACE ( 'NONE', ( #17272 ), #7121, .F. ) ;
#10270=DIRECTION ( 'NONE',  ( -0.1566598588826321192, 0.9876526153536342445, 7.798540720466730171E-17 ) ) ;
#10271=CARTESIAN_POINT ( 'NONE',  ( -38.92930022185626626, -21.36217958576384390, -17.32050807568878170 ) ) ;
#10272=AXIS2_PLACEMENT_3D ( 'NONE', #5167, #10930, #3721 ) ;
#10273=CIRCLE ( 'NONE', #2959, 1.500000000000000000 ) ;
#10275=ORIENTED_EDGE ( 'NONE', *, *, #5975, .T. ) ;
#10276=CARTESIAN_POINT ( 'NONE',  ( -79.30363509306917535, 32.43333333333333002, 92.77853496600735639 ) ) ;
#10278=CIRCLE ( 'NONE', #2112, 1.500000000000000888 ) ;
#10279=DIRECTION ( 'NONE',  ( -0.9876526153536336894, -0.1566598588826349503, 0.000000000000000000 ) ) ;
#10280=AXIS2_PLACEMENT_3D ( 'NONE', #9306, #15190, #13948 ) ;
#10282=CYLINDRICAL_SURFACE ( 'NONE', #17217, 2.000000000000000000 ) ;
#10284=CIRCLE ( 'NONE', #14538, 2.500000000000002220 ) ;
#10285=CARTESIAN_POINT ( 'NONE',  ( -6.007655918272284623, -78.90817868519457079, -8.660254037844385522 ) ) ;
#10286=CIRCLE ( 'NONE', #7568, 1.500000000000001332 ) ;
#10287=LINE ( 'NONE', #1592, #8375 ) ;
#10288=CYLINDRICAL_SURFACE ( 'NONE', #10433, 1.500000000000001554 ) ;
#10289=FACE_OUTER_BOUND ( 'NONE', #13591, .T. ) ;
#10290=VERTEX_POINT ( 'NONE', #12866 ) ;
#10294=CIRCLE ( 'NONE', #4837, 1.500000000000000888 ) ;
#10295=EDGE_CURVE ( 'NONE', #8550, #8304, #17361, .T. ) ;
#10296=EDGE_CURVE ( 'NONE', #16997, #4463, #13369, .T. ) ;
#10297=DIRECTION ( 'NONE',  ( -0.1566598588826321192, 0.9876526153536342445, 7.798540720466730171E-17 ) ) ;
#10298=AXIS2_PLACEMENT_3D ( 'NONE', #7853, #13616, #14617 ) ;
#10299=VERTEX_POINT ( 'NONE', #7472 ) ;
#10300=EDGE_CURVE ( 'NONE', #11204, #16695, #11433, .T. ) ;
#10302=AXIS2_PLACEMENT_3D ( 'NONE', #8398, #8502, #12841 ) ;
#10303=LINE ( 'NONE', #11797, #15791 ) ;
#10304=DIRECTION ( 'NONE',  ( 1.000000000000000000, 0.000000000000000000, 0.000000000000000000 ) ) ;
#10307=CYLINDRICAL_SURFACE ( 'NONE', #11440, 1.500000000000001554 ) ;
#10308=AXIS2_PLACEMENT_3D ( 'NONE', #14080, #8400, #15800 ) ;
#10309=DIRECTION ( 'NONE',  ( -0.9876526153536336894, -0.1566598588826349503, 0.000000000000000000 ) ) ;
#10311=DIRECTION ( 'NONE',  ( -0.1566598588826321192, 0.9876526153536342445, 7.798540720466730171E-17 ) ) ;
#10312=DIRECTION ( 'NONE',  ( -0.1566598588826321747, 0.9876526153536343555, 0.000000000000000000 ) ) ;
#10314=EDGE_CURVE ( 'NONE', #10907, #3313, #15188, .T. ) ;
#10315=ADVANCED_FACE ( 'NONE', ( #4346 ), #89, .F. ) ;
#10316=EDGE_LOOP ( 'NONE', ( #14677, #474 ) ) ;
#10317=VECTOR ( 'NONE', #10553, 1000.000000000000000 ) ;
#10318=ADVANCED_FACE ( 'NONE', ( #14583 ), #11704, .F. ) ;
#10319=ORIENTED_EDGE ( 'NONE', *, *, #9011, .F. ) ;
#10320=DIRECTION ( 'NONE',  ( 0.000000000000000000, 0.000000000000000000, 1.000000000000000000 ) ) ;
#10321=EDGE_LOOP ( 'NONE', ( #15581, #9085 ) ) ;
#10322=ORIENTED_EDGE ( 'NONE', *, *, #2532, .F. ) ;
#10324=FACE_OUTER_BOUND ( 'NONE', #1657, .T. ) ;
#10325=DIRECTION ( 'NONE',  ( -0.9876526153536336894, -0.1566598588826349503, 0.000000000000000000 ) ) ;
#10326=VERTEX_POINT ( 'NONE', #4525 ) ;
#10327=CIRCLE ( 'NONE', #2482, 1.500000000000001332 ) ;
#10328=CARTESIAN_POINT ( 'NONE',  ( -40.61513246582718040, -26.69209230973856251, 21.65063509461101887 ) ) ;
#10329=VERTEX_POINT ( 'NONE', #17647 ) ;
#10330=AXIS2_PLACEMENT_3D ( 'NONE', #16150, #1729, #7517 ) ;
#10331=VERTEX_POINT ( 'NONE', #16103 ) ;
#10332=DIRECTION ( 'NONE',  ( -0.1566598588826321747, 0.9876526153536343555, 0.000000000000000000 ) ) ;
#10333=DIRECTION ( 'NONE',  ( -0.9876526153536341335, -0.1566598588826327021, 0.000000000000000000 ) ) ;
#10334=CARTESIAN_POINT ( 'NONE',  ( -35.67686938905902849, -25.90879301532540779, 4.330127018922217630 ) ) ;
#10335=AXIS2_PLACEMENT_3D ( 'NONE', #1686, #13233, #10391 ) ;
#10336=ORIENTED_EDGE ( 'NONE', *, *, #7448, .T. ) ;
#10338=ORIENTED_EDGE ( 'NONE', *, *, #3193, .T. ) ;
#10340=VERTEX_POINT ( 'NONE', #4251 ) ;
#10341=VERTEX_POINT ( 'NONE', #3100 ) ;
#10342=FACE_BOUND ( 'NONE', #2677, .T. ) ;
#10343=ADVANCED_FACE ( 'NONE', ( #10030 ), #14669, .F. ) ;
#10344=CIRCLE ( 'NONE', #14305, 20.00000000000001066 ) ;
#10348=CARTESIAN_POINT ( 'NONE',  ( -54.44226908077801852, -28.88533033409541062, -17.32050807568878170 ) ) ;
#10349=ORIENTED_EDGE ( 'NONE', *, *, #15638, .F. ) ;
#10351=EDGE_CURVE ( 'NONE', #14703, #16242, #9075, .T. ) ;
#10352=VERTEX_POINT ( 'NONE', #13504 ) ;
#10353=CARTESIAN_POINT ( 'NONE',  ( -19.87442754340095519, -23.40223527320329922, -17.32050807568878170 ) ) ;
#10356=DIRECTION ( 'NONE',  ( -0.1566598588826321192, 0.9876526153536342445, 7.798540720466731404E-17 ) ) ;
#10357=LINE ( 'NONE', #8858, #10538 ) ;
#10358=CARTESIAN_POINT ( 'NONE',  ( 8.807133312032172867, -76.55828080195509244, 17.32050807568880657 ) ) ;
#10361=DIRECTION ( 'NONE',  ( -0.1566598588826321192, 0.9876526153536342445, 7.798540720466730171E-17 ) ) ;
#10362=CARTESIAN_POINT ( 'NONE',  ( -20.82244514857674389, -81.25807656843404914, -17.32050807568878525 ) ) ;
#10364=CIRCLE ( 'NONE', #12796, 1.500000000000001332 ) ;
#10365=ORIENTED_EDGE ( 'NONE', *, *, #10987, .F. ) ;
#10367=FACE_BOUND ( 'NONE', #11637, .T. ) ;
#10368=CARTESIAN_POINT ( 'NONE',  ( -27.73601345605214519, -82.35469558061247142, -17.32050807568878525 ) ) ;
#10369=ADVANCED_FACE ( 'NONE', ( #16275 ), #17926, .F. ) ;
#10371=DIRECTION ( 'NONE',  ( -0.1566598588826321192, 0.9876526153536342445, 7.798540720466730171E-17 ) ) ;
#10372=VERTEX_POINT ( 'NONE', #5073 ) ;
#10373=AXIS2_PLACEMENT_3D ( 'NONE', #3756, #15444, #2463 ) ;
#10375=CARTESIAN_POINT ( 'NONE',  ( -56.21322099054476240, -24.10372711620991382, 21.65063509461102242 ) ) ;
#10376=EDGE_CURVE ( 'NONE', #7723, #16742, #7745, .T. ) ;
#10378=DIRECTION ( 'NONE',  ( -0.9876526153536336894, -0.1566598588826349503, 0.000000000000000000 ) ) ;
#10379=ORIENTED_EDGE ( 'NONE', *, *, #7689, .F. ) ;
#10380=ORIENTED_EDGE ( 'NONE', *, *, #8729, .F. ) ;
#10381=CARTESIAN_POINT ( 'NONE',  ( -8.476787456656362352, -79.29982833240116236, 12.99038105676660848 ) ) ;
#10382=VERTEX_POINT ( 'NONE', #16673 ) ;
#10383=ORIENTED_EDGE ( 'NONE', *, *, #9492, .F. ) ;
#10384=CIRCLE ( 'NONE', #13399, 1.500000000000001332 ) ;
#10385=LINE ( 'NONE', #3096, #11088 ) ;
#10388=ADVANCED_FACE ( 'NONE', ( #18013 ), #13697, .F. ) ;
#10391=DIRECTION ( 'NONE',  ( -0.9876526153536336894, -0.1566598588826349503, 0.000000000000000000 ) ) ;
#10393=CARTESIAN_POINT ( 'NONE',  ( -74.48479437458692587, -27.00193450553860330, 21.65063509461101887 ) ) ;
#10394=ORIENTED_EDGE ( 'NONE', *, *, #12968, .F. ) ;
#10395=CARTESIAN_POINT ( 'NONE',  ( -49.01017969633304006, -28.02370111024093191, -21.65063509461098334 ) ) ;
#10397=DIRECTION ( 'NONE',  ( -0.1566598588826321747, 0.9876526153536343555, 0.000000000000000000 ) ) ;
#10399=ORIENTED_EDGE ( 'NONE', *, *, #7642, .T. ) ;
#10400=CARTESIAN_POINT ( 'NONE',  ( -14.93616446663280328, -22.61893597879013740, 8.660254037844413944 ) ) ;
#10402=ORIENTED_EDGE ( 'NONE', *, *, #3899, .F. ) ;
#10403=CARTESIAN_POINT ( 'NONE',  ( -75.96627329761737712, -27.23692429386253266, -12.99038105676658006 ) ) ;
#10405=VERTEX_POINT ( 'NONE', #6346 ) ;
#10406=CARTESIAN_POINT ( 'NONE',  ( -71.02801022084922522, -26.45362499944937440, -12.99038105676658006 ) ) ;
#10407=EDGE_CURVE ( 'NONE', #450, #9967, #4894, .T. ) ;
#10408=ORIENTED_EDGE ( 'NONE', *, *, #16598, .F. ) ;
#10409=DIRECTION ( 'NONE',  ( -0.9876526153536336894, -0.1566598588826349503, 0.000000000000000000 ) ) ;
#10410=ORIENTED_EDGE ( 'NONE', *, *, #12264, .T. ) ;
#10412=EDGE_CURVE ( 'NONE', #1601, #13816, #7945, .T. ) ;
#10415=DIRECTION ( 'NONE',  ( -0.1566598588826321192, 0.9876526153536342445, 7.798540720466730171E-17 ) ) ;
#10416=EDGE_CURVE ( 'NONE', #6562, #12633, #10654, .T. ) ;
#10417=CARTESIAN_POINT ( 'NONE',  ( -30.53425299135042081, -20.03057078526148871, 17.32050807568881723 ) ) ;
#10419=AXIS2_PLACEMENT_3D ( 'NONE', #4734, #6185, #10518 ) ;
#10420=ORIENTED_EDGE ( 'NONE', *, *, #13715, .T. ) ;
#10421=EDGE_CURVE ( 'NONE', #13736, #12390, #18593, .T. ) ;
#10423=ORIENTED_EDGE ( 'NONE', *, *, #10984, .T. ) ;
#10424=DIRECTION ( 'NONE',  ( -0.1566598588826321747, 0.9876526153536343555, 0.000000000000000000 ) ) ;
#10425=FACE_OUTER_BOUND ( 'NONE', #4652, .T. ) ;
#10426=ORIENTED_EDGE ( 'NONE', *, *, #13629, .F. ) ;
#10428=ORIENTED_EDGE ( 'NONE', *, *, #16212, .T. ) ;
#10429=ORIENTED_EDGE ( 'NONE', *, *, #13123, .T. ) ;
#10430=EDGE_LOOP ( 'NONE', ( #2205, #7805 ) ) ;
#10431=DIRECTION ( 'NONE',  ( 1.000000000000000000, 0.000000000000000000, 0.000000000000000000 ) ) ;
#10432=ORIENTED_EDGE ( 'NONE', *, *, #16368, .T. ) ;
#10433=AXIS2_PLACEMENT_3D ( 'NONE', #13128, #74, #4329 ) ;
#10434=FACE_BOUND ( 'NONE', #12565, .T. ) ;
#10435=DIRECTION ( 'NONE',  ( -0.1566598588826321747, 0.9876526153536343555, 0.000000000000000000 ) ) ;
#10436=LINE ( 'NONE', #12217, #15203 ) ;
#10437=EDGE_LOOP ( 'NONE', ( #13222, #2002, #5965, #17410 ) ) ;
#10438=EDGE_CURVE ( 'NONE', #14662, #93, #11888, .T. ) ;
#10439=VERTEX_POINT ( 'NONE', #12269 ) ;
#10440=LINE ( 'NONE', #17875, #2475 ) ;
#10441=EDGE_LOOP ( 'NONE', ( #910, #7383, #5979, #13352 ) ) ;
#10442=DIRECTION ( 'NONE',  ( -2.887450008416415878E-16, -0.000000000000000000, -1.000000000000000000 ) ) ;
#10447=DIRECTION ( 'NONE',  ( 0.000000000000000000, 0.000000000000000000, 1.000000000000000000 ) ) ;
#10449=CARTESIAN_POINT ( 'NONE',  ( -69.25705831108246002, -31.23522821733487476, 17.32050807568881723 ) ) ;
#10450=VERTEX_POINT ( 'NONE', #15137 ) ;
#10451=ORIENTED_EDGE ( 'NONE', *, *, #12615, .T. ) ;
#10453=CARTESIAN_POINT ( 'NONE',  ( -62.79768130110601021, -87.91612057094592103, 21.65063509461101532 ) ) ;
#10454=DIRECTION ( 'NONE',  ( -0.1566598588826321192, 0.9876526153536342445, 7.798540720466730171E-17 ) ) ;
#10455=CARTESIAN_POINT ( 'NONE',  ( -33.99103714508810725, -20.57888029135069630, 8.660254037844417496 ) ) ;
#10456=EDGE_LOOP ( 'NONE', ( #4157, #14804 ) ) ;
#10458=CARTESIAN_POINT ( 'NONE',  ( -44.56574292724170760, -27.31873174526908699, 1.869203119972154228E-14 ) ) ;
#10459=CYLINDRICAL_SURFACE ( 'NONE', #16074, 1.500000000000001554 ) ;
#10461=EDGE_LOOP ( 'NONE', ( #9269, #16426 ) ) ;
#10462=AXIS2_PLACEMENT_3D ( 'NONE', #407, #17768, #4839 ) ;
#10463=CARTESIAN_POINT ( 'NONE',  ( 0.5768043922889515285, -15.09578523045857601, 1.387778780781445676E-14 ) ) ;
#10466=DIRECTION ( 'NONE',  ( -0.1566598588826321747, 0.9876526153536343555, 0.000000000000000000 ) ) ;
#10467=VERTEX_POINT ( 'NONE', #13416 ) ;
#10468=EDGE_LOOP ( 'NONE', ( #7086, #11807, #2971, #13157 ) ) ;
#10469=DIRECTION ( 'NONE',  ( -0.1566598588826321192, 0.9876526153536342445, 7.798540720466730171E-17 ) ) ;
#10470=VERTEX_POINT ( 'NONE', #6241 ) ;
#10471=AXIS2_PLACEMENT_3D ( 'NONE', #16676, #8128, #2621 ) ;
#10472=ORIENTED_EDGE ( 'NONE', *, *, #10087, .T. ) ;
#10474=ORIENTED_EDGE ( 'NONE', *, *, #12239, .F. ) ;
#10475=CIRCLE ( 'NONE', #2310, 1.500000000000001332 ) ;
#10476=DIRECTION ( 'NONE',  ( -0.1566598588826321747, 0.9876526153536343555, 0.000000000000000000 ) ) ;
#10477=FACE_OUTER_BOUND ( 'NONE', #2781, .T. ) ;
#10482=CARTESIAN_POINT ( 'NONE',  ( -13.25033222266188560, -17.28902325481542235, 21.65063509461101177 ) ) ;
#10485=CIRCLE ( 'NONE', #16249, 1.500000000000000000 ) ;
#10486=FACE_BOUND ( 'NONE', #15764, .T. ) ;
#10488=FACE_OUTER_BOUND ( 'NONE', #12125, .T. ) ;
#10489=ORIENTED_EDGE ( 'NONE', *, *, #5792, .T. ) ;
#10490=CIRCLE ( 'NONE', #12255, 1.500000000000001332 ) ;
#10491=FACE_OUTER_BOUND ( 'NONE', #17979, .T. ) ;
#10492=ORIENTED_EDGE ( 'NONE', *, *, #15162, .F. ) ;
#10493=VERTEX_POINT ( 'NONE', #16385 ) ;
#10494=DIRECTION ( 'NONE',  ( -0.9876526153536341335, -0.1566598588826327021, 0.000000000000000000 ) ) ;
#10495=ORIENTED_EDGE ( 'NONE', *, *, #5714, .T. ) ;
#10496=EDGE_CURVE ( 'NONE', #14458, #5860, #11256, .T. ) ;
#10497=CIRCLE ( 'NONE', #9604, 1.500000000000000444 ) ;
#10499=VECTOR ( 'NONE', #1481, 1000.000000000000114 ) ;
#10501=DIRECTION ( 'NONE',  ( -0.9876526153536336894, -0.1566598588826349503, 0.000000000000000000 ) ) ;
#10502=ORIENTED_EDGE ( 'NONE', *, *, #18443, .F. ) ;
#10503=CARTESIAN_POINT ( 'NONE',  ( -9.504075082187826595, -21.75730675493566579, -4.330127018922181215 ) ) ;
#10504=ADVANCED_FACE ( 'NONE', ( #9644 ), #6617, .F. ) ;
#10505=ORIENTED_EDGE ( 'NONE', *, *, #123, .F. ) ;
#10508=DIRECTION ( 'NONE',  ( -0.1566598588826321747, 0.9876526153536343555, 0.000000000000000000 ) ) ;
#10509=DIRECTION ( 'NONE',  ( 0.000000000000000000, 0.000000000000000000, 1.000000000000000000 ) ) ;
#10511=DIRECTION ( 'NONE',  ( -0.000000000000000000, -0.000000000000000000, -1.000000000000000000 ) ) ;
#10512=CARTESIAN_POINT ( 'NONE',  ( -34.15575545585074480, -83.37298466334958391, -8.660254037844385522 ) ) ;
#10514=ORIENTED_EDGE ( 'NONE', *, *, #18077, .F. ) ;
#10515=CIRCLE ( 'NONE', #5981, 1.499999999999999556 ) ;
#10516=DIRECTION ( 'NONE',  ( -0.000000000000000000, -0.000000000000000000, -1.000000000000000000 ) ) ;
#10517=VERTEX_POINT ( 'NONE', #1047 ) ;
#10518=DIRECTION ( 'NONE',  ( 0.000000000000000000, 0.000000000000000000, 1.000000000000000000 ) ) ;
#10521=VERTEX_POINT ( 'NONE', #3831 ) ;
#10522=DIRECTION ( 'NONE',  ( -0.1566598588826321192, 0.9876526153536342445, 7.798540720466730171E-17 ) ) ;
#10523=ORIENTED_EDGE ( 'NONE', *, *, #16346, .T. ) ;
#10525=FACE_OUTER_BOUND ( 'NONE', #10468, .T. ) ;
#10527=ADVANCED_FACE ( 'NONE', ( #2443 ), #5192, .F. ) ;
#10529=FACE_BOUND ( 'NONE', #14322, .T. ) ;
#10531=EDGE_CURVE ( 'NONE', #7400, #10171, #8553, .T. ) ;
#10532=ORIENTED_EDGE ( 'NONE', *, *, #1411, .F. ) ;
#10533=VERTEX_POINT ( 'NONE', #18606 ) ;
#10534=VECTOR ( 'NONE', #8075, 1000.000000000000000 ) ;
#10536=CARTESIAN_POINT ( 'NONE',  ( 0.4120860815263194254, -77.88988960245745830, -8.660254037844385522 ) ) ;
#10537=DIRECTION ( 'NONE',  ( 1.000000000000000000, 0.000000000000000000, 0.000000000000000000 ) ) ;
#10538=VECTOR ( 'NONE', #223, 1000.000000000000000 ) ;
#10539=CARTESIAN_POINT ( 'NONE',  ( -56.21322099054479082, -24.10372711620990316, -4.330127018922180326 ) ) ;
#10542=CARTESIAN_POINT ( 'NONE',  ( -63.78533391645962780, -88.07278042982852639, -17.32050807568878525 ) ) ;
#10543=CARTESIAN_POINT ( 'NONE',  ( -88.14047854185180597, 6.938893903907228378E-15, 30.00000000000000000 ) ) ;
#10545=EDGE_LOOP ( 'NONE', ( #5038, #15871 ) ) ;
#10546=DIRECTION ( 'NONE',  ( -0.1566598588826321192, 0.9876526153536342445, 7.798540720466730171E-17 ) ) ;
#10547=CARTESIAN_POINT ( 'NONE',  ( -62.79768130110601021, -87.91612057094590682, 4.330127018922213189 ) ) ;
#10550=ADVANCED_FACE ( 'NONE', ( #15318 ), #12478, .F. ) ;
#10552=VERTEX_POINT ( 'NONE', #18507 ) ;
#10553=DIRECTION ( 'NONE',  ( -0.1566598588826321192, 0.9876526153536342445, 7.798540720466730171E-17 ) ) ;
#10554=AXIS2_PLACEMENT_3D ( 'NONE', #262, #17444, #8710 ) ;
#10555=VECTOR ( 'NONE', #3401, 1000.000000000000000 ) ;
#10557=CARTESIAN_POINT ( 'NONE',  ( -24.31886431249228409, -24.10720463817513703, 12.99038105676661736 ) ) ;
#10558=DIRECTION ( 'NONE',  ( -0.1566598588826321192, 0.9876526153536342445, 7.798540720466730171E-17 ) ) ;
#10559=CARTESIAN_POINT ( 'NONE',  ( -54.89646037827694869, -86.66284169988485075, 21.65063509461101532 ) ) ;
#10560=CIRCLE ( 'NONE', #12979, 1.500000000000000000 ) ;
#10561=DIRECTION ( 'NONE',  ( -0.9876526153536336894, -0.1566598588826349503, 0.000000000000000000 ) ) ;
#10562=VECTOR ( 'NONE', #6558, 1000.000000000000000 ) ;
#10563=DIRECTION ( 'NONE',  ( -0.1566598588826321192, 0.9876526153536342445, 7.798540720466730171E-17 ) ) ;
#10564=DIRECTION ( 'NONE',  ( -0.1566598588826321192, 0.9876526153536342445, 7.798540720466730171E-17 ) ) ;
#10566=VERTEX_POINT ( 'NONE', #2243 ) ;
#10568=CYLINDRICAL_SURFACE ( 'NONE', #9099, 1.500000000000000666 ) ;
#10569=AXIS2_PLACEMENT_3D ( 'NONE', #6131, #9048, #11871 ) ;
#10570=CIRCLE ( 'NONE', #2402, 1.500000000000001332 ) ;
#10572=ORIENTED_EDGE ( 'NONE', *, *, #15672, .F. ) ;
#10574=AXIS2_PLACEMENT_3D ( 'NONE', #14351, #4300, #10072 ) ;
#10575=CIRCLE ( 'NONE', #2413, 1.500000000000000888 ) ;
#10576=CARTESIAN_POINT ( 'NONE',  ( -30.69897130211303349, -82.82467515726038698, 17.32050807568881368 ) ) ;
#10577=EDGE_CURVE ( 'NONE', #2139, #272, #16725, .T. ) ;
#10578=ORIENTED_EDGE ( 'NONE', *, *, #1871, .T. ) ;
#10579=CIRCLE ( 'NONE', #3306, 1.500000000000001332 ) ;
#10580=EDGE_CURVE ( 'NONE', #3795, #6562, #5477, .T. ) ;
#10582=CIRCLE ( 'NONE', #1531, 1.500000000000001332 ) ;
#10583=DIRECTION ( 'NONE',  ( -0.9876526153536336894, -0.1566598588826349503, 0.000000000000000000 ) ) ;
#10584=ORIENTED_EDGE ( 'NONE', *, *, #1580, .T. ) ;
#10587=ADVANCED_FACE ( 'NONE', ( #15594 ), #6907, .F. ) ;
#10588=DIRECTION ( 'NONE',  ( -0.1566598588826321192, 0.9876526153536342445, 7.798540720466730171E-17 ) ) ;
#10591=AXIS2_PLACEMENT_3D ( 'NONE', #18010, #3827, #5376 ) ;
#10592=DIRECTION ( 'NONE',  ( -0.9876526153536336894, -0.1566598588826350336, 0.000000000000000000 ) ) ;
#10593=CARTESIAN_POINT ( 'NONE',  ( -19.87442754340095519, -23.40223527320329922, 17.32050807568881012 ) ) ;
#10594=VECTOR ( 'NONE', #462, 1000.000000000000000 ) ;
#10595=CYLINDRICAL_SURFACE ( 'NONE', #15646, 1.500000000000001554 ) ;
#10596=DIRECTION ( 'NONE',  ( -0.1566598588826321192, 0.9876526153536342445, 7.798540720466731404E-17 ) ) ;
#10597=ORIENTED_EDGE ( 'NONE', *, *, #7448, .F. ) ;
#10598=VERTEX_POINT ( 'NONE', #11036 ) ;
#10599=AXIS2_PLACEMENT_3D ( 'NONE', #13106, #7082, #13011 ) ;
#10600=FACE_OUTER_BOUND ( 'NONE', #12489, .T. ) ;
#10602=ORIENTED_EDGE ( 'NONE', *, *, #9152, .F. ) ;
#10604=ORIENTED_EDGE ( 'NONE', *, *, #463, .T. ) ;
#10606=DIRECTION ( 'NONE',  ( -0.1566598588826321192, 0.9876526153536342445, 7.798540720466730171E-17 ) ) ;
#10607=ORIENTED_EDGE ( 'NONE', *, *, #15478, .F. ) ;
#10608=CARTESIAN_POINT ( 'NONE',  ( -15.92381708198642798, -22.77559583767277473, -21.65063509461098334 ) ) ;
#10609=AXIS2_PLACEMENT_3D ( 'NONE', #15324, #950, #2339 ) ;
#10610=DIRECTION ( 'NONE',  ( -0.9876526153536341335, -0.1566598588826327021, 0.000000000000000000 ) ) ;
#10612=EDGE_CURVE ( 'NONE', #1825, #11443, #4302, .T. ) ;
#10613=DIRECTION ( 'NONE',  ( -0.1566598588826321747, 0.9876526153536343555, 0.000000000000000000 ) ) ;
#10614=FACE_OUTER_BOUND ( 'NONE', #4882, .T. ) ;
#10615=ORIENTED_EDGE ( 'NONE', *, *, #13745, .F. ) ;
#10616=VECTOR ( 'NONE', #16769, 1000.000000000000000 ) ;
#10617=CARTESIAN_POINT ( 'NONE',  ( -56.21322099054479082, -24.10372711620989605, -21.65063509461097979 ) ) ;
#10618=ORIENTED_EDGE ( 'NONE', *, *, #9005, .T. ) ;
#10619=CYLINDRICAL_SURFACE ( 'NONE', #8329, 1.500000000000000666 ) ;
#10620=ADVANCED_FACE ( 'NONE', ( #16864 ), #15515, .F. ) ;
#10621=AXIS2_PLACEMENT_3D ( 'NONE', #4613, #7387, #17817 ) ;
#10625=ORIENTED_EDGE ( 'NONE', *, *, #690, .F. ) ;
#10627=DIRECTION ( 'NONE',  ( -0.9876526153536341335, -0.1566598588826327021, 0.000000000000000000 ) ) ;
#10628=AXIS2_PLACEMENT_3D ( 'NONE', #4115, #5571, #17138 ) ;
#10629=VERTEX_POINT ( 'NONE', #5379 ) ;
#10630=FACE_BOUND ( 'NONE', #7213, .T. ) ;
#10631=CIRCLE ( 'NONE', #17324, 1.500000000000000888 ) ;
#10632=ORIENTED_EDGE ( 'NONE', *, *, #13766, .T. ) ;
#10634=EDGE_CURVE ( 'NONE', #6863, #17521, #4025, .T. ) ;
#10636=CIRCLE ( 'NONE', #3967, 1.500000000000000888 ) ;
#10637=CIRCLE ( 'NONE', #16405, 1.500000000000000444 ) ;
#10638=EDGE_CURVE ( 'NONE', #6457, #17941, #9766, .T. ) ;
#10639=ORIENTED_EDGE ( 'NONE', *, *, #5490, .T. ) ;
#10640=EDGE_CURVE ( 'NONE', #6894, #8134, #16424, .T. ) ;
#10641=DIRECTION ( 'NONE',  ( -0.9876526153536341335, -0.1566598588826327021, 0.000000000000000000 ) ) ;
#10642=CARTESIAN_POINT ( 'NONE',  ( -15.92381708198643153, -22.77559583767277473, 12.99038105676661381 ) ) ;
#10643=EDGE_CURVE ( 'NONE', #5513, #2328, #12154, .T. ) ;
#10644=CIRCLE ( 'NONE', #15799, 1.500000000000000888 ) ;
#10646=CARTESIAN_POINT ( 'NONE',  ( -65.30644784966793281, -30.60858878180435738, -12.99038105676658006 ) ) ;
#10647=ORIENTED_EDGE ( 'NONE', *, *, #6884, .T. ) ;
#10648=ORIENTED_EDGE ( 'NONE', *, *, #7635, .F. ) ;
#10649=FACE_OUTER_BOUND ( 'NONE', #8965, .T. ) ;
#10650=CARTESIAN_POINT ( 'NONE',  ( -65.10209452872744862, -25.51366584615359656, 17.32050807568881723 ) ) ;
#10651=AXIS2_PLACEMENT_3D ( 'NONE', #12298, #9572, #2361 ) ;
#10652=ORIENTED_EDGE ( 'NONE', *, *, #10884, .T. ) ;
#10653=CARTESIAN_POINT ( 'NONE',  ( -51.97313754239392836, -28.49368068688882971, -4.330127018922181215 ) ) ;
#10654=CIRCLE ( 'NONE', #1878, 1.500000000000000000 ) ;
#10655=DIRECTION ( 'NONE',  ( -0.1566598588826321192, 0.9876526153536342445, 7.798540720466730171E-17 ) ) ;
#10657=DIRECTION ( 'NONE',  ( -0.1566598588826321192, 0.9876526153536342445, 7.798540720466730171E-17 ) ) ;
#10659=EDGE_CURVE ( 'NONE', #9088, #4142, #3250, .T. ) ;
#10660=EDGE_CURVE ( 'NONE', #1682, #3315, #6962, .T. ) ;
#10661=ADVANCED_FACE ( 'NONE', ( #17339 ), #2715, .T. ) ;
#10662=CARTESIAN_POINT ( 'NONE',  ( -45.34904222165486942, -22.38046866850095284, -8.660254037844380193 ) ) ;
#10663=CYLINDRICAL_SURFACE ( 'NONE', #5663, 1.500000000000001554 ) ;
#10664=CARTESIAN_POINT ( 'NONE',  ( -29.25712738926042888, -24.89050393258829175, -12.99038105676658006 ) ) ;
#10665=VERTEX_POINT ( 'NONE', #14463 ) ;
#10666=AXIS2_PLACEMENT_3D ( 'NONE', #11366, #14332, #4276 ) ;
#10667=CARTESIAN_POINT ( 'NONE',  ( -61.31620237807555895, -87.68113078262194904, -12.99038105676658539 ) ) ;
#10668=ORIENTED_EDGE ( 'NONE', *, *, #1940, .T. ) ;
#10669=EDGE_LOOP ( 'NONE', ( #6316, #612, #8721, #15311 ) ) ;
#10670=VERTEX_POINT ( 'NONE', #4222 ) ;
#10672=CARTESIAN_POINT ( 'NONE',  ( -30.53425299135042081, -20.03057078526148160, 1.908195823574487804E-14 ) ) ;
#10673=VERTEX_POINT ( 'NONE', #13121 ) ;
#10676=DIRECTION ( 'NONE',  ( 0.000000000000000000, 0.000000000000000000, 1.000000000000000000 ) ) ;
#10677=ORIENTED_EDGE ( 'NONE', *, *, #8184, .F. ) ;
#10678=CARTESIAN_POINT ( 'NONE',  ( -70.20507591625822386, -89.09106951256565310, 17.32050807568881368 ) ) ;
#10680=DIRECTION ( 'NONE',  ( -0.1566598588826321192, 0.9876526153536342445, 7.798540720466730171E-17 ) ) ;
#10681=CYLINDRICAL_SURFACE ( 'NONE', #6245, 1.500000000000001554 ) ;
#10682=CARTESIAN_POINT ( 'NONE',  ( 0.4120860815263194254, -77.88988960245745830, 17.32050807568880657 ) ) ;
#10683=CARTESIAN_POINT ( 'NONE',  ( -17.40529600501687923, -23.01058562599671831, -21.65063509461098334 ) ) ;
#10684=DIRECTION ( 'NONE',  ( 0.000000000000000000, 0.000000000000000000, 1.000000000000000000 ) ) ;
#10687=ADVANCED_FACE ( 'NONE', ( #4116 ), #10097, .F. ) ;
#10688=EDGE_CURVE ( 'NONE', #3161, #11647, #5852, .T. ) ;
#10690=VECTOR ( 'NONE', #2833, 1000.000000000000000 ) ;
#10691=ORIENTED_EDGE ( 'NONE', *, *, #6465, .F. ) ;
#10692=VERTEX_POINT ( 'NONE', #8510 ) ;
#10694=CARTESIAN_POINT ( 'NONE',  ( -84.23462711737164454, 33.01666666666666572, -30.00000000000000000 ) ) ;
#10695=DIRECTION ( 'NONE',  ( -0.1566598588826321747, 0.9876526153536343555, 0.000000000000000000 ) ) ;
#10699=DIRECTION ( 'NONE',  ( -0.9876526153536341335, -0.1566598588826327021, 0.000000000000000000 ) ) ;
#10700=CARTESIAN_POINT ( 'NONE',  ( -48.02252708097939404, -27.86704125135830523, 17.32050807568881723 ) ) ;
#10702=EDGE_CURVE ( 'NONE', #3364, #931, #12321, .T. ) ;
#10703=CARTESIAN_POINT ( 'NONE',  ( -32.22008523532134205, -25.36048350923618955, 21.65063509461101887 ) ) ;
#10704=EDGE_LOOP ( 'NONE', ( #10106, #11747 ) ) ;
#10706=VERTEX_POINT ( 'NONE', #15803 ) ;
#10708=EDGE_CURVE ( 'NONE', #2965, #13292, #12988, .T. ) ;
#10709=FACE_BOUND ( 'NONE', #17111, .T. ) ;
#10710=FACE_OUTER_BOUND ( 'NONE', #12613, .T. ) ;
#10711=EDGE_CURVE ( 'NONE', #2692, #3641, #13895, .T. ) ;
#10712=VERTEX_POINT ( 'NONE', #4324 ) ;
#10713=ORIENTED_EDGE ( 'NONE', *, *, #3850, .T. ) ;
#10714=FACE_OUTER_BOUND ( 'NONE', #776, .T. ) ;
#10715=DIRECTION ( 'NONE',  ( 0.000000000000000000, 0.000000000000000000, 1.000000000000000000 ) ) ;
#10719=ORIENTED_EDGE ( 'NONE', *, *, #3610, .T. ) ;
#10720=EDGE_LOOP ( 'NONE', ( #11689, #2009 ) ) ;
#10722=CIRCLE ( 'NONE', #6507, 1.500000000000000888 ) ;
#10723=CARTESIAN_POINT ( 'NONE',  ( -66.29410046502155751, -30.76524864068697696, 1.887572821959364500E-14 ) ) ;
#10726=ADVANCED_FACE ( 'NONE', ( #11678 ), #10282, .F. ) ;
#10727=ORIENTED_EDGE ( 'NONE', *, *, #5588, .F. ) ;
#10728=PLANE ( 'NONE',  #12437 ) ;
#10729=FACE_OUTER_BOUND ( 'NONE', #4925, .T. ) ;
#10730=EDGE_CURVE ( 'NONE', #1541, #2560, #6609, .T. ) ;
#10732=CARTESIAN_POINT ( 'NONE',  ( -38.14600092744309734, -26.30044266253198160, 1.175313729581431390E-14 ) ) ;
#10733=ORIENTED_EDGE ( 'NONE', *, *, #9925, .F. ) ;
#10734=CARTESIAN_POINT ( 'NONE',  ( -58.68235252892886678, -24.49537676341648051, -8.660254037844380193 ) ) ;
#10735=CARTESIAN_POINT ( 'NONE',  ( -39.62747985047357702, -26.53543245085592517, -17.32050807568878170 ) ) ;
#10736=DIRECTION ( 'NONE',  ( -0.1566598588826321192, 0.9876526153536342445, 7.798540720466730171E-17 ) ) ;
#10737=DIRECTION ( 'NONE',  ( -0.9876526153536336894, -0.1566598588826349503, 0.000000000000000000 ) ) ;
#10738=EDGE_LOOP ( 'NONE', ( #12547, #15089 ) ) ;
#10739=EDGE_LOOP ( 'NONE', ( #16957, #1403, #16667, #15563 ) ) ;
#10740=LINE ( 'NONE', #352, #15761 ) ;
#10741=ORIENTED_EDGE ( 'NONE', *, *, #18523, .F. ) ;
#10742=CARTESIAN_POINT ( 'NONE',  ( 5.350349158294472218, -77.10659030804430358, 17.32050807568880657 ) ) ;
#10743=VECTOR ( 'NONE', #3235, 1000.000000000000000 ) ;
#10744=ORIENTED_EDGE ( 'NONE', *, *, #10412, .T. ) ;
#10745=EDGE_CURVE ( 'NONE', #12642, #5059, #14378, .T. ) ;
#10746=EDGE_CURVE ( 'NONE', #16739, #405, #3291, .T. ) ;
#10747=CARTESIAN_POINT ( 'NONE',  ( -66.08974714408108753, -25.67032570503621614, -12.99038105676658006 ) ) ;
#10748=EDGE_CURVE ( 'NONE', #16279, #5230, #13281, .T. ) ;
#10749=LINE ( 'NONE', #15416, #2430 ) ;
#10751=DIRECTION ( 'NONE',  ( 0.000000000000000000, 0.000000000000000000, 1.000000000000000000 ) ) ;
#10752=DIRECTION ( 'NONE',  ( -0.1566598588826321192, 0.9876526153536342445, 7.798540720466730171E-17 ) ) ;
#10753=CYLINDRICAL_SURFACE ( 'NONE', #6950, 1.500000000000001554 ) ;
#10754=CIRCLE ( 'NONE', #15614, 1.500000000000000888 ) ;
#10755=DIRECTION ( 'NONE',  ( -0.1566598588826321192, 0.9876526153536342445, 7.798540720466730171E-17 ) ) ;
#10756=CYLINDRICAL_SURFACE ( 'NONE', #7229, 1.500000000000000888 ) ;
#10757=DIRECTION ( 'NONE',  ( -0.9876526153536336894, -0.1566598588826349503, 0.000000000000000000 ) ) ;
#10758=DIRECTION ( 'NONE',  ( -0.9876526153536341335, -0.1566598588826327576, 0.000000000000000000 ) ) ;
#10761=VECTOR ( 'NONE', #6846, 1000.000000000000000 ) ;
#10763=ADVANCED_FACE ( 'NONE', ( #1588 ), #9908, .F. ) ;
#10764=ORIENTED_EDGE ( 'NONE', *, *, #596, .T. ) ;
#10765=ADVANCED_FACE ( 'NONE', ( #12846 ), #11410, .F. ) ;
#10766=ORIENTED_EDGE ( 'NONE', *, *, #555, .F. ) ;
#10767=CARTESIAN_POINT ( 'NONE',  ( -12.46703292824873088, -22.22728633158356359, -21.65063509461098334 ) ) ;
#10768=CARTESIAN_POINT ( 'NONE',  ( -33.99103714508810725, -20.57888029135069985, 17.32050807568882078 ) ) ;
#10769=DIRECTION ( 'NONE',  ( -0.9876526153536344665, -0.1566598588826304539, 0.000000000000000000 ) ) ;
#10770=FACE_OUTER_BOUND ( 'NONE', #3788, .T. ) ;
#10771=EDGE_CURVE ( 'NONE', #17353, #2946, #16281, .T. ) ;
#10775=EDGE_LOOP ( 'NONE', ( #7139, #1937 ) ) ;
#10776=DIRECTION ( 'NONE',  ( -0.1566598588826321747, 0.9876526153536343555, 0.000000000000000000 ) ) ;
#10777=ORIENTED_EDGE ( 'NONE', *, *, #14901, .T. ) ;
#10778=FACE_BOUND ( 'NONE', #12425, .T. ) ;
#10779=FACE_OUTER_BOUND ( 'NONE', #3216, .T. ) ;
#10782=VECTOR ( 'NONE', #18195, 1000.000000000000000 ) ;
#10784=VERTEX_POINT ( 'NONE', #3349 ) ;
#10785=CARTESIAN_POINT ( 'NONE',  ( -88.14047854185180597, -33.59999999999994458, 25.00000000000001776 ) ) ;
#10786=ORIENTED_EDGE ( 'NONE', *, *, #11593, .T. ) ;
#10787=ORIENTED_EDGE ( 'NONE', *, *, #7756, .F. ) ;
#10788=ORIENTED_EDGE ( 'NONE', *, *, #631, .T. ) ;
#10789=ORIENTED_EDGE ( 'NONE', *, *, #101, .T. ) ;
#10791=DIRECTION ( 'NONE',  ( 0.000000000000000000, 0.000000000000000000, 1.000000000000000000 ) ) ;
#10792=VECTOR ( 'NONE', #12965, 1000.000000000000000 ) ;
#10793=FACE_BOUND ( 'NONE', #8608, .T. ) ;
#10794=CARTESIAN_POINT ( 'NONE',  ( -66.25446545484369665, -88.46443007703511796, -4.330127018922185655 ) ) ;
#10797=ORIENTED_EDGE ( 'NONE', *, *, #14791, .F. ) ;
#10799=CIRCLE ( 'NONE', #15656, 2.000000000000000000 ) ;
#10800=FACE_BOUND ( 'NONE', #16487, .T. ) ;
#10801=EDGE_CURVE ( 'NONE', #10229, #12874, #12665, .T. ) ;
#10805=CARTESIAN_POINT ( 'NONE',  ( -17.85948730251583783, -80.78809699178616199, -8.660254037844385522 ) ) ;
#10806=ORIENTED_EDGE ( 'NONE', *, *, #12886, .F. ) ;
#10808=AXIS2_PLACEMENT_3D ( 'NONE', #18688, #2814, #12929 ) ;
#10809=LINE ( 'NONE', #4670, #13912 ) ;
#10810=AXIS2_PLACEMENT_3D ( 'NONE', #3395, #3856, #10875 ) ;
#10811=DIRECTION ( 'NONE',  ( 0.000000000000000000, 0.000000000000000000, 1.000000000000000000 ) ) ;
#10813=DIRECTION ( 'NONE',  ( -0.9876526153536341335, -0.1566598588826327021, 0.000000000000000000 ) ) ;
#10814=CARTESIAN_POINT ( 'NONE',  ( -73.49714175923330117, -26.84527464665595531, -8.660254037844380193 ) ) ;
#10816=VERTEX_POINT ( 'NONE', #16536 ) ;
#10817=FACE_BOUND ( 'NONE', #13393, .T. ) ;
#10818=CIRCLE ( 'NONE', #9024, 1.499999999999999556 ) ;
#10820=AXIS2_PLACEMENT_3D ( 'NONE', #1806, #17318, #9885 ) ;
#10821=CARTESIAN_POINT ( 'NONE',  ( -56.41757431148526081, -29.19865005186066753, -17.32050807568878170 ) ) ;
#10822=LINE ( 'NONE', #11108, #18183 ) ;
#10824=AXIS2_PLACEMENT_3D ( 'NONE', #3101, #7035, #6443 ) ;
#10826=EDGE_CURVE ( 'NONE', #14760, #10382, #9155, .T. ) ;
#10827=DIRECTION ( 'NONE',  ( -0.1566598588826321192, 0.9876526153536342445, 7.798540720466731404E-17 ) ) ;
#10828=CARTESIAN_POINT ( 'NONE',  ( 1.399738696879940791, -77.73322974357483872, 12.99038105676660493 ) ) ;
#10830=CIRCLE ( 'NONE', #13573, 1.500000000000000888 ) ;
#10831=CARTESIAN_POINT ( 'NONE',  ( -61.15148406731292852, -24.88702641062307208, 21.65063509461102242 ) ) ;
#10833=ORIENTED_EDGE ( 'NONE', *, *, #8069, .T. ) ;
#10834=DIRECTION ( 'NONE',  ( -0.1566598588826321747, 0.9876526153536343555, 0.000000000000000000 ) ) ;
#10835=CARTESIAN_POINT ( 'NONE',  ( -72.50948914387967648, -26.68861478777333218, 12.99038105676661736 ) ) ;
#10836=VECTOR ( 'NONE', #1816, 1000.000000000000000 ) ;
#10838=EDGE_CURVE ( 'NONE', #11621, #15511, #11463, .T. ) ;
#10839=CIRCLE ( 'NONE', #17237, 1.499999999999999556 ) ;
#10840=EDGE_LOOP ( 'NONE', ( #11024, #8635, #15186, #5293 ) ) ;
#10841=CARTESIAN_POINT ( 'NONE',  ( -71.23236354178969520, -31.54854793510013877, -17.32050807568878170 ) ) ;
#10843=DIRECTION ( 'NONE',  ( 0.000000000000000000, 0.000000000000000000, 1.000000000000000000 ) ) ;
#10844=CARTESIAN_POINT ( 'NONE',  ( 8.807133312032172867, -76.55828080195509244, 9.043241838514131834E-15 ) ) ;
#10845=CARTESIAN_POINT ( 'NONE',  ( -39.13365354279672914, -26.45710252141460828, 12.99038105676661736 ) ) ;
#10846=CIRCLE ( 'NONE', #12981, 1.500000000000000888 ) ;
#10847=ORIENTED_EDGE ( 'NONE', *, *, #3852, .F. ) ;
#10848=CARTESIAN_POINT ( 'NONE',  ( -1.892327146095121204, -15.48743487766515337, -12.99038105676658361 ) ) ;
#10849=AXIS2_PLACEMENT_3D ( 'NONE', #18221, #5195, #16866 ) ;
#10850=CIRCLE ( 'NONE', #11426, 1.500000000000000000 ) ;
#10852=AXIS2_PLACEMENT_3D ( 'NONE', #13397, #3526, #12243 ) ;
#10853=CYLINDRICAL_SURFACE ( 'NONE', #10471, 1.500000000000001554 ) ;
#10854=FACE_BOUND ( 'NONE', #12701, .T. ) ;
#10855=EDGE_CURVE ( 'NONE', #6097, #9271, #17903, .T. ) ;
#10857=CARTESIAN_POINT ( 'NONE',  ( -36.66452200441264608, -26.06545287420802737, 1.193683431568641663E-14 ) ) ;
#10858=EDGE_CURVE ( 'NONE', #3849, #15836, #7645, .T. ) ;
#10859=ORIENTED_EDGE ( 'NONE', *, *, #17660, .T. ) ;
#10860=EDGE_CURVE ( 'NONE', #16572, #8813, #4166, .T. ) ;
#10862=VERTEX_POINT ( 'NONE', #13582 ) ;
#10863=VECTOR ( 'NONE', #14178, 1000.000000000000000 ) ;
#10864=DIRECTION ( 'NONE',  ( -0.1566598588826321747, 0.9876526153536343555, 0.000000000000000000 ) ) ;
#10865=VECTOR ( 'NONE', #6570, 1000.000000000000000 ) ;
#10866=ORIENTED_EDGE ( 'NONE', *, *, #3222, .F. ) ;
#10867=CARTESIAN_POINT ( 'NONE',  ( -47.48906576312474215, -85.48789275826510448, -17.32050807568878525 ) ) ;
#10869=AXIS2_PLACEMENT_3D ( 'NONE', #5032, #17892, #515 ) ;
#10870=CARTESIAN_POINT ( 'NONE',  ( -74.97862068226375243, -27.08026443497991309, 17.32050807568881723 ) ) ;
#10871=EDGE_LOOP ( 'NONE', ( #5081, #17152, #1651, #4190 ) ) ;
#10872=DIRECTION ( 'NONE',  ( -0.1566598588826321747, 0.9876526153536343555, 0.000000000000000000 ) ) ;
#10873=FACE_OUTER_BOUND ( 'NONE', #9579, .T. ) ;
#10874=DIRECTION ( 'NONE',  ( -0.1566598588826321192, 0.9876526153536342445, 7.798540720466730171E-17 ) ) ;
#10875=DIRECTION ( 'NONE',  ( -0.9876526153536336894, -0.1566598588826349503, 0.000000000000000000 ) ) ;
#10878=DIRECTION ( 'NONE',  ( -0.1566598588826321747, 0.9876526153536343555, 0.000000000000000000 ) ) ;
#10879=AXIS2_PLACEMENT_3D ( 'NONE', #3942, #12655, #5290 ) ;
#10880=CARTESIAN_POINT ( 'NONE',  ( -5.513829610595458064, -78.82984875575324679, -12.99038105676658539 ) ) ;
#10882=EDGE_LOOP ( 'NONE', ( #5510, #11021 ) ) ;
#10883=AXIS2_PLACEMENT_3D ( 'NONE', #419, #18163, #14038 ) ;
#10884=EDGE_CURVE ( 'NONE', #9527, #1938, #17268, .T. ) ;
#10886=DIRECTION ( 'NONE',  ( -0.9876526153536344665, -0.1566598588826304539, 0.000000000000000000 ) ) ;
#10888=CARTESIAN_POINT ( 'NONE',  ( -54.44226908077801852, -28.88533033409541062, -8.660254037844380193 ) ) ;
#10889=EDGE_LOOP ( 'NONE', ( #9811, #15740 ) ) ;
#10890=ORIENTED_EDGE ( 'NONE', *, *, #17484, .T. ) ;
#10891=ORIENTED_EDGE ( 'NONE', *, *, #18720, .F. ) ;
#10892=CIRCLE ( 'NONE', #10591, 2.500000000000002220 ) ;
#10894=DIRECTION ( 'NONE',  ( -0.1566598588826321192, 0.9876526153536342445, 7.798540720466730171E-17 ) ) ;
#10895=AXIS2_PLACEMENT_3D ( 'NONE', #17912, #15122, #7928 ) ;
#10896=FACE_BOUND ( 'NONE', #17534, .T. ) ;
#10897=ORIENTED_EDGE ( 'NONE', *, *, #17001, .F. ) ;
#10898=CIRCLE ( 'NONE', #14849, 1.500000000000001332 ) ;
#10899=EDGE_LOOP ( 'NONE', ( #18400, #1952 ) ) ;
#10900=LINE ( 'NONE', #3875, #1290 ) ;
#10901=AXIS2_PLACEMENT_3D ( 'NONE', #13208, #8770, #10176 ) ;
#10903=CIRCLE ( 'NONE', #2767, 1.499999999999999556 ) ;
#10906=CARTESIAN_POINT ( 'NONE',  ( -78.43540483600145308, -27.62857394106911357, -8.660254037844380193 ) ) ;
#10907=VERTEX_POINT ( 'NONE', #1853 ) ;
#10908=EDGE_LOOP ( 'NONE', ( #7297, #3996 ) ) ;
#10910=ORIENTED_EDGE ( 'NONE', *, *, #18443, .T. ) ;
#10911=ADVANCED_FACE ( 'NONE', ( #433 ), #17799, .F. ) ;
#10913=VERTEX_POINT ( 'NONE', #15014 ) ;
#10914=ORIENTED_EDGE ( 'NONE', *, *, #8971, .T. ) ;
#10915=CYLINDRICAL_SURFACE ( 'NONE', #13043, 1.500000000000000666 ) ;
#10916=ADVANCED_FACE ( 'NONE', ( #7917 ), #12156, .F. ) ;
#10917=ORIENTED_EDGE ( 'NONE', *, *, #10140, .F. ) ;
#10920=AXIS2_PLACEMENT_3D ( 'NONE', #12491, #18333, #5301 ) ;
#10921=CIRCLE ( 'NONE', #2461, 1.500000000000001332 ) ;
#10922=CARTESIAN_POINT ( 'NONE',  ( -25.80034323552273534, -24.34219442649909126, 12.99038105676661736 ) ) ;
#10923=EDGE_CURVE ( 'NONE', #15832, #16090, #3588, .T. ) ;
#10924=CYLINDRICAL_SURFACE ( 'NONE', #13027, 1.500000000000001554 ) ;
#10925=AXIS2_PLACEMENT_3D ( 'NONE', #13055, #8892, #5953 ) ;
#10926=DIRECTION ( 'NONE',  ( -0.9876526153536341335, -0.1566598588826327021, 0.000000000000000000 ) ) ;
#10930=DIRECTION ( 'NONE',  ( -0.1566598588826321192, 0.9876526153536342445, 7.798540720466730171E-17 ) ) ;
#10931=DIRECTION ( 'NONE',  ( -0.1566598588826321192, 0.9876526153536342445, 7.798540720466731404E-17 ) ) ;
#10932=AXIS2_PLACEMENT_3D ( 'NONE', #8256, #14019, #12579 ) ;
#10933=CARTESIAN_POINT ( 'NONE',  ( -38.14600092744311155, -26.30044266253198160, -17.32050807568878170 ) ) ;
#10934=VERTEX_POINT ( 'NONE', #16254 ) ;
#10935=ORIENTED_EDGE ( 'NONE', *, *, #17731, .T. ) ;
#10936=FACE_BOUND ( 'NONE', #16273, .T. ) ;
#10937=CARTESIAN_POINT ( 'NONE',  ( -1.069392841504132052, -78.12487939078141608, -17.32050807568878525 ) ) ;
#10938=EDGE_LOOP ( 'NONE', ( #9843, #5394, #11288, #302 ) ) ;
#10939=EDGE_CURVE ( 'NONE', #13454, #6106, #911, .T. ) ;
#10940=DIRECTION ( 'NONE',  ( -0.9876526153536336894, -0.1566598588826349503, 0.000000000000000000 ) ) ;
#10941=EDGE_LOOP ( 'NONE', ( #15858, #11306 ) ) ;
#10942=CARTESIAN_POINT ( 'NONE',  ( -68.55887868246516348, -26.06197535224279704, -8.660254037844380193 ) ) ;
#10943=DIRECTION ( 'NONE',  ( -0.1566598588826321192, 0.9876526153536342445, 7.798540720466730171E-17 ) ) ;
#10944=EDGE_CURVE ( 'NONE', #3259, #5362, #9015, .T. ) ;
#10945=CARTESIAN_POINT ( 'NONE',  ( -19.34096622554629263, -81.02308678011010556, 1.424741226644455312E-14 ) ) ;
#10946=DIRECTION ( 'NONE',  ( 0.000000000000000000, 0.000000000000000000, 1.000000000000000000 ) ) ;
#10947=EDGE_LOOP ( 'NONE', ( #8244, #8854 ) ) ;
#10948=CIRCLE ( 'NONE', #2182, 1.500000000000001332 ) ;
#10949=DIRECTION ( 'NONE',  ( -0.9876526153536336894, -0.1566598588826349503, 0.000000000000000000 ) ) ;
#10950=CARTESIAN_POINT ( 'NONE',  ( -69.54653129781877396, -26.21863521112543083, -12.99038105676658006 ) ) ;
#10951=DIRECTION ( 'NONE',  ( 0.000000000000000000, 0.000000000000000000, 1.000000000000000000 ) ) ;
#10952=( LENGTH_UNIT ( ) NAMED_UNIT ( * ) SI_UNIT ( .MILLI., .METRE. ) );
#10956=DIRECTION ( 'NONE',  ( -0.9876526153536336894, -0.1566598588826350336, 0.000000000000000000 ) ) ;
#10957=CARTESIAN_POINT ( 'NONE',  ( 7.819480696678551723, -76.71494066083772623, -4.330127018922189208 ) ) ;
#10958=DIRECTION ( 'NONE',  ( -0.1566598588826321192, 0.9876526153536342445, 7.798540720466731404E-17 ) ) ;
#10959=ORIENTED_EDGE ( 'NONE', *, *, #10745, .T. ) ;
#10961=CYLINDRICAL_SURFACE ( 'NONE', #17487, 1.500000000000000666 ) ;
#10963=AXIS2_PLACEMENT_3D ( 'NONE', #13357, #6177, #11905 ) ;
#10966=DIRECTION ( 'NONE',  ( 0.000000000000000000, 0.000000000000000000, 1.000000000000000000 ) ) ;
#10967=CYLINDRICAL_SURFACE ( 'NONE', #6539, 1.500000000000001554 ) ;
#10968=CARTESIAN_POINT ( 'NONE',  ( -46.54104815794895700, -27.63205146303434390, -8.660254037844380193 ) ) ;
#10969=DIRECTION ( 'NONE',  ( -0.1566598588826321747, 0.9876526153536343555, 0.000000000000000000 ) ) ;
#10970=EDGE_CURVE ( 'NONE', #5711, #10784, #13968, .T. ) ;
#10972=DIRECTION ( 'NONE',  ( -0.9876526153536341335, -0.1566598588826327576, 0.000000000000000000 ) ) ;
#10973=FACE_OUTER_BOUND ( 'NONE', #15213, .T. ) ;
#10974=CARTESIAN_POINT ( 'NONE',  ( -49.50400600400987372, -28.10203103968224170, -17.32050807568878170 ) ) ;
#10975=ORIENTED_EDGE ( 'NONE', *, *, #16669, .T. ) ;
#10976=FACE_BOUND ( 'NONE', #18329, .T. ) ;
#10977=CARTESIAN_POINT ( 'NONE',  ( -9.299721761247353058, -16.66238381928489787, -8.660254037844380193 ) ) ;
#10979=DIRECTION ( 'NONE',  ( -0.1566598588826321192, 0.9876526153536342445, 7.798540720466730171E-17 ) ) ;
#10980=ORIENTED_EDGE ( 'NONE', *, *, #11760, .F. ) ;
#10981=ORIENTED_EDGE ( 'NONE', *, *, #872, .T. ) ;
#10982=CYLINDRICAL_SURFACE ( 'NONE', #8371, 1.500000000000000666 ) ;
#10983=FACE_BOUND ( 'NONE', #13344, .T. ) ;
#10984=EDGE_CURVE ( 'NONE', #2681, #12551, #10850, .T. ) ;
#10985=EDGE_CURVE ( 'NONE', #9759, #4810, #6881, .T. ) ;
#10987=EDGE_CURVE ( 'NONE', #8469, #6106, #12451, .T. ) ;
#10991=CARTESIAN_POINT ( 'NONE',  ( -22.63303206852135929, -18.77729191420043264, 1.926565525561698076E-14 ) ) ;
#10992=DIRECTION ( 'NONE',  ( 0.000000000000000000, 0.000000000000000000, 1.000000000000000000 ) ) ;
#10993=CARTESIAN_POINT ( 'NONE',  ( -15.92381708198643153, -22.77559583767277473, 21.65063509461101177 ) ) ;
#10994=ORIENTED_EDGE ( 'NONE', *, *, #8703, .F. ) ;
#10996=DIRECTION ( 'NONE',  ( -0.9876526153536341335, -0.1566598588826327021, 0.000000000000000000 ) ) ;
#10997=ORIENTED_EDGE ( 'NONE', *, *, #8118, .F. ) ;
#10998=DIRECTION ( 'NONE',  ( 0.000000000000000000, 0.000000000000000000, 1.000000000000000000 ) ) ;
#10999=CYLINDRICAL_SURFACE ( 'NONE', #15753, 1.500000000000001554 ) ;
#11000=DIRECTION ( 'NONE',  ( -0.1566598588826321192, 0.9876526153536342445, 7.798540720466730171E-17 ) ) ;
#11001=ORIENTED_EDGE ( 'NONE', *, *, #17194, .T. ) ;
#11002=EDGE_LOOP ( 'NONE', ( #5514, #13361, #2419, #12392 ) ) ;
#11003=CARTESIAN_POINT ( 'NONE',  ( -44.03228160938703439, -84.93958325217590755, 8.660254037844412167 ) ) ;
#11006=EDGE_CURVE ( 'NONE', #17992, #3563, #3802, .T. ) ;
#11007=DIRECTION ( 'NONE',  ( -0.9876526153536341335, -0.1566598588826327021, 0.000000000000000000 ) ) ;
#11008=EDGE_CURVE ( 'NONE', #6102, #3468, #10822, .T. ) ;
#11009=CARTESIAN_POINT ( 'NONE',  ( -50.28730529842302843, -23.16376796291410756, -17.32050807568878170 ) ) ;
#11010=CARTESIAN_POINT ( 'NONE',  ( -51.27495791377664602, -23.32042782179674134, -12.99038105676658006 ) ) ;
#11014=EDGE_CURVE ( 'NONE', #98, #8230, #18080, .T. ) ;
#11015=DIRECTION ( 'NONE',  ( -0.1566598588826321192, 0.9876526153536342445, 7.798540720466730171E-17 ) ) ;
#11016=CIRCLE ( 'NONE', #11910, 1.500000000000000888 ) ;
#11017=CARTESIAN_POINT ( 'NONE',  ( -47.81817376003893827, -22.77211831570753020, -12.99038105676658006 ) ) ;
#11018=CARTESIAN_POINT ( 'NONE',  ( -58.84707083969148300, -87.28948113541537168, 17.32050807568881368 ) ) ;
#11019=CARTESIAN_POINT ( 'NONE',  ( -35.47251606811855851, -20.81387007967463987, 1.908195823574487804E-14 ) ) ;
#11021=ORIENTED_EDGE ( 'NONE', *, *, #15973, .F. ) ;
#11022=CARTESIAN_POINT ( 'NONE',  ( -59.38053215754616332, -29.66862962850856533, 1.869203119972154228E-14 ) ) ;
#11023=DIRECTION ( 'NONE',  ( -0.9876526153536336894, -0.1566598588826350336, 0.000000000000000000 ) ) ;
#11024=ORIENTED_EDGE ( 'NONE', *, *, #7408, .F. ) ;
#11027=EDGE_LOOP ( 'NONE', ( #15877, #7323, #12649, #18033 ) ) ;
#11028=CYLINDRICAL_SURFACE ( 'NONE', #3948, 1.500000000000001554 ) ;
#11029=FACE_OUTER_BOUND ( 'NONE', #8320, .T. ) ;
#11030=ORIENTED_EDGE ( 'NONE', *, *, #7944, .F. ) ;
#11031=AXIS2_PLACEMENT_3D ( 'NONE', #9161, #10564, #12160 ) ;
#11032=CARTESIAN_POINT ( 'NONE',  ( -61.84966369593023217, -30.06027927571513914, 12.99038105676661736 ) ) ;
#11033=DIRECTION ( 'NONE',  ( -0.1566598588826321747, 0.9876526153536343555, 0.000000000000000000 ) ) ;
#11034=CARTESIAN_POINT ( 'NONE',  ( -26.78799585087635649, -24.49885428538171794, 17.32050807568881723 ) ) ;
#11035=ORIENTED_EDGE ( 'NONE', *, *, #11898, .F. ) ;
#11036=CARTESIAN_POINT ( 'NONE',  ( -12.75650591498505371, -17.21069332537411256, 8.660254037844413944 ) ) ;
#11038=EDGE_CURVE ( 'NONE', #6863, #4996, #6621, .T. ) ;
#11040=ORIENTED_EDGE ( 'NONE', *, *, #13483, .T. ) ;
#11041=PRODUCT_DEFINITION_SHAPE ( 'NONE', 'NONE',  #9414 ) ;
#11043=DIRECTION ( 'NONE',  ( 0.000000000000000000, 0.000000000000000000, 1.000000000000000000 ) ) ;
#11044=ORIENTED_EDGE ( 'NONE', *, *, #13511, .F. ) ;
#11045=DIRECTION ( 'NONE',  ( -0.1566598588826321192, 0.9876526153536342445, 7.798540720466730171E-17 ) ) ;
#11046=DIRECTION ( 'NONE',  ( -0.1566598588826321747, 0.9876526153536343555, 0.000000000000000000 ) ) ;
#11047=ORIENTED_EDGE ( 'NONE', *, *, #11070, .T. ) ;
#11048=CARTESIAN_POINT ( 'NONE',  ( -10.45209268736360997, -79.61314805016641571, 21.65063509461100821 ) ) ;
#11049=EDGE_CURVE ( 'NONE', #2279, #13719, #3857, .T. ) ;
#11051=LINE ( 'NONE', #14005, #12924 ) ;
#11052=ORIENTED_EDGE ( 'NONE', *, *, #18353, .T. ) ;
#11053=CARTESIAN_POINT ( 'NONE',  ( -40.61513246582717329, -26.69209230973856251, -4.330127018922181215 ) ) ;
#11054=ORIENTED_EDGE ( 'NONE', *, *, #1067, .T. ) ;
#11055=EDGE_LOOP ( 'NONE', ( #18177, #18169, #8654, #7788 ) ) ;
#11056=AXIS2_PLACEMENT_3D ( 'NONE', #14020, #9382, #15249 ) ;
#11058=DIRECTION ( 'NONE',  ( -0.1566598588826321192, 0.9876526153536342445, 7.798540720466731404E-17 ) ) ;
#11059=ORIENTED_EDGE ( 'NONE', *, *, #7949, .F. ) ;
#11060=CARTESIAN_POINT ( 'NONE',  ( -5.842937607509656850, -16.11407431319567962, 8.660254037844412167 ) ) ;
#11061=CARTESIAN_POINT ( 'NONE',  ( -60.36818477289977380, -29.82528948739119556, 12.99038105676661736 ) ) ;
#11063=DIRECTION ( 'NONE',  ( -0.1566598588826321192, 0.9876526153536342445, 7.798540720466731404E-17 ) ) ;
#11066=DIRECTION ( 'NONE',  ( -0.1566598588826321747, 0.9876526153536343555, 0.000000000000000000 ) ) ;
#11067=FACE_BOUND ( 'NONE', #16470, .T. ) ;
#11068=DIRECTION ( 'NONE',  ( -0.1566598588826321192, 0.9876526153536342445, 7.798540720466731404E-17 ) ) ;
#11069=CIRCLE ( 'NONE', #17462, 2.000000000000000000 ) ;
#11070=EDGE_CURVE ( 'NONE', #16672, #1209, #18188, .T. ) ;
#11072=DIRECTION ( 'NONE',  ( -0.1566598588826321192, 0.9876526153536342445, 7.798540720466731404E-17 ) ) ;
#11073=EDGE_LOOP ( 'NONE', ( #7884, #4911, #17383, #4585 ) ) ;
#11074=CIRCLE ( 'NONE', #16549, 1.500000000000001332 ) ;
#11076=EDGE_CURVE ( 'NONE', #8123, #14703, #4775, .T. ) ;
#11077=ORIENTED_EDGE ( 'NONE', *, *, #10531, .F. ) ;
#11079=ORIENTED_EDGE ( 'NONE', *, *, #17095, .T. ) ;
#11080=FACE_BOUND ( 'NONE', #10889, .T. ) ;
#11081=AXIS2_PLACEMENT_3D ( 'NONE', #12975, #15921, #18726 ) ;
#11082=EDGE_LOOP ( 'NONE', ( #5973, #16763, #17693, #15671 ) ) ;
#11083=AXIS2_PLACEMENT_3D ( 'NONE', #7548, #10563, #3257 ) ;
#11084=CARTESIAN_POINT ( 'NONE',  ( -48.02252708097942246, -27.86704125135829813, -17.32050807568878170 ) ) ;
#11085=AXIS2_PLACEMENT_3D ( 'NONE', #6070, #7401, #16012 ) ;
#11087=FACE_OUTER_BOUND ( 'NONE', #3121, .T. ) ;
#11088=VECTOR ( 'NONE', #14940, 1000.000000000000000 ) ;
#11089=DIRECTION ( 'NONE',  ( -0.1566598588826321192, 0.9876526153536342445, 7.798540720466731404E-17 ) ) ;
#11090=DIRECTION ( 'NONE',  ( -0.1566598588826321192, 0.9876526153536342445, 7.798540720466730171E-17 ) ) ;
#11091=ADVANCED_FACE ( 'NONE', ( #9520 ), #9982, .T. ) ;
#11092=VERTEX_POINT ( 'NONE', #16213 ) ;
#11093=DIRECTION ( 'NONE',  ( -0.9876526153536336894, -0.1566598588826350336, 0.000000000000000000 ) ) ;
#11095=DIRECTION ( 'NONE',  ( -0.9876526153536336894, -0.1566598588826349503, 0.000000000000000000 ) ) ;
#11096=EDGE_CURVE ( 'NONE', #15378, #14170, #4641, .T. ) ;
#11098=EDGE_LOOP ( 'NONE', ( #5559, #14389, #7464, #3512 ) ) ;
#11099=ORIENTED_EDGE ( 'NONE', *, *, #1612, .T. ) ;
#11100=DIRECTION ( 'NONE',  ( -0.1566598588826321192, 0.9876526153536342445, 7.798540720466730171E-17 ) ) ;
#11101=CIRCLE ( 'NONE', #18732, 1.500000000000000888 ) ;
#11102=VERTEX_POINT ( 'NONE', #11481 ) ;
#11105=CIRCLE ( 'NONE', #2937, 1.500000000000001332 ) ;
#11108=CARTESIAN_POINT ( 'NONE',  ( -33.16810284049712010, -83.21632480446695013, -12.99038105676658539 ) ) ;
#11109=CYLINDRICAL_SURFACE ( 'NONE', #2730, 1.500000000000001554 ) ;
#11112=VECTOR ( 'NONE', #16800, 1000.000000000000000 ) ;
#11113=DIRECTION ( 'NONE',  ( -0.1566598588826321747, 0.9876526153536343555, 0.000000000000000000 ) ) ;
#11114=DIRECTION ( 'NONE',  ( -0.1566598588826321747, 0.9876526153536343555, 0.000000000000000000 ) ) ;
#11115=EDGE_CURVE ( 'NONE', #1326, #1662, #7519, .T. ) ;
#11116=EDGE_LOOP ( 'NONE', ( #12627, #4694, #12384, #9065 ) ) ;
#11117=ORIENTED_EDGE ( 'NONE', *, *, #13796, .F. ) ;
#11118=FACE_BOUND ( 'NONE', #6903, .T. ) ;
#11119=DIRECTION ( 'NONE',  ( -0.1566598588826321192, 0.9876526153536342445, 7.798540720466730171E-17 ) ) ;
#11120=EDGE_LOOP ( 'NONE', ( #4905, #15283, #8471, #13688 ) ) ;
#11121=ORIENTED_EDGE ( 'NONE', *, *, #3055, .T. ) ;
#11122=EDGE_CURVE ( 'NONE', #8055, #13293, #7596, .T. ) ;
#11125=CARTESIAN_POINT ( 'NONE',  ( -1.109027851681966492, -20.42569795443330349, -12.99038105676658361 ) ) ;
#11126=VERTEX_POINT ( 'NONE', #16305 ) ;
#11127=DIRECTION ( 'NONE',  ( -0.1566598588826321192, 0.9876526153536342445, 7.798540720466731404E-17 ) ) ;
#11128=VECTOR ( 'NONE', #14970, 1000.000000000000000 ) ;
#11129=AXIS2_PLACEMENT_3D ( 'NONE', #11328, #1236, #7198 ) ;
#11130=DIRECTION ( 'NONE',  ( -0.1566598588826321192, 0.9876526153536342445, 7.798540720466730171E-17 ) ) ;
#11131=CIRCLE ( 'NONE', #2675, 2.000000000000000000 ) ;
#11132=EDGE_LOOP ( 'NONE', ( #97, #1945 ) ) ;
#11133=CARTESIAN_POINT ( 'NONE',  ( -57.36559191666103175, -87.05449134709141390, -17.32050807568878525 ) ) ;
#11134=DIRECTION ( 'NONE',  ( -0.1566598588826321192, 0.9876526153536342445, 7.798540720466730171E-17 ) ) ;
#11136=CYLINDRICAL_SURFACE ( 'NONE', #12984, 1.500000000000001554 ) ;
#11137=ORIENTED_EDGE ( 'NONE', *, *, #11680, .T. ) ;
#11138=VECTOR ( 'NONE', #16159, 1000.000000000000000 ) ;
#11139=CARTESIAN_POINT ( 'NONE',  ( -9.997901389864651378, -21.83563668437698269, -8.660254037844380193 ) ) ;
#11140=CIRCLE ( 'NONE', #2380, 1.500000000000001332 ) ;
#11141=DIRECTION ( 'NONE',  ( -0.9876526153536341335, -0.1566598588826327021, 0.000000000000000000 ) ) ;
#11142=ORIENTED_EDGE ( 'NONE', *, *, #8959, .T. ) ;
#11144=CIRCLE ( 'NONE', #13559, 1.500000000000000888 ) ;
#11148=ORIENTED_EDGE ( 'NONE', *, *, #6359, .F. ) ;
#11149=CARTESIAN_POINT ( 'NONE',  ( 7.819480696678551723, -76.71494066083772623, 4.330127018922207860 ) ) ;
#11150=VERTEX_POINT ( 'NONE', #7161 ) ;
#11152=ORIENTED_EDGE ( 'NONE', *, *, #9495, .T. ) ;
#11153=ADVANCED_FACE ( 'NONE', ( #1380 ), #3300, .F. ) ;
#11157=DIRECTION ( 'NONE',  ( -0.9876526153536336894, -0.1566598588826349503, 0.000000000000000000 ) ) ;
#11158=AXIS2_PLACEMENT_3D ( 'NONE', #5202, #12383, #9361 ) ;
#11161=DIRECTION ( 'NONE',  ( -0.9876526153536336894, -0.1566598588826349503, 0.000000000000000000 ) ) ;
#11162=ORIENTED_EDGE ( 'NONE', *, *, #6828, .T. ) ;
#11163=CARTESIAN_POINT ( 'NONE',  ( -72.50948914387967648, -26.68861478777333573, 21.65063509461101887 ) ) ;
#11164=FACE_BOUND ( 'NONE', #16785, .T. ) ;
#11165=AXIS2_PLACEMENT_3D ( 'NONE', #10922, #2399, #8194 ) ;
#11166=DIRECTION ( 'NONE',  ( -0.1566598588826321192, 0.9876526153536342445, 7.798540720466730171E-17 ) ) ;
#11167=AXIS2_PLACEMENT_3D ( 'NONE', #14887, #1909, #488 ) ;
#11168=DIRECTION ( 'NONE',  ( -0.9876526153536336894, -0.1566598588826349503, 0.000000000000000000 ) ) ;
#11171=VERTEX_POINT ( 'NONE', #14783 ) ;
#11172=VERTEX_POINT ( 'NONE', #8581 ) ;
#11174=CYLINDRICAL_SURFACE ( 'NONE', #10168, 2.500000000000002220 ) ;
#11175=FACE_BOUND ( 'NONE', #7489, .T. ) ;
#11177=ADVANCED_FACE ( 'NONE', ( #11299 ), #17115, .F. ) ;
#11180=VERTEX_POINT ( 'NONE', #10417 ) ;
#11181=AXIS2_PLACEMENT_3D ( 'NONE', #13558, #1731, #11929 ) ;
#11182=VECTOR ( 'NONE', #9642, 1000.000000000000000 ) ;
#11183=VERTEX_POINT ( 'NONE', #15777 ) ;
#11184=DIRECTION ( 'NONE',  ( -0.1566598588826321192, 0.9876526153536342445, 7.798540720466731404E-17 ) ) ;
#11185=EDGE_CURVE ( 'NONE', #13999, #6818, #3264, .T. ) ;
#11186=CARTESIAN_POINT ( 'NONE',  ( -10.94591899504043830, -79.69147797960773971, 1.424741226644455312E-14 ) ) ;
#11188=FACE_OUTER_BOUND ( 'NONE', #3141, .T. ) ;
#11189=CARTESIAN_POINT ( 'NONE',  ( -45.55339554259532520, -27.47539160415171722, 21.65063509461101887 ) ) ;
#11191=CARTESIAN_POINT ( 'NONE',  ( -2.057045456857756971, -78.28153924966404986, 12.99038105676660848 ) ) ;
#11192=AXIS2_PLACEMENT_3D ( 'NONE', #8464, #1450, #10059 ) ;
#11193=EDGE_LOOP ( 'NONE', ( #8153, #16270 ) ) ;
#11194=ORIENTED_EDGE ( 'NONE', *, *, #2847, .T. ) ;
#11196=VECTOR ( 'NONE', #15844, 1000.000000000000000 ) ;
#11197=CARTESIAN_POINT ( 'NONE',  ( -58.88670584986932965, -29.59029969906724844, -12.99038105676658006 ) ) ;
#11198=ORIENTED_EDGE ( 'NONE', *, *, #5339, .T. ) ;
#11199=ORIENTED_EDGE ( 'NONE', *, *, #12501, .T. ) ;
#11201=DIRECTION ( 'NONE',  ( -0.9876526153536341335, -0.1566598588826327021, 0.000000000000000000 ) ) ;
#11202=EDGE_CURVE ( 'NONE', #7608, #344, #1470, .T. ) ;
#11203=DIRECTION ( 'NONE',  ( -0.9876526153536341335, -0.1566598588826327021, 0.000000000000000000 ) ) ;
#11204=VERTEX_POINT ( 'NONE', #2690 ) ;
#11207=AXIS2_PLACEMENT_3D ( 'NONE', #7368, #2977, #17421 ) ;
#11208=VECTOR ( 'NONE', #441, 1000.000000000000000 ) ;
#11209=DIRECTION ( 'NONE',  ( -0.1566598588826321747, 0.9876526153536343555, 0.000000000000000000 ) ) ;
#11211=EDGE_CURVE ( 'NONE', #5059, #2873, #4182, .T. ) ;
#11214=CARTESIAN_POINT ( 'NONE',  ( -25.80034323552273179, -24.34219442649909126, -21.65063509461098334 ) ) ;
#11215=CIRCLE ( 'NONE', #5171, 1.500000000000001332 ) ;
#11216=DIRECTION ( 'NONE',  ( -0.1566598588826321192, 0.9876526153536342445, 7.798540720466731404E-17 ) ) ;
#11218=ORIENTED_EDGE ( 'NONE', *, *, #7688, .T. ) ;
#11219=FACE_BOUND ( 'NONE', #3766, .T. ) ;
#11220=CARTESIAN_POINT ( 'NONE',  ( -72.71384246482016067, -31.78353772342409300, 1.869203119972154228E-14 ) ) ;
#11221=ORIENTED_EDGE ( 'NONE', *, *, #12545, .F. ) ;
#11223=DIRECTION ( 'NONE',  ( -0.1566598588826321192, 0.9876526153536342445, 7.798540720466730171E-17 ) ) ;
#11224=CARTESIAN_POINT ( 'NONE',  ( -51.43967622453925514, -86.11453219379563961, 21.65063509461101532 ) ) ;
#11227=EDGE_CURVE ( 'NONE', #17592, #306, #6001, .T. ) ;
#11229=CARTESIAN_POINT ( 'NONE',  ( -71.02801022084922522, -26.45362499944938151, 4.330127018922218518 ) ) ;
#11230=EDGE_CURVE ( 'NONE', #15425, #16044, #15987, .T. ) ;
#11231=AXIS2_PLACEMENT_3D ( 'NONE', #6976, #5542, #11295 ) ;
#11232=ORIENTED_EDGE ( 'NONE', *, *, #3929, .T. ) ;
#11233=EDGE_CURVE ( 'NONE', #14533, #2476, #4197, .T. ) ;
#11235=ADVANCED_FACE ( 'NONE', ( #3574 ), #16801, .F. ) ;
#11236=FACE_OUTER_BOUND ( 'NONE', #1288, .T. ) ;
#11239=CIRCLE ( 'NONE', #3667, 1.500000000000000444 ) ;
#11240=DIRECTION ( 'NONE',  ( -0.1566598588826321192, 0.9876526153536342445, 7.798540720466730171E-17 ) ) ;
#11241=DIRECTION ( 'NONE',  ( -0.1566598588826321192, 0.9876526153536342445, 7.798540720466731404E-17 ) ) ;
#11243=CARTESIAN_POINT ( 'NONE',  ( -73.70149508017377116, -31.94019758230671258, 4.330127018922217630 ) ) ;
#11244=EDGE_LOOP ( 'NONE', ( #3109, #7969, #5927, #17247 ) ) ;
#11245=AXIS2_PLACEMENT_3D ( 'NONE', #16697, #4725, #4821 ) ;
#11247=CARTESIAN_POINT ( 'NONE',  ( -34.19539046602857724, -25.67380322700145356, 21.65063509461101887 ) ) ;
#11248=DIRECTION ( 'NONE',  ( -0.1566598588826321192, 0.9876526153536342445, 7.798540720466731404E-17 ) ) ;
#11249=EDGE_LOOP ( 'NONE', ( #17029, #17655, #16873, #869 ) ) ;
#11252=CIRCLE ( 'NONE', #9763, 1.500000000000001332 ) ;
#11253=CARTESIAN_POINT ( 'NONE',  ( -52.26261052913025651, -23.47708768067938578, 8.660254037844417496 ) ) ;
#11254=ORIENTED_EDGE ( 'NONE', *, *, #5614, .T. ) ;
#11255=FACE_OUTER_BOUND ( 'NONE', #13242, .T. ) ;
#11256=CIRCLE ( 'NONE', #1293, 1.500000000000000888 ) ;
#11258=DIRECTION ( 'NONE',  ( -0.1566598588826321192, 0.9876526153536342445, 7.798540720466731404E-17 ) ) ;
#11261=CYLINDRICAL_SURFACE ( 'NONE', #363, 1.500000000000000666 ) ;
#11267=LINE ( 'NONE', #12872, #16904 ) ;
#11268=EDGE_LOOP ( 'NONE', ( #13240, #17938 ) ) ;
#11269=EDGE_LOOP ( 'NONE', ( #14795, #5495 ) ) ;
#11270=DIRECTION ( 'NONE',  ( -0.9876526153536341335, -0.1566598588826327021, 0.000000000000000000 ) ) ;
#11274=ORIENTED_EDGE ( 'NONE', *, *, #15392, .F. ) ;
#11275=CARTESIAN_POINT ( 'NONE',  ( -61.84966369593023927, -30.06027927571514624, -21.65063509461098334 ) ) ;
#11277=FACE_BOUND ( 'NONE', #9238, .T. ) ;
#11278=DIRECTION ( 'NONE',  ( -0.1566598588826321192, 0.9876526153536342445, 7.798540720466730171E-17 ) ) ;
#11279=AXIS2_PLACEMENT_3D ( 'NONE', #1443, #10231, #3032 ) ;
#11280=DIRECTION ( 'NONE',  ( -0.1566598588826321192, 0.9876526153536342445, 7.798540720466731404E-17 ) ) ;
#11281=EDGE_CURVE ( 'NONE', #17456, #15676, #5218, .T. ) ;
#11282=DIRECTION ( 'NONE',  ( -0.9876526153536336894, -0.1566598588826350336, 0.000000000000000000 ) ) ;
#11283=DIRECTION ( 'NONE',  ( -0.1566598588826321192, 0.9876526153536342445, 7.798540720466730171E-17 ) ) ;
#11284=FACE_OUTER_BOUND ( 'NONE', #7854, .T. ) ;
#11285=DIRECTION ( 'NONE',  ( 0.000000000000000000, 0.000000000000000000, 1.000000000000000000 ) ) ;
#11286=LINE ( 'NONE', #17105, #5421 ) ;
#11287=EDGE_CURVE ( 'NONE', #4611, #7789, #16299, .T. ) ;
#11288=ORIENTED_EDGE ( 'NONE', *, *, #17153, .T. ) ;
#11289=EDGE_LOOP ( 'NONE', ( #7832, #14430 ) ) ;
#11290=ORIENTED_EDGE ( 'NONE', *, *, #8262, .T. ) ;
#11291=FACE_OUTER_BOUND ( 'NONE', #4847, .T. ) ;
#11292=VECTOR ( 'NONE', #1774, 1000.000000000000000 ) ;
#11293=VERTEX_POINT ( 'NONE', #16493 ) ;
#11295=DIRECTION ( 'NONE',  ( -0.9876526153536341335, -0.1566598588826327021, 0.000000000000000000 ) ) ;
#11296=CARTESIAN_POINT ( 'NONE',  ( -35.63723437888118184, -83.60797445167352748, 17.32050807568881368 ) ) ;
#11297=ORIENTED_EDGE ( 'NONE', *, *, #8503, .T. ) ;
#11298=PRODUCT_DEFINITION_CONTEXT ( 'detailed design', #13654, 'design' ) ;
#11299=FACE_OUTER_BOUND ( 'NONE', #11401, .T. ) ;
#11301=CARTESIAN_POINT ( 'NONE',  ( -36.62488699423479943, -83.76463431055617548, 4.330127018922213189 ) ) ;
#11303=DIRECTION ( 'NONE',  ( -0.9876526153536341335, -0.1566598588826327021, 0.000000000000000000 ) ) ;
#11304=DIRECTION ( 'NONE',  ( -0.9876526153536341335, -0.1566598588826327021, 0.000000000000000000 ) ) ;
#11306=ORIENTED_EDGE ( 'NONE', *, *, #16111, .F. ) ;
#11307=DIRECTION ( 'NONE',  ( -0.9876526153536341335, -0.1566598588826327576, 0.000000000000000000 ) ) ;
#11308=CARTESIAN_POINT ( 'NONE',  ( -17.69476899175320739, -17.99399261978727438, 17.32050807568881012 ) ) ;
#11309=ORIENTED_EDGE ( 'NONE', *, *, #191, .F. ) ;
#11311=LINE ( 'NONE', #17130, #2711 ) ;
#11312=ORIENTED_EDGE ( 'NONE', *, *, #8184, .T. ) ;
#11314=EDGE_CURVE ( 'NONE', #5645, #16215, #18769, .T. ) ;
#11318=CARTESIAN_POINT ( 'NONE',  ( -81.73462711737164454, 33.01666666666666572, 35.00000000000000000 ) ) ;
#11319=DIRECTION ( 'NONE',  ( -0.9876526153536341335, -0.1566598588826327021, 0.000000000000000000 ) ) ;
#11320=VERTEX_POINT ( 'NONE', #5105 ) ;
#11321=CARTESIAN_POINT ( 'NONE',  ( -34.15575545585073058, -83.37298466334958391, 1.424741226644455312E-14 ) ) ;
#11322=ORIENTED_EDGE ( 'NONE', *, *, #10082, .T. ) ;
#11323=CARTESIAN_POINT ( 'NONE',  ( -40.61513246582718750, -26.69209230973856251, -21.65063509461098334 ) ) ;
#11324=DIRECTION ( 'NONE',  ( 0.000000000000000000, 0.000000000000000000, 1.000000000000000000 ) ) ;
#11325=DIRECTION ( 'NONE',  ( -0.1566598588826321192, 0.9876526153536342445, 7.798540720466731404E-17 ) ) ;
#11326=VERTEX_POINT ( 'NONE', #7691 ) ;
#11328=CARTESIAN_POINT ( 'NONE',  ( -48.97054468615517919, -85.72288254658906226, 17.32050807568881368 ) ) ;
#11329=ORIENTED_EDGE ( 'NONE', *, *, #15337, .F. ) ;
#11331=EDGE_CURVE ( 'NONE', #15461, #11513, #18463, .T. ) ;
#11332=DIRECTION ( 'NONE',  ( -0.1566598588826321747, 0.9876526153536343555, 0.000000000000000000 ) ) ;
#11333=CIRCLE ( 'NONE', #14988, 1.500000000000000444 ) ;
#11335=EDGE_LOOP ( 'NONE', ( #12797, #4008 ) ) ;
#11336=ORIENTED_EDGE ( 'NONE', *, *, #6440, .T. ) ;
#11337=EDGE_CURVE ( 'NONE', #1532, #16572, #7870, .T. ) ;
#11338=VERTEX_POINT ( 'NONE', #6272 ) ;
#11339=CARTESIAN_POINT ( 'NONE',  ( -62.30385499342917655, -87.83779064150458282, 8.660254037844412167 ) ) ;
#11342=LINE ( 'NONE', #14312, #4929 ) ;
#11343=DIRECTION ( 'NONE',  ( 0.000000000000000000, 0.000000000000000000, 1.000000000000000000 ) ) ;
#11344=CARTESIAN_POINT ( 'NONE',  ( -6.995308533625909320, -79.06483854407721878, -4.330127018922185655 ) ) ;
#11345=CARTESIAN_POINT ( 'NONE',  ( -30.53425299135042081, -20.03057078526147805, -8.660254037844380193 ) ) ;
#11346=DIRECTION ( 'NONE',  ( -0.9876526153536336894, -0.1566598588826349503, 0.000000000000000000 ) ) ;
#11347=CIRCLE ( 'NONE', #6543, 1.500000000000000888 ) ;
#11348=CARTESIAN_POINT ( 'NONE',  ( -14.44233815895597672, -22.54060604934882051, 4.330127018922217630 ) ) ;
#11350=DIRECTION ( 'NONE',  ( -0.9876526153536336894, -0.1566598588826349503, 0.000000000000000000 ) ) ;
#11352=EDGE_CURVE ( 'NONE', #17569, #8605, #4479, .T. ) ;
#11353=EDGE_CURVE ( 'NONE', #9249, #10116, #3392, .T. ) ;
#11354=ORIENTED_EDGE ( 'NONE', *, *, #5902, .F. ) ;
#11356=LINE ( 'NONE', #17177, #8456 ) ;
#11358=ORIENTED_EDGE ( 'NONE', *, *, #14049, .T. ) ;
#11361=DIRECTION ( 'NONE',  ( -0.1566598588826321192, 0.9876526153536342445, 7.798540720466730171E-17 ) ) ;
#11362=VECTOR ( 'NONE', #4529, 1000.000000000000000 ) ;
#11364=CYLINDRICAL_SURFACE ( 'NONE', #12453, 1.500000000000001554 ) ;
#11365=EDGE_CURVE ( 'NONE', #17063, #4741, #1986, .T. ) ;
#11366=CARTESIAN_POINT ( 'NONE',  ( 0.000000000000000000, 0.000000000000000000, 24.99999999999999289 ) ) ;
#11367=ORIENTED_EDGE ( 'NONE', *, *, #10860, .F. ) ;
#11368=FACE_BOUND ( 'NONE', #10704, .T. ) ;
#11369=EDGE_LOOP ( 'NONE', ( #16647, #2542, #3607, #8904, #9292, #13323, #4806 ) ) ;
#11370=CARTESIAN_POINT ( 'NONE',  ( -19.87442754340095519, -23.40223527320329922, 8.660254037844417496 ) ) ;
#11372=CIRCLE ( 'NONE', #2010, 1.500000000000001332 ) ;
#11373=CARTESIAN_POINT ( 'NONE',  ( -34.15575545585073058, -83.37298466334958391, 17.32050807568881368 ) ) ;
#11374=DIRECTION ( 'NONE',  ( -0.9876526153536344665, -0.1566598588826304539, 0.000000000000000000 ) ) ;
#11376=CYLINDRICAL_SURFACE ( 'NONE', #6634, 1.500000000000001554 ) ;
#11377=VERTEX_POINT ( 'NONE', #677 ) ;
#11379=VERTEX_POINT ( 'NONE', #15163 ) ;
#11380=DIRECTION ( 'NONE',  ( -0.1566598588826321192, 0.9876526153536342445, 7.798540720466730171E-17 ) ) ;
#11382=ORIENTED_EDGE ( 'NONE', *, *, #6193, .T. ) ;
#11384=EDGE_CURVE ( 'NONE', #17992, #983, #2060, .T. ) ;
#11385=CARTESIAN_POINT ( 'NONE',  ( -44.56574292724170760, -27.31873174526908699, 17.32050807568881723 ) ) ;
#11388=PLANE ( 'NONE',  #2774 ) ;
#11389=EDGE_CURVE ( 'NONE', #14949, #8287, #1182, .T. ) ;
#11390=CIRCLE ( 'NONE', #4447, 1.500000000000000444 ) ;
#11391=DIRECTION ( 'NONE',  ( 0.000000000000000000, 0.000000000000000000, 1.000000000000000000 ) ) ;
#11392=CARTESIAN_POINT ( 'NONE',  ( -41.56315007100294423, -84.54793360496931598, 12.99038105676661203 ) ) ;
#11393=CYLINDRICAL_SURFACE ( 'NONE', #11772, 1.500000000000001554 ) ;
#11395=DIRECTION ( 'NONE',  ( -0.9876526153536341335, -0.1566598588826327021, 0.000000000000000000 ) ) ;
#11396=CARTESIAN_POINT ( 'NONE',  ( -20.16390053013728334, -18.38564226699384463, -21.65063509461098334 ) ) ;
#11397=LINE ( 'NONE', #10358, #6847 ) ;
#11400=DIRECTION ( 'NONE',  ( -0.1566598588826321192, 0.9876526153536342445, 7.798540720466730171E-17 ) ) ;
#11401=EDGE_LOOP ( 'NONE', ( #12210, #16538, #11745, #14774 ) ) ;
#11404=DIRECTION ( 'NONE',  ( -0.1566598588826321747, 0.9876526153536343555, 0.000000000000000000 ) ) ;
#11405=EDGE_LOOP ( 'NONE', ( #7344, #10189 ) ) ;
#11406=CARTESIAN_POINT ( 'NONE',  ( -0.4108482230646692823, -15.25244508934120802, -4.330127018922183879 ) ) ;
#11407=CARTESIAN_POINT ( 'NONE',  ( -51.43967622453926936, -86.11453219379563961, -4.330127018922185655 ) ) ;
#11410=CYLINDRICAL_SURFACE ( 'NONE', #2356, 1.500000000000001554 ) ;
#11412=AXIS2_PLACEMENT_3D ( 'NONE', #3072, #8865, #14646 ) ;
#11414=ORIENTED_EDGE ( 'NONE', *, *, #18466, .T. ) ;
#11416=ADVANCED_FACE ( 'NONE', ( #9770 ), #12868, .F. ) ;
#11417=CARTESIAN_POINT ( 'NONE',  ( -33.99103714508810725, -20.57888029135069274, 1.908195823574487804E-14 ) ) ;
#11420=DIRECTION ( 'NONE',  ( -0.1566598588826321192, 0.9876526153536342445, 7.798540720466730171E-17 ) ) ;
#11421=AXIS2_PLACEMENT_3D ( 'NONE', #6351, #9358, #3463 ) ;
#11422=EDGE_CURVE ( 'NONE', #14703, #8123, #8450, .T. ) ;
#11423=LINE ( 'NONE', #6920, #13834 ) ;
#11424=DIRECTION ( 'NONE',  ( -0.1566598588826321192, 0.9876526153536342445, 7.798540720466730171E-17 ) ) ;
#11425=ORIENTED_EDGE ( 'NONE', *, *, #6164, .T. ) ;
#11426=AXIS2_PLACEMENT_3D ( 'NONE', #13863, #12531, #8000 ) ;
#11427=FACE_OUTER_BOUND ( 'NONE', #10102, .T. ) ;
#11428=ORIENTED_EDGE ( 'NONE', *, *, #727, .T. ) ;
#11429=DIRECTION ( 'NONE',  ( -0.1566598588826321747, 0.9876526153536343555, 0.000000000000000000 ) ) ;
#11430=DIRECTION ( 'NONE',  ( -0.1566598588826321192, 0.9876526153536342445, 7.798540720466730171E-17 ) ) ;
#11431=CARTESIAN_POINT ( 'NONE',  ( -24.31886431249228053, -24.10720463817513703, -21.65063509461098334 ) ) ;
#11432=AXIS2_PLACEMENT_3D ( 'NONE', #12434, #6864, #10998 ) ;
#11433=LINE ( 'NONE', #4427, #3088 ) ;
#11434=CARTESIAN_POINT ( 'NONE',  ( -76.95392591297100182, -27.39358415274517711, 8.660254037844417496 ) ) ;
#11435=AXIS2_PLACEMENT_3D ( 'NONE', #6180, #10511, #5546 ) ;
#11436=ADVANCED_FACE ( 'NONE', ( #14109 ), #4049, .F. ) ;
#11437=CARTESIAN_POINT ( 'NONE',  ( -12.75650591498505371, -17.21069332537411256, -8.660254037844380193 ) ) ;
#11438=CIRCLE ( 'NONE', #12032, 2.500000000000002220 ) ;
#11440=AXIS2_PLACEMENT_3D ( 'NONE', #5688, #16104, #4252 ) ;
#11443=VERTEX_POINT ( 'NONE', #6835 ) ;
#11445=CARTESIAN_POINT ( 'NONE',  ( -45.55339554259532520, -27.47539160415171722, 12.99038105676661736 ) ) ;
#11446=CIRCLE ( 'NONE', #13876, 1.499999999999999556 ) ;
#11448=ORIENTED_EDGE ( 'NONE', *, *, #18162, .F. ) ;
#11449=DIRECTION ( 'NONE',  ( -0.9876526153536341335, -0.1566598588826327021, 0.000000000000000000 ) ) ;
#11451=ORIENTED_EDGE ( 'NONE', *, *, #4367, .F. ) ;
#11452=CIRCLE ( 'NONE', #15718, 1.500000000000000000 ) ;
#11453=FACE_BOUND ( 'NONE', #16593, .T. ) ;
#11454=ORIENTED_EDGE ( 'NONE', *, *, #9898, .F. ) ;
#11455=ADVANCED_FACE ( 'NONE', ( #14210 ), #18533, .F. ) ;
#11456=VECTOR ( 'NONE', #14097, 1000.000000000000000 ) ;
#11457=EDGE_CURVE ( 'NONE', #13719, #2279, #17838, .T. ) ;
#11459=ORIENTED_EDGE ( 'NONE', *, *, #15667, .T. ) ;
#11460=AXIS2_PLACEMENT_3D ( 'NONE', #5857, #2817, #14380 ) ;
#11461=VERTEX_POINT ( 'NONE', #17275 ) ;
#11462=DIRECTION ( 'NONE',  ( -0.9876526153536336894, -0.1566598588826349503, 0.000000000000000000 ) ) ;
#11463=CIRCLE ( 'NONE', #1216, 1.500000000000000888 ) ;
#11464=VECTOR ( 'NONE', #8808, 1000.000000000000000 ) ;
#11465=AXIS2_PLACEMENT_3D ( 'NONE', #11774, #2813, #16171 ) ;
#11466=CARTESIAN_POINT ( 'NONE',  ( -20.86208015875458344, -23.55889513208593655, -4.330127018922181215 ) ) ;
#11468=DIRECTION ( 'NONE',  ( -0.1566598588826321192, 0.9876526153536342445, 7.798540720466731404E-17 ) ) ;
#11469=ORIENTED_EDGE ( 'NONE', *, *, #4293, .F. ) ;
#11470=VERTEX_POINT ( 'NONE', #7039 ) ;
#11472=VERTEX_POINT ( 'NONE', #2357 ) ;
#11474=CIRCLE ( 'NONE', #6044, 1.500000000000000000 ) ;
#11476=VECTOR ( 'NONE', #18166, 1000.000000000000000 ) ;
#11478=CARTESIAN_POINT ( 'NONE',  ( -65.30644784966793281, -30.60858878180435738, -21.65063509461098334 ) ) ;
#11479=AXIS2_PLACEMENT_3D ( 'NONE', #17337, #14081, #10095 ) ;
#11480=DIRECTION ( 'NONE',  ( -0.1566598588826321192, 0.9876526153536342445, 7.798540720466730171E-17 ) ) ;
#11481=CARTESIAN_POINT ( 'NONE',  ( -9.504075082187826595, -21.75730675493566579, -21.65063509461098334 ) ) ;
#11482=SHAPE_DEFINITION_REPRESENTATION ( #11041, #6739 ) ;
#11485=CIRCLE ( 'NONE', #8186, 1.500000000000001332 ) ;
#11486=FACE_OUTER_BOUND ( 'NONE', #11369, .T. ) ;
#11487=EDGE_CURVE ( 'NONE', #2990, #8008, #9650, .T. ) ;
#11490=ORIENTED_EDGE ( 'NONE', *, *, #15768, .T. ) ;
#11491=EDGE_CURVE ( 'NONE', #14533, #9448, #13557, .T. ) ;
#11492=ORIENTED_EDGE ( 'NONE', *, *, #1080, .F. ) ;
#11493=FACE_OUTER_BOUND ( 'NONE', #9247, .T. ) ;
#11494=ORIENTED_EDGE ( 'NONE', *, *, #17129, .T. ) ;
#11496=DIRECTION ( 'NONE',  ( -0.1566598588826321192, 0.9876526153536342445, 7.798540720466731404E-17 ) ) ;
#11497=DIRECTION ( 'NONE',  ( -0.1566598588826321192, 0.9876526153536342445, 7.798540720466730171E-17 ) ) ;
#11499=VERTEX_POINT ( 'NONE', #11345 ) ;
#11500=DIRECTION ( 'NONE',  ( 0.000000000000000000, 0.000000000000000000, 1.000000000000000000 ) ) ;
#11501=CIRCLE ( 'NONE', #3327, 1.499999999999999556 ) ;
#11502=CIRCLE ( 'NONE', #12724, 1.500000000000000444 ) ;
#11503=CARTESIAN_POINT ( 'NONE',  ( -11.97320662057189899, -22.14895640214223960, -17.32050807568878170 ) ) ;
#11506=CARTESIAN_POINT ( 'NONE',  ( -75.96627329761737712, -27.23692429386253622, -4.330127018922180326 ) ) ;
#11507=CIRCLE ( 'NONE', #14560, 1.500000000000001332 ) ;
#11508=CARTESIAN_POINT ( 'NONE',  ( -51.47931123471711601, -28.41535075744751282, -17.32050807568878170 ) ) ;
#11509=CARTESIAN_POINT ( 'NONE',  ( -29.21749237908259644, -82.58968536893641499, -17.32050807568878525 ) ) ;
#11511=LINE ( 'NONE', #14840, #7433 ) ;
#11512=CARTESIAN_POINT ( 'NONE',  ( -46.33669483700848701, -22.53712852738358663, -4.330127018922180326 ) ) ;
#11513=VERTEX_POINT ( 'NONE', #7123 ) ;
#11514=DIRECTION ( 'NONE',  ( -0.1566598588826321192, 0.9876526153536342445, 7.798540720466730171E-17 ) ) ;
#11515=AXIS2_PLACEMENT_3D ( 'NONE', #3814, #926, #8208 ) ;
#11516=DIRECTION ( 'NONE',  ( -0.1566598588826321192, 0.9876526153536342445, 7.798540720466730171E-17 ) ) ;
#11517=ORIENTED_EDGE ( 'NONE', *, *, #16634, .F. ) ;
#11518=CIRCLE ( 'NONE', #7327, 1.500000000000000888 ) ;
#11520=DIRECTION ( 'NONE',  ( -0.1566598588826321192, 0.9876526153536342445, 7.798540720466730171E-17 ) ) ;
#11522=VECTOR ( 'NONE', #16834, 1000.000000000000000 ) ;
#11523=DIRECTION ( 'NONE',  ( -0.1566598588826321192, 0.9876526153536342445, 7.798540720466730171E-17 ) ) ;
#11524=EDGE_CURVE ( 'NONE', #11126, #8986, #5505, .T. ) ;
#11526=CIRCLE ( 'NONE', #6424, 1.500000000000001332 ) ;
#11527=CARTESIAN_POINT ( 'NONE',  ( -77.44775222064782838, -27.47191408218649045, 12.99038105676661736 ) ) ;
#11528=DIRECTION ( 'NONE',  ( -0.1566598588826321192, 0.9876526153536342445, 7.798540720466730171E-17 ) ) ;
#11529=ORIENTED_EDGE ( 'NONE', *, *, #5114, .F. ) ;
#11531=FACE_OUTER_BOUND ( 'NONE', #10441, .T. ) ;
#11533=CARTESIAN_POINT ( 'NONE',  ( -50.49165861936349131, -28.25869089856488614, -12.99038105676658006 ) ) ;
#11534=DIRECTION ( 'NONE',  ( -0.9876526153536336894, -0.1566598588826349503, 0.000000000000000000 ) ) ;
#11535=FACE_BOUND ( 'NONE', #13534, .T. ) ;
#11536=FACE_OUTER_BOUND ( 'NONE', #18745, .T. ) ;
#11539=ORIENTED_EDGE ( 'NONE', *, *, #5862, .T. ) ;
#11540=DIRECTION ( 'NONE',  ( -0.1566598588826321747, 0.9876526153536343555, 0.000000000000000000 ) ) ;
#11542=EDGE_LOOP ( 'NONE', ( #7488, #15805, #8802, #15052 ) ) ;
#11543=VERTEX_POINT ( 'NONE', #11437 ) ;
#11545=CARTESIAN_POINT ( 'NONE',  ( -41.39843176024032800, -21.75382923297043547, 12.99038105676661736 ) ) ;
#11546=VECTOR ( 'NONE', #18105, 1000.000000000000000 ) ;
#11548=ORIENTED_EDGE ( 'NONE', *, *, #12756, .F. ) ;
#11549=FACE_BOUND ( 'NONE', #9113, .T. ) ;
#11550=ADVANCED_FACE ( 'NONE', ( #17080 ), #8149, .F. ) ;
#11551=CARTESIAN_POINT ( 'NONE',  ( -57.85941822433786541, -87.13282127653273790, -4.330127018922185655 ) ) ;
#11552=CARTESIAN_POINT ( 'NONE',  ( -29.05277406831996245, -19.79558099693753093, -8.660254037844380193 ) ) ;
#11553=ORIENTED_EDGE ( 'NONE', *, *, #10577, .F. ) ;
#11554=CIRCLE ( 'NONE', #13990, 1.499999999999999556 ) ;
#11555=FACE_OUTER_BOUND ( 'NONE', #13946, .T. ) ;
#11556=ORIENTED_EDGE ( 'NONE', *, *, #11791, .T. ) ;
#11557=FACE_BOUND ( 'NONE', #8597, .T. ) ;
#11558=CARTESIAN_POINT ( 'NONE',  ( 0.000000000000000000, 0.000000000000000000, -30.00000000000000000 ) ) ;
#11559=AXIS2_PLACEMENT_3D ( 'NONE', #5890, #5710, #4547 ) ;
#11560=DIRECTION ( 'NONE',  ( -0.9876526153536336894, -0.1566598588826349503, 0.000000000000000000 ) ) ;
#11562=CARTESIAN_POINT ( 'NONE',  ( 2.881217619910392269, -77.49823995525089515, -12.99038105676658539 ) ) ;
#11564=FACE_BOUND ( 'NONE', #9009, .T. ) ;
#11565=DIRECTION ( 'NONE',  ( 0.000000000000000000, 0.000000000000000000, 1.000000000000000000 ) ) ;
#11567=EDGE_LOOP ( 'NONE', ( #1794, #2792 ) ) ;
#11568=EDGE_LOOP ( 'NONE', ( #11606, #15329, #11290, #7253 ) ) ;
#11569=ORIENTED_EDGE ( 'NONE', *, *, #7054, .F. ) ;
#11570=DIRECTION ( 'NONE',  ( -0.1566598588826321192, 0.9876526153536342445, 7.798540720466730171E-17 ) ) ;
#11571=EDGE_CURVE ( 'NONE', #10712, #11171, #1488, .T. ) ;
#11572=EDGE_CURVE ( 'NONE', #17136, #6756, #7537, .T. ) ;
#11573=ORIENTED_EDGE ( 'NONE', *, *, #14660, .T. ) ;
#11574=CARTESIAN_POINT ( 'NONE',  ( -61.84966369593024638, -30.06027927571514624, -4.330127018922181215 ) ) ;
#11575=EDGE_CURVE ( 'NONE', #17944, #10450, #12578, .T. ) ;
#11576=DIRECTION ( 'NONE',  ( -0.9876526153536341335, -0.1566598588826327021, 0.000000000000000000 ) ) ;
#11577=CIRCLE ( 'NONE', #8276, 1.499999999999999556 ) ;
#11578=EDGE_CURVE ( 'NONE', #17378, #4142, #175, .T. ) ;
#11580=CARTESIAN_POINT ( 'NONE',  ( -49.95819730150881099, -85.87954240547168183, -4.330127018922185655 ) ) ;
#11581=CARTESIAN_POINT ( 'NONE',  ( -3.044698072211382112, -78.43819910854666944, -8.660254037844385522 ) ) ;
#11583=VERTEX_POINT ( 'NONE', #7216 ) ;
#11585=CARTESIAN_POINT ( 'NONE',  ( -48.80582637539257718, -22.92877817459016043, -17.32050807568878170 ) ) ;
#11586=CARTESIAN_POINT ( 'NONE',  ( -36.46016868347218320, -20.97052993855727721, 12.99038105676661736 ) ) ;
#11588=VERTEX_POINT ( 'NONE', #11889 ) ;
#11589=ORIENTED_EDGE ( 'NONE', *, *, #2111, .T. ) ;
#11590=LINE ( 'NONE', #15964, #17232 ) ;
#11591=DIRECTION ( 'NONE',  ( -0.1566598588826321192, 0.9876526153536342445, 7.798540720466730171E-17 ) ) ;
#11593=EDGE_CURVE ( 'NONE', #18515, #1621, #14489, .T. ) ;
#11594=LINE ( 'NONE', #14917, #14814 ) ;
#11596=CARTESIAN_POINT ( 'NONE',  ( -20.16390053013728689, -18.38564226699385173, -4.330127018922180326 ) ) ;
#11598=EDGE_CURVE ( 'NONE', #12109, #11293, #5099, .T. ) ;
#11600=CARTESIAN_POINT ( 'NONE',  ( -39.62747985047356281, -26.53543245085591806, 17.32050807568881723 ) ) ;
#11601=CARTESIAN_POINT ( 'NONE',  ( -16.70711637639958269, -17.83733276090463704, 4.330127018922218518 ) ) ;
#11603=DIRECTION ( 'NONE',  ( -0.9876526153536341335, -0.1566598588826327021, 0.000000000000000000 ) ) ;
#11605=CARTESIAN_POINT ( 'NONE',  ( -15.71946376104596155, -17.68067290202199970, -17.32050807568878170 ) ) ;
#11606=ORIENTED_EDGE ( 'NONE', *, *, #8041, .F. ) ;
#11607=CARTESIAN_POINT ( 'NONE',  ( -30.69897130211303349, -82.82467515726037277, -8.660254037844385522 ) ) ;
#11608=DIRECTION ( 'NONE',  ( 0.000000000000000000, 0.000000000000000000, 1.000000000000000000 ) ) ;
#11609=VERTEX_POINT ( 'NONE', #4349 ) ;
#11610=CARTESIAN_POINT ( 'NONE',  ( -10.78120068427780964, -16.89737360760884144, 8.660254037844413944 ) ) ;
#11611=ORIENTED_EDGE ( 'NONE', *, *, #1147, .T. ) ;
#11612=CARTESIAN_POINT ( 'NONE',  ( -17.40529600501688279, -23.01058562599671831, -4.330127018922181215 ) ) ;
#11613=EDGE_CURVE ( 'NONE', #1459, #14963, #12958, .T. ) ;
#11614=DIRECTION ( 'NONE',  ( -0.1566598588826321747, 0.9876526153536343555, 0.000000000000000000 ) ) ;
#11616=LINE ( 'NONE', #5871, #10690 ) ;
#11617=CYLINDRICAL_SURFACE ( 'NONE', #16411, 1.500000000000000666 ) ;
#11619=EDGE_CURVE ( 'NONE', #12390, #8349, #7571, .T. ) ;
#11620=DIRECTION ( 'NONE',  ( -0.1566598588826321192, 0.9876526153536342445, 7.798540720466731404E-17 ) ) ;
#11621=VERTEX_POINT ( 'NONE', #8895 ) ;
#11622=FACE_OUTER_BOUND ( 'NONE', #14078, .T. ) ;
#11623=DIRECTION ( 'NONE',  ( -0.1566598588826321192, 0.9876526153536342445, 7.798540720466730171E-17 ) ) ;
#11625=CIRCLE ( 'NONE', #3451, 1.500000000000000888 ) ;
#11626=EDGE_LOOP ( 'NONE', ( #15379, #11054, #11079, #2349 ) ) ;
#11627=ORIENTED_EDGE ( 'NONE', *, *, #6269, .F. ) ;
#11629=ORIENTED_EDGE ( 'NONE', *, *, #4622, .T. ) ;
#11630=ORIENTED_EDGE ( 'NONE', *, *, #9854, .T. ) ;
#11631=DIRECTION ( 'NONE',  ( -0.1566598588826321192, 0.9876526153536342445, 7.798540720466730171E-17 ) ) ;
#11633=FACE_BOUND ( 'NONE', #2506, .T. ) ;
#11634=CARTESIAN_POINT ( 'NONE',  ( -2.057045456857756971, -78.28153924966404986, 12.99038105676660848 ) ) ;
#11635=ORIENTED_EDGE ( 'NONE', *, *, #358, .F. ) ;
#11637=EDGE_LOOP ( 'NONE', ( #18024, #6426 ) ) ;
#11639=ORIENTED_EDGE ( 'NONE', *, *, #16137, .F. ) ;
#11640=DIRECTION ( 'NONE',  ( -0.9876526153536336894, -0.1566598588826349503, 0.000000000000000000 ) ) ;
#11641=DIRECTION ( 'NONE',  ( -0.9876526153536336894, -0.1566598588826350336, 0.000000000000000000 ) ) ;
#11644=DIRECTION ( 'NONE',  ( -0.1566598588826321747, 0.9876526153536343555, 0.000000000000000000 ) ) ;
#11645=AXIS2_PLACEMENT_3D ( 'NONE', #3704, #18363, #1002 ) ;
#11646=ORIENTED_EDGE ( 'NONE', *, *, #16207, .T. ) ;
#11647=VERTEX_POINT ( 'NONE', #10393 ) ;
#11648=ORIENTED_EDGE ( 'NONE', *, *, #15922, .F. ) ;
#11649=EDGE_LOOP ( 'NONE', ( #819, #3710, #14975, #5607 ) ) ;
#11650=DIRECTION ( 'NONE',  ( -0.1566598588826321747, 0.9876526153536343555, 0.000000000000000000 ) ) ;
#11651=ORIENTED_EDGE ( 'NONE', *, *, #1419, .T. ) ;
#11652=DIRECTION ( 'NONE',  ( -0.1566598588826321192, 0.9876526153536342445, 7.798540720466730171E-17 ) ) ;
#11653=CARTESIAN_POINT ( 'NONE',  ( -9.997901389864651378, -21.83563668437698269, 8.660254037844413944 ) ) ;
#11654=ORIENTED_EDGE ( 'NONE', *, *, #8761, .T. ) ;
#11655=CIRCLE ( 'NONE', #16525, 1.500000000000000000 ) ;
#11657=DIRECTION ( 'NONE',  ( -0.9876526153536341335, -0.1566598588826327021, 0.000000000000000000 ) ) ;
#11658=EDGE_CURVE ( 'NONE', #10862, #8789, #18477, .T. ) ;
#11659=EDGE_CURVE ( 'NONE', #6405, #5249, #13338, .T. ) ;
#11661=LINE ( 'NONE', #16061, #14534 ) ;
#11662=ADVANCED_FACE ( 'NONE', ( #15905 ), #5955, .F. ) ;
#11663=DIRECTION ( 'NONE',  ( -0.1566598588826321747, 0.9876526153536343555, 0.000000000000000000 ) ) ;
#11664=ORIENTED_EDGE ( 'NONE', *, *, #18096, .F. ) ;
#11669=DIRECTION ( 'NONE',  ( 0.000000000000000000, 0.000000000000000000, 1.000000000000000000 ) ) ;
#11670=AXIS2_PLACEMENT_3D ( 'NONE', #14765, #3278, #9078 ) ;
#11671=VERTEX_POINT ( 'NONE', #2909 ) ;
#11672=VERTEX_POINT ( 'NONE', #14671 ) ;
#11673=DIRECTION ( 'NONE',  ( 0.000000000000000000, 0.000000000000000000, 1.000000000000000000 ) ) ;
#11675=DIRECTION ( 'NONE',  ( 0.000000000000000000, 0.000000000000000000, 1.000000000000000000 ) ) ;
#11676=AXIS2_PLACEMENT_3D ( 'NONE', #14120, #15632, #14329 ) ;
#11677=CARTESIAN_POINT ( 'NONE',  ( -44.56574292724170760, -27.31873174526908699, 8.660254037844417496 ) ) ;
#11678=FACE_OUTER_BOUND ( 'NONE', #3625, .T. ) ;
#11679=EDGE_CURVE ( 'NONE', #8810, #1168, #16315, .T. ) ;
#11680=EDGE_CURVE ( 'NONE', #11588, #15928, #11140, .T. ) ;
#11681=CARTESIAN_POINT ( 'NONE',  ( -31.68662391746665463, -82.98133501614300656, 21.65063509461101532 ) ) ;
#11682=AXIS2_PLACEMENT_3D ( 'NONE', #16261, #1948, #533 ) ;
#11683=CARTESIAN_POINT ( 'NONE',  ( 55.85952145814821534, 6.938893903907228378E-15, 30.00000000000000000 ) ) ;
#11684=VECTOR ( 'NONE', #14680, 1000.000000000000000 ) ;
#11685=CARTESIAN_POINT ( 'NONE',  ( -77.65210554158829837, -32.56683701783724416, 8.660254037844417496 ) ) ;
#11687=VERTEX_POINT ( 'NONE', #13060 ) ;
#11688=CARTESIAN_POINT ( 'NONE',  ( -57.69469991357524208, -24.33871690453384673, -12.99038105676658006 ) ) ;
#11689=ORIENTED_EDGE ( 'NONE', *, *, #7756, .T. ) ;
#11690=CIRCLE ( 'NONE', #8394, 1.500000000000001332 ) ;
#11691=ORIENTED_EDGE ( 'NONE', *, *, #6366, .F. ) ;
#11692=EDGE_CURVE ( 'NONE', #4161, #3161, #2975, .T. ) ;
#11693=ORIENTED_EDGE ( 'NONE', *, *, #6000, .F. ) ;
#11694=AXIS2_PLACEMENT_3D ( 'NONE', #663, #6450, #12186 ) ;
#11695=ORIENTED_EDGE ( 'NONE', *, *, #13598, .F. ) ;
#11696=CARTESIAN_POINT ( 'NONE',  ( -61.15148406731293562, -24.88702641062306142, -4.330127018922180326 ) ) ;
#11698=ORIENTED_EDGE ( 'NONE', *, *, #6747, .T. ) ;
#11699=LINE ( 'NONE', #8888, #18256 ) ;
#11701=FACE_OUTER_BOUND ( 'NONE', #9205, .T. ) ;
#11702=DIRECTION ( 'NONE',  ( -0.1566598588826321192, 0.9876526153536342445, 7.798540720466730171E-17 ) ) ;
#11703=CARTESIAN_POINT ( 'NONE',  ( -47.03487446562577645, -27.71038139247565368, 4.330127018922217630 ) ) ;
#11704=CYLINDRICAL_SURFACE ( 'NONE', #10047, 1.500000000000000666 ) ;
#11706=DIRECTION ( 'NONE',  ( -0.1566598588826321192, 0.9876526153536342445, 7.798540720466730171E-17 ) ) ;
#11708=FACE_OUTER_BOUND ( 'NONE', #11027, .T. ) ;
#11709=DIRECTION ( 'NONE',  ( 1.000000000000000000, 0.000000000000000000, -0.000000000000000000 ) ) ;
#11710=DIRECTION ( 'NONE',  ( -0.9876526153536336894, -0.1566598588826349503, 0.000000000000000000 ) ) ;
#11713=AXIS2_PLACEMENT_3D ( 'NONE', #12399, #13916, #16698 ) ;
#11714=ORIENTED_EDGE ( 'NONE', *, *, #9681, .T. ) ;
#11715=EDGE_CURVE ( 'NONE', #15259, #18385, #4705, .T. ) ;
#11717=ORIENTED_EDGE ( 'NONE', *, *, #6776, .F. ) ;
#11719=DIRECTION ( 'NONE',  ( 0.000000000000000000, 0.000000000000000000, 1.000000000000000000 ) ) ;
#11720=ADVANCED_FACE ( 'NONE', ( #16478 ), #10753, .F. ) ;
#11723=DIRECTION ( 'NONE',  ( -0.1566598588826321192, 0.9876526153536342445, 7.798540720466730171E-17 ) ) ;
#11724=VECTOR ( 'NONE', #3483, 1000.000000000000000 ) ;
#11725=CIRCLE ( 'NONE', #16619, 1.500000000000000888 ) ;
#11727=ORIENTED_EDGE ( 'NONE', *, *, #4633, .F. ) ;
#11728=DIRECTION ( 'NONE',  ( 0.000000000000000000, 0.000000000000000000, 1.000000000000000000 ) ) ;
#11729=ORIENTED_EDGE ( 'NONE', *, *, #2847, .F. ) ;
#11730=DIRECTION ( 'NONE',  ( -0.9876526153536344665, -0.1566598588826304539, 0.000000000000000000 ) ) ;
#11731=CIRCLE ( 'NONE', #16947, 1.499999999999999556 ) ;
#11732=CARTESIAN_POINT ( 'NONE',  ( -30.20514499443620338, -82.74634522781903456, -4.330127018922185655 ) ) ;
#11733=CIRCLE ( 'NONE', #3570, 1.500000000000000888 ) ;
#11734=DIRECTION ( 'NONE',  ( 0.000000000000000000, 0.000000000000000000, 1.000000000000000000 ) ) ;
#11735=EDGE_LOOP ( 'NONE', ( #1434, #17225 ) ) ;
#11736=CIRCLE ( 'NONE', #16003, 1.500000000000001332 ) ;
#11737=ORIENTED_EDGE ( 'NONE', *, *, #18785, .F. ) ;
#11742=VERTEX_POINT ( 'NONE', #3553 ) ;
#11743=CARTESIAN_POINT ( 'NONE',  ( -33.16810284049712010, -83.21632480446695013, -21.65063509461098690 ) ) ;
#11744=DIRECTION ( 'NONE',  ( -0.1566598588826321192, 0.9876526153536342445, 7.798540720466731404E-17 ) ) ;
#11745=ORIENTED_EDGE ( 'NONE', *, *, #7518, .T. ) ;
#11746=AXIS2_PLACEMENT_3D ( 'NONE', #13928, #981, #6753 ) ;
#11747=ORIENTED_EDGE ( 'NONE', *, *, #8633, .T. ) ;
#11748=EDGE_CURVE ( 'NONE', #13719, #3635, #13786, .T. ) ;
#11749=AXIS2_PLACEMENT_3D ( 'NONE', #7946, #656, #12081 ) ;
#11750=ORIENTED_EDGE ( 'NONE', *, *, #4671, .T. ) ;
#11751=ORIENTED_EDGE ( 'NONE', *, *, #3998, .T. ) ;
#11752=DIRECTION ( 'NONE',  ( -0.1566598588826321192, 0.9876526153536342445, 7.798540720466730171E-17 ) ) ;
#11754=DIRECTION ( 'NONE',  ( -0.1566598588826321747, 0.9876526153536343555, 0.000000000000000000 ) ) ;
#11755=AXIS2_PLACEMENT_3D ( 'NONE', #14921, #524, #12445 ) ;
#11757=ORIENTED_EDGE ( 'NONE', *, *, #12952, .F. ) ;
#11758=ORIENTED_EDGE ( 'NONE', *, *, #3719, .F. ) ;
#11759=CARTESIAN_POINT ( 'NONE',  ( -25.59598991458226536, -19.24727149084831979, -8.660254037844380193 ) ) ;
#11760=EDGE_CURVE ( 'NONE', #5727, #8327, #11733, .T. ) ;
#11763=DIRECTION ( 'NONE',  ( 0.000000000000000000, 0.000000000000000000, 1.000000000000000000 ) ) ;
#11764=CARTESIAN_POINT ( 'NONE',  ( -12.46703292824872733, -22.22728633158356359, 4.330127018922214077 ) ) ;
#11765=AXIS2_PLACEMENT_3D ( 'NONE', #10734, #532, #16460 ) ;
#11766=EDGE_CURVE ( 'NONE', #14764, #4082, #4975, .T. ) ;
#11767=CIRCLE ( 'NONE', #12063, 1.500000000000000888 ) ;
#11769=ORIENTED_EDGE ( 'NONE', *, *, #5449, .T. ) ;
#11770=FACE_OUTER_BOUND ( 'NONE', #15533, .T. ) ;
#11771=EDGE_CURVE ( 'NONE', #755, #13426, #8023, .T. ) ;
#11772=AXIS2_PLACEMENT_3D ( 'NONE', #8378, #5549, #15862 ) ;
#11773=CIRCLE ( 'NONE', #3597, 1.500000000000000888 ) ;
#11774=CARTESIAN_POINT ( 'NONE',  ( -11.93357161039406300, -79.84813783849037350, 21.65063509461100821 ) ) ;
#11775=DIRECTION ( 'NONE',  ( -0.1566598588826321192, 0.9876526153536342445, 7.798540720466730171E-17 ) ) ;
#11776=EDGE_LOOP ( 'NONE', ( #5882, #5273, #3994, #11148 ) ) ;
#11778=DIRECTION ( 'NONE',  ( -0.1566598588826321192, 0.9876526153536342445, 7.798540720466730171E-17 ) ) ;
#11780=CARTESIAN_POINT ( 'NONE',  ( 7.819480696678551723, -76.71494066083772623, 21.65063509461100821 ) ) ;
#11781=CARTESIAN_POINT ( 'NONE',  ( -19.34096622554629263, -81.02308678011010556, 17.32050807568881368 ) ) ;
#11785=FACE_OUTER_BOUND ( 'NONE', #9004, .T. ) ;
#11786=EDGE_CURVE ( 'NONE', #18596, #8019, #14855, .T. ) ;
#11788=ORIENTED_EDGE ( 'NONE', *, *, #1330, .T. ) ;
#11790=ORIENTED_EDGE ( 'NONE', *, *, #4064, .T. ) ;
#11791=EDGE_CURVE ( 'NONE', #4290, #7926, #15103, .T. ) ;
#11792=EDGE_CURVE ( 'NONE', #13882, #15648, #16636, .T. ) ;
#11793=EDGE_CURVE ( 'NONE', #15439, #16580, #9667, .T. ) ;
#11794=CIRCLE ( 'NONE', #5785, 1.500000000000001332 ) ;
#11795=CARTESIAN_POINT ( 'NONE',  ( -37.94164760650263446, -21.20551972688122788, 21.65063509461101887 ) ) ;
#11796=VECTOR ( 'NONE', #10172, 1000.000000000000000 ) ;
#11797=CARTESIAN_POINT ( 'NONE',  ( -8.476787456656362352, -79.29982833240116236, 21.65063509461100821 ) ) ;
#11798=DIRECTION ( 'NONE',  ( -0.1566598588826321192, 0.9876526153536342445, 7.798540720466731404E-17 ) ) ;
#11799=CARTESIAN_POINT ( 'NONE',  ( -49.01017969633301874, -28.02370111024092481, 21.65063509461101887 ) ) ;
#11801=AXIS2_PLACEMENT_3D ( 'NONE', #6024, #14924, #16360 ) ;
#11803=VERTEX_POINT ( 'NONE', #1879 ) ;
#11805=DIRECTION ( 'NONE',  ( -0.1566598588826321192, 0.9876526153536342445, 7.798540720466731404E-17 ) ) ;
#11806=CARTESIAN_POINT ( 'NONE',  ( -6.047290928450125946, -21.20899724884646531, -4.330127018922184767 ) ) ;
#11807=ORIENTED_EDGE ( 'NONE', *, *, #17686, .F. ) ;
#11808=DIRECTION ( 'NONE',  ( -0.1566598588826321192, 0.9876526153536342445, 7.798540720466731404E-17 ) ) ;
#11809=DIRECTION ( 'NONE',  ( -0.9876526153536341335, -0.1566598588826327021, 0.000000000000000000 ) ) ;
#11810=ORIENTED_EDGE ( 'NONE', *, *, #4297, .T. ) ;
#11812=ORIENTED_EDGE ( 'NONE', *, *, #3818, .F. ) ;
#11813=FACE_OUTER_BOUND ( 'NONE', #1348, .T. ) ;
#11814=VERTEX_POINT ( 'NONE', #9456 ) ;
#11815=VECTOR ( 'NONE', #14307, 1000.000000000000000 ) ;
#11816=ORIENTED_EDGE ( 'NONE', *, *, #519, .T. ) ;
#11817=AXIS2_PLACEMENT_3D ( 'NONE', #8534, #8621, #14309 ) ;
#11818=ORIENTED_EDGE ( 'NONE', *, *, #12705, .F. ) ;
#11819=CARTESIAN_POINT ( 'NONE',  ( -22.79775037928398618, -81.57139628619930249, -8.660254037844385522 ) ) ;
#11820=ORIENTED_EDGE ( 'NONE', *, *, #2271, .T. ) ;
#11821=DIRECTION ( 'NONE',  ( -0.1566598588826321192, 0.9876526153536342445, 7.798540720466730171E-17 ) ) ;
#11822=ORIENTED_EDGE ( 'NONE', *, *, #6025, .T. ) ;
#11823=DIRECTION ( 'NONE',  ( -0.1566598588826321747, 0.9876526153536343555, 0.000000000000000000 ) ) ;
#11824=DIRECTION ( 'NONE',  ( -0.9876526153536336894, -0.1566598588826349503, 0.000000000000000000 ) ) ;
#11825=ORIENTED_EDGE ( 'NONE', *, *, #434, .F. ) ;
#11826=EDGE_CURVE ( 'NONE', #5678, #12283, #1499, .T. ) ;
#11827=AXIS2_PLACEMENT_3D ( 'NONE', #8848, #15655, #41 ) ;
#11828=ADVANCED_FACE ( 'NONE', ( #18017 ), #15228, .F. ) ;
#11830=CARTESIAN_POINT ( 'NONE',  ( -31.68662391746666884, -82.98133501614299234, -21.65063509461098690 ) ) ;
#11831=VERTEX_POINT ( 'NONE', #3372 ) ;
#11832=FACE_BOUND ( 'NONE', #115, .T. ) ;
#11833=VECTOR ( 'NONE', #17097, 1000.000000000000000 ) ;
#11835=ORIENTED_EDGE ( 'NONE', *, *, #1956, .T. ) ;
#11837=CARTESIAN_POINT ( 'NONE',  ( 4.362696542940843081, -77.26325016692693737, -4.330127018922189208 ) ) ;
#11839=ORIENTED_EDGE ( 'NONE', *, *, #9023, .T. ) ;
#11840=ORIENTED_EDGE ( 'NONE', *, *, #12963, .F. ) ;
#11841=ORIENTED_EDGE ( 'NONE', *, *, #7332, .F. ) ;
#11842=EDGE_LOOP ( 'NONE', ( #234, #6773 ) ) ;
#11845=ORIENTED_EDGE ( 'NONE', *, *, #13427, .T. ) ;
#11846=FACE_BOUND ( 'NONE', #14227, .T. ) ;
#11849=EDGE_LOOP ( 'NONE', ( #8861, #7919 ) ) ;
#11850=FACE_OUTER_BOUND ( 'NONE', #17435, .T. ) ;
#11851=ORIENTED_EDGE ( 'NONE', *, *, #169, .F. ) ;
#11853=VECTOR ( 'NONE', #16433, 1000.000000000000000 ) ;
#11854=EDGE_CURVE ( 'NONE', #1643, #4960, #17870, .T. ) ;
#11855=ORIENTED_EDGE ( 'NONE', *, *, #17021, .F. ) ;
#11857=CARTESIAN_POINT ( 'NONE',  ( -44.07191661956487394, -27.24040181582776299, 4.330127018922217630 ) ) ;
#11858=LINE ( 'NONE', #6301, #1225 ) ;
#11859=CYLINDRICAL_SURFACE ( 'NONE', #9340, 1.500000000000001554 ) ;
#11860=CARTESIAN_POINT ( 'NONE',  ( -18.35331361019266794, -80.86642692122747178, -12.99038105676658539 ) ) ;
#11861=VERTEX_POINT ( 'NONE', #18510 ) ;
#11862=VERTEX_POINT ( 'NONE', #18317 ) ;
#11864=DIRECTION ( 'NONE',  ( -0.1566598588826321192, 0.9876526153536342445, 7.798540720466731404E-17 ) ) ;
#11865=CARTESIAN_POINT ( 'NONE',  ( -63.62061560569701157, -25.27867605782963523, -17.32050807568878170 ) ) ;
#11866=AXIS2_PLACEMENT_3D ( 'NONE', #17946, #10695, #7865 ) ;
#11868=DIRECTION ( 'NONE',  ( -0.9876526153536336894, -0.1566598588826350336, 0.000000000000000000 ) ) ;
#11869=CARTESIAN_POINT ( 'NONE',  ( -21.64537945316773460, -18.62063205531779531, -4.330127018922180326 ) ) ;
#11871=DIRECTION ( 'NONE',  ( 0.000000000000000000, 0.000000000000000000, 1.000000000000000000 ) ) ;
#11872=ORIENTED_EDGE ( 'NONE', *, *, #9131, .F. ) ;
#11874=CARTESIAN_POINT ( 'NONE',  ( -45.55339554259533230, -27.47539160415171722, -4.330127018922181215 ) ) ;
#11876=CARTESIAN_POINT ( 'NONE',  ( -61.15148406731292852, -24.88702641062306853, 12.99038105676661736 ) ) ;
#11877=EDGE_LOOP ( 'NONE', ( #12533, #12707, #3773, #17180 ) ) ;
#11879=DIRECTION ( 'NONE',  ( -0.9876526153536336894, -0.1566598588826349503, 0.000000000000000000 ) ) ;
#11880=ORIENTED_EDGE ( 'NONE', *, *, #9840, .T. ) ;
#11881=ADVANCED_FACE ( 'NONE', ( #8319 ), #18609, .F. ) ;
#11882=ORIENTED_EDGE ( 'NONE', *, *, #12943, .F. ) ;
#11883=VERTEX_POINT ( 'NONE', #5479 ) ;
#11885=LINE ( 'NONE', #15313, #8975 ) ;
#11887=DIRECTION ( 'NONE',  ( 0.000000000000000000, 0.000000000000000000, 1.000000000000000000 ) ) ;
#11888=LINE ( 'NONE', #4796, #9150 ) ;
#11889=CARTESIAN_POINT ( 'NONE',  ( -22.63303206852135929, -18.77729191420042554, -17.32050807568878170 ) ) ;
#11890=VERTEX_POINT ( 'NONE', #5573 ) ;
#11891=CARTESIAN_POINT ( 'NONE',  ( -57.89905323451571206, -29.43363984018462176, -8.660254037844380193 ) ) ;
#11892=EDGE_CURVE ( 'NONE', #13882, #2681, #4117, .T. ) ;
#11893=FACE_OUTER_BOUND ( 'NONE', #12393, .T. ) ;
#11894=VERTEX_POINT ( 'NONE', #9831 ) ;
#11896=CARTESIAN_POINT ( 'NONE',  ( -9.997901389864651378, -21.83563668437698269, 17.32050807568881012 ) ) ;
#11898=EDGE_CURVE ( 'NONE', #211, #14889, #2400, .T. ) ;
#11899=ORIENTED_EDGE ( 'NONE', *, *, #10161, .T. ) ;
#11900=DIRECTION ( 'NONE',  ( -0.9876526153536341335, -0.1566598588826327021, 0.000000000000000000 ) ) ;
#11901=ORIENTED_EDGE ( 'NONE', *, *, #2803, .F. ) ;
#11903=CARTESIAN_POINT ( 'NONE',  ( -14.93616446663280328, -22.61893597879013740, 17.32050807568881012 ) ) ;
#11904=FACE_OUTER_BOUND ( 'NONE', #2149, .T. ) ;
#11905=DIRECTION ( 'NONE',  ( -0.9876526153536341335, -0.1566598588826327021, 0.000000000000000000 ) ) ;
#11906=FACE_BOUND ( 'NONE', #15307, .T. ) ;
#11909=CARTESIAN_POINT ( 'NONE',  ( -84.16561914167408531, 33.59999999999999432, 25.00000000000001776 ) ) ;
#11910=AXIS2_PLACEMENT_3D ( 'NONE', #4647, #10424, #16218 ) ;
#11911=DIRECTION ( 'NONE',  ( -0.1566598588826321192, 0.9876526153536342445, 7.798540720466730171E-17 ) ) ;
#11915=EDGE_LOOP ( 'NONE', ( #3131, #6899, #2815, #14212 ) ) ;
#11916=DIRECTION ( 'NONE',  ( -0.1566598588826321192, 0.9876526153536342445, 7.798540720466730171E-17 ) ) ;
#11917=LINE ( 'NONE', #14698, #3286 ) ;
#11919=ORIENTED_EDGE ( 'NONE', *, *, #7495, .F. ) ;
#11920=EDGE_LOOP ( 'NONE', ( #16927, #13448 ) ) ;
#11921=CARTESIAN_POINT ( 'NONE',  ( -43.86756329862440396, -22.14547888017700927, 1.908195823574487804E-14 ) ) ;
#11922=ORIENTED_EDGE ( 'NONE', *, *, #13766, .F. ) ;
#11924=FACE_BOUND ( 'NONE', #4646, .T. ) ;
#11925=ORIENTED_EDGE ( 'NONE', *, *, #1471, .F. ) ;
#11926=ORIENTED_EDGE ( 'NONE', *, *, #6876, .F. ) ;
#11927=VERTEX_POINT ( 'NONE', #15422 ) ;
#11929=DIRECTION ( 'NONE',  ( 0.000000000000000000, 0.000000000000000000, 1.000000000000000000 ) ) ;
#11930=CIRCLE ( 'NONE', #4077, 1.499999999999999556 ) ;
#11931=CARTESIAN_POINT ( 'NONE',  ( -15.92381708198643153, -22.77559583767277473, 4.330127018922217630 ) ) ;
#11933=LINE ( 'NONE', #9032, #14998 ) ;
#11934=EDGE_LOOP ( 'NONE', ( #8818, #6187, #13892, #6805 ) ) ;
#11935=ORIENTED_EDGE ( 'NONE', *, *, #5461, .F. ) ;
#11936=CYLINDRICAL_SURFACE ( 'NONE', #5411, 1.500000000000001554 ) ;
#11938=ADVANCED_FACE ( 'NONE', ( #15597 ), #14185, .F. ) ;
#11939=CARTESIAN_POINT ( 'NONE',  ( -39.91695283720987675, -21.51883944464649190, 12.99038105676661736 ) ) ;
#11940=EDGE_LOOP ( 'NONE', ( #4118, #10489, #5098, #13728 ) ) ;
#11941=EDGE_LOOP ( 'NONE', ( #18058, #17284 ) ) ;
#11942=ADVANCED_FACE ( 'NONE', ( #13896 ), #944, .F. ) ;
#11943=AXIS2_PLACEMENT_3D ( 'NONE', #17196, #15755, #8176 ) ;
#11944=ORIENTED_EDGE ( 'NONE', *, *, #5223, .F. ) ;
#11946=DIRECTION ( 'NONE',  ( -0.1566598588826321192, 0.9876526153536342445, 7.798540720466730171E-17 ) ) ;
#11947=EDGE_CURVE ( 'NONE', #9479, #13518, #6654, .T. ) ;
#11948=CARTESIAN_POINT ( 'NONE',  ( -25.10216360690543524, -19.16894156140700645, -12.99038105676658006 ) ) ;
#11949=CARTESIAN_POINT ( 'NONE',  ( -28.22983976372896109, -82.43302551005379541, 4.330127018922213189 ) ) ;
#11950=DIRECTION ( 'NONE',  ( 0.000000000000000000, 0.000000000000000000, 1.000000000000000000 ) ) ;
#11953=AXIS2_PLACEMENT_3D ( 'NONE', #8846, #206, #17583 ) ;
#11954=CARTESIAN_POINT ( 'NONE',  ( -68.72359699322777260, -88.85607972424168111, -8.660254037844385522 ) ) ;
#11955=DIRECTION ( 'NONE',  ( 1.000000000000000000, 0.000000000000000000, 0.000000000000000000 ) ) ;
#11957=CARTESIAN_POINT ( 'NONE',  ( -47.03487446562577645, -27.71038139247565368, 12.99038105676661736 ) ) ;
#11958=ORIENTED_EDGE ( 'NONE', *, *, #3645, .T. ) ;
#11960=CARTESIAN_POINT ( 'NONE',  ( -0.1213752363283457369, -20.26903809555066616, 1.348786077179112100E-14 ) ) ;
#11961=AXIS2_PLACEMENT_3D ( 'NONE', #14292, #2818, #1404 ) ;
#11963=DIRECTION ( 'NONE',  ( -0.1566598588826321192, 0.9876526153536342445, 7.798540720466731404E-17 ) ) ;
#11964=ORIENTED_EDGE ( 'NONE', *, *, #14218, .T. ) ;
#11965=CIRCLE ( 'NONE', #3804, 1.500000000000000444 ) ;
#11966=EDGE_CURVE ( 'NONE', #1641, #10341, #10258, .T. ) ;
#11967=CARTESIAN_POINT ( 'NONE',  ( -26.58364252993588650, -19.40393134973095357, -12.99038105676658006 ) ) ;
#11968=VERTEX_POINT ( 'NONE', #13998 ) ;
#11969=CARTESIAN_POINT ( 'NONE',  ( -62.83731631128386397, -30.21693913459777647, -17.32050807568878170 ) ) ;
#11970=ORIENTED_EDGE ( 'NONE', *, *, #14923, .T. ) ;
#11971=CARTESIAN_POINT ( 'NONE',  ( -35.14340807120436239, -83.52964452223220349, -4.330127018922185655 ) ) ;
#11973=ADVANCED_FACE ( 'NONE', ( #12555 ), #18410, .F. ) ;
#11974=AXIS2_PLACEMENT_3D ( 'NONE', #3469, #10864, #12488 ) ;
#11977=DIRECTION ( 'NONE',  ( 0.000000000000000000, 0.000000000000000000, 1.000000000000000000 ) ) ;
#11978=FACE_BOUND ( 'NONE', #2523, .T. ) ;
#11979=CIRCLE ( 'NONE', #9595, 1.500000000000000888 ) ;
#11982=CARTESIAN_POINT ( 'NONE',  ( -0.5755665338273054932, -78.04654946134009208, 12.99038105676660848 ) ) ;
#11984=CARTESIAN_POINT ( 'NONE',  ( -46.50141314777111745, -85.33123289938248490, -4.330127018922185655 ) ) ;
#11986=ORIENTED_EDGE ( 'NONE', *, *, #14705, .F. ) ;
#11987=DIRECTION ( 'NONE',  ( -0.1566598588826321192, 0.9876526153536342445, 7.798540720466731404E-17 ) ) ;
#11988=CIRCLE ( 'NONE', #12918, 1.500000000000001332 ) ;
#11991=CIRCLE ( 'NONE', #8701, 1.500000000000000000 ) ;
#11992=ORIENTED_EDGE ( 'NONE', *, *, #6505, .F. ) ;
#11993=CARTESIAN_POINT ( 'NONE',  ( -48.97054468615519340, -85.72288254658904805, -17.32050807568878525 ) ) ;
#11994=ADVANCED_FACE ( 'NONE', ( #3937 ), #11136, .F. ) ;
#11995=DIRECTION ( 'NONE',  ( -0.9876526153536336894, -0.1566598588826349503, 0.000000000000000000 ) ) ;
#11996=CIRCLE ( 'NONE', #11694, 1.500000000000000888 ) ;
#11997=EDGE_CURVE ( 'NONE', #2873, #15378, #7013, .T. ) ;
#11999=CARTESIAN_POINT ( 'NONE',  ( -9.299721761247353058, -16.66238381928489787, 1.561251128379126385E-14 ) ) ;
#12003=CARTESIAN_POINT ( 'NONE',  ( -11.76885329963143434, -17.05403346649147878, -12.99038105676658006 ) ) ;
#12004=DIRECTION ( 'NONE',  ( -0.1566598588826321192, 0.9876526153536342445, 7.798540720466731404E-17 ) ) ;
#12005=CARTESIAN_POINT ( 'NONE',  ( 10.28861223506262412, -76.32329101363113466, -17.32050807568878525 ) ) ;
#12006=ORIENTED_EDGE ( 'NONE', *, *, #1735, .T. ) ;
#12007=AXIS2_PLACEMENT_3D ( 'NONE', #7693, #13360, #13442 ) ;
#12008=CARTESIAN_POINT ( 'NONE',  ( 4.362696542940843081, -77.26325016692693737, 21.65063509461100821 ) ) ;
#12010=CARTESIAN_POINT ( 'NONE',  ( -12.92122422574768592, -80.00479769737299307, -8.660254037844385522 ) ) ;
#12011=DIRECTION ( 'NONE',  ( -0.9876526153536336894, -0.1566598588826349503, 0.000000000000000000 ) ) ;
#12012=AXIS2_PLACEMENT_3D ( 'NONE', #13343, #14673, #11709 ) ;
#12013=LINE ( 'NONE', #13264, #18790 ) ;
#12014=ORIENTED_EDGE ( 'NONE', *, *, #11076, .T. ) ;
#12016=ORIENTED_EDGE ( 'NONE', *, *, #15105, .F. ) ;
#12020=FACE_BOUND ( 'NONE', #11567, .T. ) ;
#12021=ADVANCED_FACE ( 'NONE', ( #18777 ), #7187, .F. ) ;
#12023=ADVANCED_FACE ( 'NONE', ( #5771 ), #17624, .F. ) ;
#12024=ADVANCED_FACE ( 'NONE', ( #1495 ), #14465, .F. ) ;
#12025=DIRECTION ( 'NONE',  ( -0.9876526153536336894, -0.1566598588826349503, 0.000000000000000000 ) ) ;
#12026=ORIENTED_EDGE ( 'NONE', *, *, #14153, .F. ) ;
#12028=AXIS2_PLACEMENT_3D ( 'NONE', #9037, #6012, #17605 ) ;
#12030=LINE ( 'NONE', #14633, #9145 ) ;
#12031=CARTESIAN_POINT ( 'NONE',  ( -28.22983976372897530, -82.43302551005378120, -21.65063509461098690 ) ) ;
#12032=AXIS2_PLACEMENT_3D ( 'NONE', #4485, #8753, #17599 ) ;
#12033=DIRECTION ( 'NONE',  ( -0.000000000000000000, -0.000000000000000000, -1.000000000000000000 ) ) ;
#12035=CARTESIAN_POINT ( 'NONE',  ( -57.89905323451569785, -29.43363984018461466, 8.660254037844417496 ) ) ;
#12037=DIRECTION ( 'NONE',  ( -0.9876526153536341335, -0.1566598588826327021, 0.000000000000000000 ) ) ;
#12039=ORIENTED_EDGE ( 'NONE', *, *, #15829, .T. ) ;
#12041=CARTESIAN_POINT ( 'NONE',  ( -19.17624791478365864, -18.22898240811121795, 1.908195823574487804E-14 ) ) ;
#12042=EDGE_CURVE ( 'NONE', #5315, #12777, #1756, .T. ) ;
#12044=AXIS2_PLACEMENT_3D ( 'NONE', #4376, #2580, #17200 ) ;
#12045=ORIENTED_EDGE ( 'NONE', *, *, #1694, .T. ) ;
#12046=CARTESIAN_POINT ( 'NONE',  ( -65.26681283949008616, -88.30777021815246997, 1.424741226644455312E-14 ) ) ;
#12048=CIRCLE ( 'NONE', #8462, 1.499999999999999556 ) ;
#12049=DIRECTION ( 'NONE',  ( -0.1566598588826321192, 0.9876526153536342445, 7.798540720466730171E-17 ) ) ;
#12051=DIRECTION ( 'NONE',  ( -0.1566598588826321192, 0.9876526153536342445, 7.798540720466730171E-17 ) ) ;
#12052=EDGE_CURVE ( 'NONE', #14468, #299, #2987, .T. ) ;
#12053=VERTEX_POINT ( 'NONE', #11508 ) ;
#12054=CIRCLE ( 'NONE', #6972, 1.499999999999999556 ) ;
#12055=EDGE_CURVE ( 'NONE', #6017, #8901, #13577, .T. ) ;
#12056=CARTESIAN_POINT ( 'NONE',  ( -65.30644784966793281, -30.60858878180435738, 12.99038105676661736 ) ) ;
#12058=DIRECTION ( 'NONE',  ( -0.9876526153536336894, -0.1566598588826349503, 0.000000000000000000 ) ) ;
#12060=AXIS2_PLACEMENT_3D ( 'NONE', #10463, #10827, #635 ) ;
#12061=EDGE_LOOP ( 'NONE', ( #11925, #4858 ) ) ;
#12062=LINE ( 'NONE', #6229, #11208 ) ;
#12063=AXIS2_PLACEMENT_3D ( 'NONE', #163, #17528, #7461 ) ;
#12065=LINE ( 'NONE', #17044, #7285 ) ;
#12066=EDGE_LOOP ( 'NONE', ( #16876, #15300, #2479, #15704 ) ) ;
#12067=VERTEX_POINT ( 'NONE', #13125 ) ;
#12068=EDGE_LOOP ( 'NONE', ( #8690, #16468, #15194, #2584 ) ) ;
#12070=CIRCLE ( 'NONE', #916, 1.500000000000001332 ) ;
#12071=AXIS2_PLACEMENT_3D ( 'NONE', #10539, #10356, #16152 ) ;
#12072=LINE ( 'NONE', #5949, #7197 ) ;
#12073=VERTEX_POINT ( 'NONE', #157 ) ;
#12074=DIRECTION ( 'NONE',  ( -0.1566598588826321192, 0.9876526153536342445, 7.798540720466731404E-17 ) ) ;
#12076=AXIS2_PLACEMENT_3D ( 'NONE', #2525, #2612, #17238 ) ;
#12077=EDGE_LOOP ( 'NONE', ( #15372, #5341, #13957, #11992 ) ) ;
#12081=DIRECTION ( 'NONE',  ( -0.9876526153536341335, -0.1566598588826327021, 0.000000000000000000 ) ) ;
#12082=CARTESIAN_POINT ( 'NONE',  ( -61.31620237807555895, -87.68113078262194904, -4.330127018922185655 ) ) ;
#12083=DIRECTION ( 'NONE',  ( 0.000000000000000000, 0.000000000000000000, 1.000000000000000000 ) ) ;
#12084=ORIENTED_EDGE ( 'NONE', *, *, #2633, .T. ) ;
#12086=EDGE_CURVE ( 'NONE', #11320, #8678, #8607, .T. ) ;
#12087=AXIS2_PLACEMENT_3D ( 'NONE', #13902, #9652, #12485 ) ;
#12088=DIRECTION ( 'NONE',  ( -0.9876526153536336894, -0.1566598588826349503, 0.000000000000000000 ) ) ;
#12089=DIRECTION ( 'NONE',  ( -0.1566598588826321192, 0.9876526153536342445, 7.798540720466730171E-17 ) ) ;
#12090=VERTEX_POINT ( 'NONE', #1670 ) ;
#12094=AXIS2_PLACEMENT_3D ( 'NONE', #2878, #14172, #15679 ) ;
#12095=EDGE_LOOP ( 'NONE', ( #4263, #35 ) ) ;
#12096=ADVANCED_FACE ( 'NONE', ( #7284 ), #13035, .F. ) ;
#12097=VERTEX_POINT ( 'NONE', #17342 ) ;
#12098=EDGE_LOOP ( 'NONE', ( #64, #18719 ) ) ;
#12099=CARTESIAN_POINT ( 'NONE',  ( -31.72625892764450839, -25.28215357979487266, 8.660254037844417496 ) ) ;
#12100=ORIENTED_EDGE ( 'NONE', *, *, #18751, .T. ) ;
#12101=AXIS2_PLACEMENT_3D ( 'NONE', #14462, #1490, #7276 ) ;
#12103=VECTOR ( 'NONE', #11119, 1000.000000000000000 ) ;
#12104=DIRECTION ( 'NONE',  ( -0.9876526153536336894, -0.1566598588826350336, 0.000000000000000000 ) ) ;
#12106=DIRECTION ( 'NONE',  ( -0.000000000000000000, -0.000000000000000000, -1.000000000000000000 ) ) ;
#12107=CARTESIAN_POINT ( 'NONE',  ( -46.50141314777111745, -85.33123289938247069, -12.99038105676658539 ) ) ;
#12108=DIRECTION ( 'NONE',  ( -0.9876526153536336894, -0.1566598588826349503, 0.000000000000000000 ) ) ;
#12109=VERTEX_POINT ( 'NONE', #4503 ) ;
#12110=VECTOR ( 'NONE', #6806, 1000.000000000000000 ) ;
#12111=DIRECTION ( 'NONE',  ( 0.000000000000000000, 0.000000000000000000, 1.000000000000000000 ) ) ;
#12113=ADVANCED_FACE ( 'NONE', ( #18692 ), #6030, .F. ) ;
#12115=AXIS2_PLACEMENT_3D ( 'NONE', #5870, #8425, #17357 ) ;
#12116=ORIENTED_EDGE ( 'NONE', *, *, #1524, .F. ) ;
#12117=FACE_OUTER_BOUND ( 'NONE', #16520, .T. ) ;
#12118=ORIENTED_EDGE ( 'NONE', *, *, #11997, .F. ) ;
#12119=EDGE_CURVE ( 'NONE', #4650, #15970, #279, .T. ) ;
#12121=EDGE_LOOP ( 'NONE', ( #17092, #404 ) ) ;
#12122=CYLINDRICAL_SURFACE ( 'NONE', #4716, 1.500000000000001554 ) ;
#12123=AXIS2_PLACEMENT_3D ( 'NONE', #8656, #14344, #12898 ) ;
#12124=FACE_BOUND ( 'NONE', #857, .T. ) ;
#12125=EDGE_LOOP ( 'NONE', ( #5706, #6104 ) ) ;
#12126=AXIS2_PLACEMENT_3D ( 'NONE', #3754, #7955, #5097 ) ;
#12127=AXIS2_PLACEMENT_3D ( 'NONE', #13655, #699, #14995 ) ;
#12128=EDGE_CURVE ( 'NONE', #777, #14841, #18181, .T. ) ;
#12129=FACE_BOUND ( 'NONE', #3126, .T. ) ;
#12130=EDGE_LOOP ( 'NONE', ( #6383, #3834, #15939, #12147, #6143, #6412, #5554 ) ) ;
#12132=ORIENTED_EDGE ( 'NONE', *, *, #9371, .T. ) ;
#12135=AXIS2_PLACEMENT_3D ( 'NONE', #9273, #7683, #283 ) ;
#12137=CYLINDRICAL_SURFACE ( 'NONE', #8028, 1.500000000000001554 ) ;
#12138=EDGE_CURVE ( 'NONE', #16672, #12097, #5752, .T. ) ;
#12139=VERTEX_POINT ( 'NONE', #17425 ) ;
#12141=CARTESIAN_POINT ( 'NONE',  ( -47.98289207080156871, -85.56622268770641426, -12.99038105676658539 ) ) ;
#12142=EDGE_CURVE ( 'NONE', #14841, #3425, #17518, .T. ) ;
#12143=ORIENTED_EDGE ( 'NONE', *, *, #8250, .F. ) ;
#12144=EDGE_CURVE ( 'NONE', #15928, #11588, #4225, .T. ) ;
#12145=DIRECTION ( 'NONE',  ( 2.887450008416415878E-16, 0.000000000000000000, 1.000000000000000000 ) ) ;
#12147=ORIENTED_EDGE ( 'NONE', *, *, #17812, .F. ) ;
#12149=EDGE_CURVE ( 'NONE', #3917, #2189, #7860, .T. ) ;
#12150=EDGE_LOOP ( 'NONE', ( #17393, #14012, #9362, #17203 ) ) ;
#12151=ORIENTED_EDGE ( 'NONE', *, *, #3556, .F. ) ;
#12153=ORIENTED_EDGE ( 'NONE', *, *, #5351, .F. ) ;
#12154=CIRCLE ( 'NONE', #3982, 1.500000000000001332 ) ;
#12155=CARTESIAN_POINT ( 'NONE',  ( -53.90880776292333820, -86.50618184100221697, -8.660254037844385522 ) ) ;
#12156=CYLINDRICAL_SURFACE ( 'NONE', #4212, 1.500000000000001554 ) ;
#12158=DIRECTION ( 'NONE',  ( -0.1566598588826321747, 0.9876526153536343555, 0.000000000000000000 ) ) ;
#12160=DIRECTION ( 'NONE',  ( -0.9876526153536336894, -0.1566598588826349503, 0.000000000000000000 ) ) ;
#12161=EDGE_CURVE ( 'NONE', #795, #7723, #14825, .T. ) ;
#12162=VERTEX_POINT ( 'NONE', #5051 ) ;
#12163=EDGE_LOOP ( 'NONE', ( #573, #13493 ) ) ;
#12164=DIRECTION ( 'NONE',  ( -0.9876526153536336894, -0.1566598588826349503, 0.000000000000000000 ) ) ;
#12165=ORIENTED_EDGE ( 'NONE', *, *, #8786, .T. ) ;
#12166=VERTEX_POINT ( 'NONE', #9235 ) ;
#12167=EDGE_CURVE ( 'NONE', #3425, #11543, #13910, .T. ) ;
#12168=DIRECTION ( 'NONE',  ( -0.1566598588826321192, 0.9876526153536342445, 7.798540720466730171E-17 ) ) ;
#12170=VERTEX_POINT ( 'NONE', #17996 ) ;
#12171=EDGE_CURVE ( 'NONE', #2476, #10913, #17894, .T. ) ;
#12174=LINE ( 'NONE', #13605, #14830 ) ;
#12175=VECTOR ( 'NONE', #14103, 1000.000000000000000 ) ;
#12177=VERTEX_POINT ( 'NONE', #7824 ) ;
#12178=CARTESIAN_POINT ( 'NONE',  ( -71.02801022084922522, -26.45362499944937795, -4.330127018922180326 ) ) ;
#12179=DIRECTION ( 'NONE',  ( -0.1566598588826321747, 0.9876526153536343555, 0.000000000000000000 ) ) ;
#12180=ORIENTED_EDGE ( 'NONE', *, *, #16472, .F. ) ;
#12181=CARTESIAN_POINT ( 'NONE',  ( -35.67686938905902849, -25.90879301532540779, 21.65063509461101887 ) ) ;
#12183=DIRECTION ( 'NONE',  ( 0.000000000000000000, 0.000000000000000000, 1.000000000000000000 ) ) ;
#12184=CARTESIAN_POINT ( 'NONE',  ( -34.19539046602857724, -25.67380322700145356, 4.330127018922217630 ) ) ;
#12185=CYLINDRICAL_SURFACE ( 'NONE', #10879, 1.500000000000001554 ) ;
#12186=DIRECTION ( 'NONE',  ( -0.9876526153536341335, -0.1566598588826327021, 0.000000000000000000 ) ) ;
#12188=ORIENTED_EDGE ( 'NONE', *, *, #17096, .F. ) ;
#12189=CARTESIAN_POINT ( 'NONE',  ( -56.37793930130739994, -86.89783148820880854, 21.65063509461101532 ) ) ;
#12190=AXIS2_PLACEMENT_3D ( 'NONE', #15613, #17160, #15825 ) ;
#12191=ORIENTED_EDGE ( 'NONE', *, *, #17071, .T. ) ;
#12192=ADVANCED_FACE ( 'NONE', ( #13679 ), #724, .F. ) ;
#12193=ORIENTED_EDGE ( 'NONE', *, *, #14335, .F. ) ;
#12194=DIRECTION ( 'NONE',  ( 0.000000000000000000, 0.000000000000000000, 1.000000000000000000 ) ) ;
#12196=LINE ( 'NONE', #3476, #17984 ) ;
#12197=ORIENTED_EDGE ( 'NONE', *, *, #15529, .T. ) ;
#12200=CYLINDRICAL_SURFACE ( 'NONE', #11056, 1.500000000000001554 ) ;
#12201=DIRECTION ( 'NONE',  ( -0.9876526153536336894, -0.1566598588826349503, 0.000000000000000000 ) ) ;
#12204=ORIENTED_EDGE ( 'NONE', *, *, #9229, .F. ) ;
#12205=CARTESIAN_POINT ( 'NONE',  ( -62.63296299034339398, -25.12201619894700855, -4.330127018922180326 ) ) ;
#12207=ORIENTED_EDGE ( 'NONE', *, *, #17118, .F. ) ;
#12208=VERTEX_POINT ( 'NONE', #13313 ) ;
#12209=ORIENTED_EDGE ( 'NONE', *, *, #5945, .F. ) ;
#12210=ORIENTED_EDGE ( 'NONE', *, *, #13759, .F. ) ;
#12211=ORIENTED_EDGE ( 'NONE', *, *, #7255, .T. ) ;
#12212=DIRECTION ( 'NONE',  ( -1.000000000000000000, 0.000000000000000000, 0.000000000000000000 ) ) ;
#12214=FACE_BOUND ( 'NONE', #17819, .T. ) ;
#12215=ORIENTED_EDGE ( 'NONE', *, *, #8841, .T. ) ;
#12216=EDGE_CURVE ( 'NONE', #14341, #1903, #6363, .T. ) ;
#12217=CARTESIAN_POINT ( 'NONE',  ( -84.16561914167408531, 33.59999999999999432, -30.00000000000000000 ) ) ;
#12218=AXIS2_PLACEMENT_3D ( 'NONE', #5577, #5111, #10886 ) ;
#12220=DIRECTION ( 'NONE',  ( -0.1566598588826321192, 0.9876526153536342445, 7.798540720466731404E-17 ) ) ;
#12221=EDGE_CURVE ( 'NONE', #7418, #12715, #9369, .T. ) ;
#12222=FACE_BOUND ( 'NONE', #7587, .T. ) ;
#12223=DIRECTION ( 'NONE',  ( -0.1566598588826321192, 0.9876526153536342445, 7.798540720466730171E-17 ) ) ;
#12224=ORIENTED_EDGE ( 'NONE', *, *, #5448, .T. ) ;
#12225=CARTESIAN_POINT ( 'NONE',  ( -4.361458684479201153, -15.87908452487173427, 8.660254037844412167 ) ) ;
#12226=DIRECTION ( 'NONE',  ( -0.1566598588826321192, 0.9876526153536342445, 7.798540720466730171E-17 ) ) ;
#12227=LINE ( 'NONE', #10805, #10743 ) ;
#12229=ORIENTED_EDGE ( 'NONE', *, *, #13917, .T. ) ;
#12230=DIRECTION ( 'NONE',  ( -0.9876526153536336894, -0.1566598588826349503, 0.000000000000000000 ) ) ;
#12231=FACE_OUTER_BOUND ( 'NONE', #17858, .T. ) ;
#12232=EDGE_LOOP ( 'NONE', ( #7599, #3172 ) ) ;
#12233=FACE_OUTER_BOUND ( 'NONE', #988, .T. ) ;
#12235=CYLINDRICAL_SURFACE ( 'NONE', #16398, 1.500000000000000888 ) ;
#12238=FACE_BOUND ( 'NONE', #18146, .T. ) ;
#12239=EDGE_CURVE ( 'NONE', #9341, #5533, #4828, .T. ) ;
#12240=CARTESIAN_POINT ( 'NONE',  ( -67.77557938805200877, -31.00023842901093118, -8.660254037844380193 ) ) ;
#12241=ADVANCED_FACE ( 'NONE', ( #14837 ), #6223, .F. ) ;
#12242=CIRCLE ( 'NONE', #477, 1.499999999999999556 ) ;
#12243=DIRECTION ( 'NONE',  ( 0.000000000000000000, 0.000000000000000000, 1.000000000000000000 ) ) ;
#12246=EDGE_CURVE ( 'NONE', #14796, #62, #9, .T. ) ;
#12247=CARTESIAN_POINT ( 'NONE',  ( -34.15575545585074480, -83.37298466334958391, -17.32050807568878525 ) ) ;
#12248=LINE ( 'NONE', #18083, #15032 ) ;
#12249=CARTESIAN_POINT ( 'NONE',  ( -14.40270314877813895, -80.23978748569695085, 1.424741226644455312E-14 ) ) ;
#12250=LINE ( 'NONE', #5056, #464 ) ;
#12251=DIRECTION ( 'NONE',  ( -0.9876526153536341335, -0.1566598588826327021, 0.000000000000000000 ) ) ;
#12253=VERTEX_POINT ( 'NONE', #10662 ) ;
#12254=DIRECTION ( 'NONE',  ( -0.1566598588826321747, 0.9876526153536343555, 0.000000000000000000 ) ) ;
#12255=AXIS2_PLACEMENT_3D ( 'NONE', #15796, #9299, #15078 ) ;
#12256=VERTEX_POINT ( 'NONE', #15113 ) ;
#12257=ORIENTED_EDGE ( 'NONE', *, *, #7737, .F. ) ;
#12258=DIRECTION ( 'NONE',  ( -0.1566598588826321192, 0.9876526153536342445, 7.798540720466730171E-17 ) ) ;
#12259=AXIS2_PLACEMENT_3D ( 'NONE', #2417, #8205, #13977 ) ;
#12260=ORIENTED_EDGE ( 'NONE', *, *, #5217, .F. ) ;
#12261=DIRECTION ( 'NONE',  ( -0.9876526153536341335, -0.1566598588826327021, 0.000000000000000000 ) ) ;
#12262=FACE_OUTER_BOUND ( 'NONE', #7110, .T. ) ;
#12263=DIRECTION ( 'NONE',  ( -0.1566598588826321192, 0.9876526153536342445, 7.798540720466731404E-17 ) ) ;
#12264=EDGE_CURVE ( 'NONE', #5148, #8214, #16964, .T. ) ;
#12265=ADVANCED_FACE ( 'NONE', ( #16540 ), #9330, .F. ) ;
#12266=CARTESIAN_POINT ( 'NONE',  ( -24.11451099155181055, -19.01228170252437266, -8.660254037844380193 ) ) ;
#12267=AXIS2_PLACEMENT_3D ( 'NONE', #14239, #14037, #7062 ) ;
#12269=CARTESIAN_POINT ( 'NONE',  ( -49.79347899074616635, -23.08543803347281198, 21.65063509461101887 ) ) ;
#12270=DIRECTION ( 'NONE',  ( 0.000000000000000000, 0.000000000000000000, 1.000000000000000000 ) ) ;
#12271=AXIS2_PLACEMENT_3D ( 'NONE', #6838, #18441, #5406 ) ;
#12272=LINE ( 'NONE', #12483, #6262 ) ;
#12273=FACE_BOUND ( 'NONE', #385, .T. ) ;
#12274=CARTESIAN_POINT ( 'NONE',  ( -19.17624791478365864, -18.22898240811121795, 17.32050807568881368 ) ) ;
#12275=FACE_OUTER_BOUND ( 'NONE', #2275, .T. ) ;
#12276=DIRECTION ( 'NONE',  ( -0.1566598588826321192, 0.9876526153536342445, 7.798540720466730171E-17 ) ) ;
#12277=ORIENTED_EDGE ( 'NONE', *, *, #14813, .F. ) ;
#12278=ORIENTED_EDGE ( 'NONE', *, *, #8506, .T. ) ;
#12279=CARTESIAN_POINT ( 'NONE',  ( -20.16390053013728334, -18.38564226699385529, 12.99038105676661736 ) ) ;
#12281=CARTESIAN_POINT ( 'NONE',  ( -83.14047854185180597, 6.938893903907228378E-15, -24.99999999999999289 ) ) ;
#12282=ORIENTED_EDGE ( 'NONE', *, *, #980, .T. ) ;
#12283=VERTEX_POINT ( 'NONE', #815 ) ;
#12284=DIRECTION ( 'NONE',  ( -0.1566598588826321747, 0.9876526153536343555, 0.000000000000000000 ) ) ;
#12286=ORIENTED_EDGE ( 'NONE', *, *, #17050, .T. ) ;
#12287=CARTESIAN_POINT ( 'NONE',  ( -37.44782129882581501, -21.12718979743990033, -17.32050807568878170 ) ) ;
#12288=FACE_OUTER_BOUND ( 'NONE', #15743, .T. ) ;
#12290=CARTESIAN_POINT ( 'NONE',  ( -24.11451099155181055, -19.01228170252437977, 17.32050807568882078 ) ) ;
#12292=CARTESIAN_POINT ( 'NONE',  ( -22.34355908178503469, -23.79388492040988012, 21.65063509461101177 ) ) ;
#12293=DIRECTION ( 'NONE',  ( -0.1566598588826321192, 0.9876526153536342445, 7.798540720466731404E-17 ) ) ;
#12294=CARTESIAN_POINT ( 'NONE',  ( -46.33669483700848701, -22.53712852738358308, -12.99038105676658006 ) ) ;
#12295=EDGE_LOOP ( 'NONE', ( #13935, #4942 ) ) ;
#12296=EDGE_CURVE ( 'NONE', #14180, #18619, #10579, .T. ) ;
#12298=CARTESIAN_POINT ( 'NONE',  ( -30.73860631229088369, -25.12549372091224598, -4.330127018922181215 ) ) ;
#12300=VECTOR ( 'NONE', #10010, 1000.000000000000000 ) ;
#12301=AXIS2_PLACEMENT_3D ( 'NONE', #12189, #5294, #3750 ) ;
#12302=CARTESIAN_POINT ( 'NONE',  ( -64.31879523431430812, -30.45192892292171294, 17.32050807568881723 ) ) ;
#12304=ORIENTED_EDGE ( 'NONE', *, *, #13940, .F. ) ;
#12305=EDGE_LOOP ( 'NONE', ( #18544, #10042, #1895, #17106 ) ) ;
#12306=EDGE_LOOP ( 'NONE', ( #14882, #2573, #6491, #15887 ) ) ;
#12307=ORIENTED_EDGE ( 'NONE', *, *, #16350, .T. ) ;
#12308=DIRECTION ( 'NONE',  ( -0.000000000000000000, -0.000000000000000000, -1.000000000000000000 ) ) ;
#12309=AXIS2_PLACEMENT_3D ( 'NONE', #9995, #2807, #14365 ) ;
#12310=FACE_BOUND ( 'NONE', #3732, .T. ) ;
#12314=DIRECTION ( 'NONE',  ( -0.1566598588826321192, 0.9876526153536342445, 7.798540720466730171E-17 ) ) ;
#12315=ORIENTED_EDGE ( 'NONE', *, *, #10376, .F. ) ;
#12316=DIRECTION ( 'NONE',  ( -0.1566598588826321192, 0.9876526153536342445, 7.798540720466730171E-17 ) ) ;
#12318=DIRECTION ( 'NONE',  ( -0.1566598588826321192, 0.9876526153536342445, 7.798540720466730171E-17 ) ) ;
#12319=LINE ( 'NONE', #1001, #10245 ) ;
#12320=DIRECTION ( 'NONE',  ( -0.9876526153536336894, -0.1566598588826349503, 0.000000000000000000 ) ) ;
#12321=CIRCLE ( 'NONE', #8461, 1.500000000000000888 ) ;
#12322=EDGE_LOOP ( 'NONE', ( #7653, #8411 ) ) ;
#12323=ORIENTED_EDGE ( 'NONE', *, *, #5216, .F. ) ;
#12324=DIRECTION ( 'NONE',  ( -0.9876526153536336894, -0.1566598588826349503, 0.000000000000000000 ) ) ;
#12326=AXIS2_PLACEMENT_3D ( 'NONE', #9476, #5104, #3675 ) ;
#12328=ORIENTED_EDGE ( 'NONE', *, *, #14034, .T. ) ;
#12329=VERTEX_POINT ( 'NONE', #1105 ) ;
#12330=DIRECTION ( 'NONE',  ( -0.1566598588826321192, 0.9876526153536342445, 7.798540720466730171E-17 ) ) ;
#12332=EDGE_CURVE ( 'NONE', #15912, #13410, #17119, .T. ) ;
#12333=ORIENTED_EDGE ( 'NONE', *, *, #8539, .T. ) ;
#12334=VECTOR ( 'NONE', #1739, 1000.000000000000000 ) ;
#12335=FACE_OUTER_BOUND ( 'NONE', #1174, .T. ) ;
#12336=AXIS2_PLACEMENT_3D ( 'NONE', #18665, #5636, #11391 ) ;
#12337=AXIS2_PLACEMENT_3D ( 'NONE', #12035, #17882, #7714 ) ;
#12340=CIRCLE ( 'NONE', #10824, 1.500000000000000444 ) ;
#12342=FACE_OUTER_BOUND ( 'NONE', #13115, .T. ) ;
#12344=DIRECTION ( 'NONE',  ( -0.9876526153536341335, -0.1566598588826327021, 0.000000000000000000 ) ) ;
#12345=CIRCLE ( 'NONE', #6953, 2.500000000000002220 ) ;
#12347=ORIENTED_EDGE ( 'NONE', *, *, #16731, .F. ) ;
#12348=ORIENTED_EDGE ( 'NONE', *, *, #10659, .T. ) ;
#12349=CARTESIAN_POINT ( 'NONE',  ( 11.77009115809307715, -76.08830122530719109, -17.32050807568878525 ) ) ;
#12350=EDGE_CURVE ( 'NONE', #5485, #384, #13767, .T. ) ;
#12351=AXIS2_PLACEMENT_3D ( 'NONE', #7605, #16038, #11734 ) ;
#12352=ORIENTED_EDGE ( 'NONE', *, *, #12610, .F. ) ;
#12353=ORIENTED_EDGE ( 'NONE', *, *, #7078, .T. ) ;
#12355=CARTESIAN_POINT ( 'NONE',  ( -43.04462899403342391, -84.78292339329327376, -12.99038105676658539 ) ) ;
#12356=AXIS2_PLACEMENT_3D ( 'NONE', #8980, #13618, #378 ) ;
#12357=ORIENTED_EDGE ( 'NONE', *, *, #14608, .F. ) ;
#12358=EDGE_LOOP ( 'NONE', ( #8962, #2563 ) ) ;
#12359=DIRECTION ( 'NONE',  ( -0.9876526153536336894, -0.1566598588826349503, 0.000000000000000000 ) ) ;
#12360=DIRECTION ( 'NONE',  ( -0.9876526153536336894, -0.1566598588826349503, 0.000000000000000000 ) ) ;
#12361=EDGE_CURVE ( 'NONE', #17699, #8605, #18193, .T. ) ;
#12362=EDGE_CURVE ( 'NONE', #3308, #13600, #3599, .T. ) ;
#12363=CARTESIAN_POINT ( 'NONE',  ( -56.21322099054479082, -24.10372711620989961, -12.99038105676658006 ) ) ;
#12365=VECTOR ( 'NONE', #5350, 1000.000000000000000 ) ;
#12366=DIRECTION ( 'NONE',  ( -0.1566598588826321192, 0.9876526153536342445, 7.798540720466730171E-17 ) ) ;
#12368=CARTESIAN_POINT ( 'NONE',  ( -57.89905323451571206, -29.43363984018462176, 1.869203119972154228E-14 ) ) ;
#12370=ORIENTED_EDGE ( 'NONE', *, *, #2362, .F. ) ;
#12371=DIRECTION ( 'NONE',  ( -0.9876526153536336894, -0.1566598588826349503, 0.000000000000000000 ) ) ;
#12372=AXIS2_PLACEMENT_3D ( 'NONE', #2034, #12051, #4776 ) ;
#12374=CIRCLE ( 'NONE', #3006, 1.500000000000000888 ) ;
#12375=CIRCLE ( 'NONE', #4524, 1.500000000000000000 ) ;
#12376=ADVANCED_FACE ( 'NONE', ( #12342 ), #3905, .F. ) ;
#12377=DIRECTION ( 'NONE',  ( 0.000000000000000000, 0.000000000000000000, 1.000000000000000000 ) ) ;
#12378=CYLINDRICAL_SURFACE ( 'NONE', #6602, 1.500000000000001554 ) ;
#12379=EDGE_LOOP ( 'NONE', ( #7930, #1737, #18394, #1889 ) ) ;
#12380=FACE_OUTER_BOUND ( 'NONE', #4071, .T. ) ;
#12381=ADVANCED_FACE ( 'NONE', ( #6790 ), #12729, .F. ) ;
#12382=CARTESIAN_POINT ( 'NONE',  ( -37.15834831208948685, -26.14378280364935137, -4.330127018922181215 ) ) ;
#12383=DIRECTION ( 'NONE',  ( -0.1566598588826321192, 0.9876526153536342445, 7.798540720466731404E-17 ) ) ;
#12384=ORIENTED_EDGE ( 'NONE', *, *, #9011, .T. ) ;
#12385=AXIS2_PLACEMENT_3D ( 'NONE', #6891, #12629, #18490 ) ;
#12386=ADVANCED_FACE ( 'NONE', ( #1204 ), #4004, .F. ) ;
#12387=VECTOR ( 'NONE', #10002, 1000.000000000000000 ) ;
#12389=EDGE_CURVE ( 'NONE', #1477, #13575, #18292, .T. ) ;
#12390=VERTEX_POINT ( 'NONE', #15393 ) ;
#12392=ORIENTED_EDGE ( 'NONE', *, *, #9066, .T. ) ;
#12393=EDGE_LOOP ( 'NONE', ( #11553, #14598, #11099, #12546 ) ) ;
#12394=AXIS2_PLACEMENT_3D ( 'NONE', #17322, #15664, #11395 ) ;
#12396=DIRECTION ( 'NONE',  ( -0.1566598588826321192, 0.9876526153536342445, 7.798540720466730171E-17 ) ) ;
#12397=DIRECTION ( 'NONE',  ( -0.1566598588826321192, 0.9876526153536342445, 7.798540720466730171E-17 ) ) ;
#12399=CARTESIAN_POINT ( 'NONE',  ( -4.361458684479201153, -15.87908452487173427, 17.32050807568881368 ) ) ;
#12400=AXIS2_PLACEMENT_3D ( 'NONE', #3092, #14661, #10109 ) ;
#12401=CARTESIAN_POINT ( 'NONE',  ( -81.73462711737164454, 33.01666666666666572, -30.00000000000000000 ) ) ;
#12403=CARTESIAN_POINT ( 'NONE',  ( -34.68921677370540380, -25.75213315644277046, -17.32050807568878170 ) ) ;
#12405=AXIS2_PLACEMENT_3D ( 'NONE', #3983, #15269, #18270 ) ;
#12407=DIRECTION ( 'NONE',  ( 0.000000000000000000, 0.000000000000000000, 1.000000000000000000 ) ) ;
#12408=VECTOR ( 'NONE', #6178, 1000.000000000000000 ) ;
#12414=AXIS2_PLACEMENT_3D ( 'NONE', #1315, #7100, #4022 ) ;
#12415=ORIENTED_EDGE ( 'NONE', *, *, #18701, .T. ) ;
#12417=AXIS2_PLACEMENT_3D ( 'NONE', #10103, #4234, #10014 ) ;
#12418=FACE_BOUND ( 'NONE', #15173, .T. ) ;
#12419=ADVANCED_FACE ( 'NONE', ( #1023 ), #18584, .F. ) ;
#12421=AXIS2_PLACEMENT_3D ( 'NONE', #17541, #3240, #10117 ) ;
#12422=VECTOR ( 'NONE', #9901, 1000.000000000000000 ) ;
#12423=DIRECTION ( 'NONE',  ( -0.1566598588826321192, 0.9876526153536342445, 7.798540720466731404E-17 ) ) ;
#12424=CARTESIAN_POINT ( 'NONE',  ( -66.08974714408108753, -25.67032570503622324, 4.330127018922218518 ) ) ;
#12425=EDGE_LOOP ( 'NONE', ( #14659, #645 ) ) ;
#12426=AXIS2_PLACEMENT_3D ( 'NONE', #8336, #1336, #4249 ) ;
#12427=LINE ( 'NONE', #8360, #4245 ) ;
#12428=CIRCLE ( 'NONE', #18239, 1.500000000000001332 ) ;
#12429=CARTESIAN_POINT ( 'NONE',  ( -54.73174206751433957, -23.86873732788595603, -12.99038105676658006 ) ) ;
#12431=LINE ( 'NONE', #5334, #7150 ) ;
#12432=ORIENTED_EDGE ( 'NONE', *, *, #17724, .T. ) ;
#12433=ORIENTED_EDGE ( 'NONE', *, *, #4343, .F. ) ;
#12434=CARTESIAN_POINT ( 'NONE',  ( -6.830590222863280658, -16.27073417207831696, -12.99038105676658006 ) ) ;
#12435=AXIS2_PLACEMENT_3D ( 'NONE', #12817, #17206, #9972 ) ;
#12437=AXIS2_PLACEMENT_3D ( 'NONE', #16527, #3521, #9318 ) ;
#12438=VERTEX_POINT ( 'NONE', #8299 ) ;
#12440=FACE_OUTER_BOUND ( 'NONE', #7509, .T. ) ;
#12441=DIRECTION ( 'NONE',  ( -0.9876526153536336894, -0.1566598588826349503, 0.000000000000000000 ) ) ;
#12442=EDGE_CURVE ( 'NONE', #17604, #13102, #3003, .T. ) ;
#12443=VECTOR ( 'NONE', #8039, 1000.000000000000000 ) ;
#12444=AXIS2_PLACEMENT_3D ( 'NONE', #8749, #14632, #217 ) ;
#12445=DIRECTION ( 'NONE',  ( -0.9876526153536344665, -0.1566598588826304539, 0.000000000000000000 ) ) ;
#12447=EDGE_CURVE ( 'NONE', #8907, #1459, #16031, .T. ) ;
#12448=CARTESIAN_POINT ( 'NONE',  ( -14.93616446663280328, -22.61893597879013740, 1.869203119972154228E-14 ) ) ;
#12450=EDGE_CURVE ( 'NONE', #8310, #15166, #14634, .T. ) ;
#12451=LINE ( 'NONE', #5259, #5116 ) ;
#12453=AXIS2_PLACEMENT_3D ( 'NONE', #1270, #7325, #12802 ) ;
#12454=DIRECTION ( 'NONE',  ( -0.9876526153536336894, -0.1566598588826349503, 0.000000000000000000 ) ) ;
#12455=CARTESIAN_POINT ( 'NONE',  ( 3.868870235264020963, -77.34158009636824715, -8.660254037844389075 ) ) ;
#12456=CYLINDRICAL_SURFACE ( 'NONE', #12959, 1.500000000000000666 ) ;
#12458=DIRECTION ( 'NONE',  ( -0.1566598588826321192, 0.9876526153536342445, 7.798540720466731404E-17 ) ) ;
#12459=ORIENTED_EDGE ( 'NONE', *, *, #11233, .F. ) ;
#12461=CARTESIAN_POINT ( 'NONE',  ( -60.32854976272193426, -87.52447092373932946, 8.660254037844412167 ) ) ;
#12463=ORIENTED_EDGE ( 'NONE', *, *, #5223, .T. ) ;
#12465=DIRECTION ( 'NONE',  ( -0.1566598588826321192, 0.9876526153536342445, 7.798540720466730171E-17 ) ) ;
#12466=VERTEX_POINT ( 'NONE', #8751 ) ;
#12467=ORIENTED_EDGE ( 'NONE', *, *, #11352, .F. ) ;
#12468=ORIENTED_EDGE ( 'NONE', *, *, #3929, .F. ) ;
#12469=DIRECTION ( 'NONE',  ( -0.1566598588826321747, 0.9876526153536343555, 0.000000000000000000 ) ) ;
#12470=CARTESIAN_POINT ( 'NONE',  ( -36.62488699423479943, -83.76463431055617548, 21.65063509461101532 ) ) ;
#12471=CARTESIAN_POINT ( 'NONE',  ( -59.38053215754616332, -29.66862962850856533, -8.660254037844380193 ) ) ;
#12472=CARTESIAN_POINT ( 'NONE',  ( -10.98555400521827607, -21.99229654325962002, 4.330127018922214077 ) ) ;
#12473=CARTESIAN_POINT ( 'NONE',  ( -44.85521591397804997, -22.30213873905963595, -21.65063509461098334 ) ) ;
#12474=CARTESIAN_POINT ( 'NONE',  ( -44.07191661956489526, -27.24040181582777009, -21.65063509461098334 ) ) ;
#12475=DIRECTION ( 'NONE',  ( -0.1566598588826321192, 0.9876526153536342445, 7.798540720466730171E-17 ) ) ;
#12476=EDGE_CURVE ( 'NONE', #14720, #12880, #4520, .T. ) ;
#12478=CYLINDRICAL_SURFACE ( 'NONE', #8853, 1.500000000000000666 ) ;
#12479=CIRCLE ( 'NONE', #13685, 1.500000000000000888 ) ;
#12480=DIRECTION ( 'NONE',  ( -0.9876526153536336894, -0.1566598588826349503, 0.000000000000000000 ) ) ;
#12481=EDGE_LOOP ( 'NONE', ( #1652, #13320 ) ) ;
#12483=CARTESIAN_POINT ( 'NONE',  ( -57.36559191666103175, -87.05449134709142811, 8.660254037844412167 ) ) ;
#12485=DIRECTION ( 'NONE',  ( 0.000000000000000000, 0.000000000000000000, 1.000000000000000000 ) ) ;
#12486=EDGE_CURVE ( 'NONE', #2560, #1541, #9071, .T. ) ;
#12488=DIRECTION ( 'NONE',  ( -0.9876526153536344665, -0.1566598588826304539, 0.000000000000000000 ) ) ;
#12489=EDGE_LOOP ( 'NONE', ( #18455, #13955, #9209, #10505 ) ) ;
#12490=ORIENTED_EDGE ( 'NONE', *, *, #9898, .T. ) ;
#12491=CARTESIAN_POINT ( 'NONE',  ( -24.11451099155181055, -19.01228170252437977, 17.32050807568882078 ) ) ;
#12492=ORIENTED_EDGE ( 'NONE', *, *, #15138, .F. ) ;
#12493=DIRECTION ( 'NONE',  ( -0.9876526153536341335, -0.1566598588826327021, 0.000000000000000000 ) ) ;
#12495=CARTESIAN_POINT ( 'NONE',  ( -28.26947477390680774, -24.73384407370567217, 8.660254037844417496 ) ) ;
#12496=ADVANCED_FACE ( 'NONE', ( #7356 ), #3064, .F. ) ;
#12497=EDGE_CURVE ( 'NONE', #15027, #10665, #17571, .T. ) ;
#12500=CARTESIAN_POINT ( 'NONE',  ( 5.350349158294472218, -77.10659030804430358, 1.077796531449093893E-14 ) ) ;
#12501=EDGE_CURVE ( 'NONE', #15663, #16739, #14268, .T. ) ;
#12502=CARTESIAN_POINT ( 'NONE',  ( -4.361458684479201153, -15.87908452487173427, 8.660254037844412167 ) ) ;
#12503=CARTESIAN_POINT ( 'NONE',  ( -78.43540483600145308, -27.62857394106911002, -17.32050807568878170 ) ) ;
#12504=AXIS2_PLACEMENT_3D ( 'NONE', #11969, #4522, #13140 ) ;
#12505=CYLINDRICAL_SURFACE ( 'NONE', #8709, 1.500000000000001554 ) ;
#12507=EDGE_LOOP ( 'NONE', ( #1007, #4187, #5989, #16356 ) ) ;
#12508=ORIENTED_EDGE ( 'NONE', *, *, #18557, .F. ) ;
#12509=ORIENTED_EDGE ( 'NONE', *, *, #5567, .T. ) ;
#12511=FACE_BOUND ( 'NONE', #6459, .T. ) ;
#12512=CIRCLE ( 'NONE', #4353, 1.500000000000000888 ) ;
#12513=DIRECTION ( 'NONE',  ( -0.1566598588826321747, 0.9876526153536343555, 0.000000000000000000 ) ) ;
#12514=DIRECTION ( 'NONE',  ( -6.505213034913026604E-17, -0.000000000000000000, 1.000000000000000000 ) ) ;
#12517=CARTESIAN_POINT ( 'NONE',  ( -49.50400600400986661, -28.10203103968224880, 1.869203119972154228E-14 ) ) ;
#12518=DIRECTION ( 'NONE',  ( -0.9876526153536341335, -0.1566598588826327021, 0.000000000000000000 ) ) ;
#12519=DIRECTION ( 'NONE',  ( -0.1566598588826321192, 0.9876526153536342445, 7.798540720466730171E-17 ) ) ;
#12520=LINE ( 'NONE', #18362, #15686 ) ;
#12521=FACE_OUTER_BOUND ( 'NONE', #7615, .T. ) ;
#12522=EDGE_LOOP ( 'NONE', ( #5091, #10250 ) ) ;
#12523=DIRECTION ( 'NONE',  ( -0.1566598588826321192, 0.9876526153536342445, 7.798540720466730171E-17 ) ) ;
#12525=EDGE_LOOP ( 'NONE', ( #2424, #14119 ) ) ;
#12526=VERTEX_POINT ( 'NONE', #1654 ) ;
#12528=CARTESIAN_POINT ( 'NONE',  ( -15.88418207180859021, -80.47477727402088021, -17.32050807568878525 ) ) ;
#12530=ORIENTED_EDGE ( 'NONE', *, *, #5923, .T. ) ;
#12531=DIRECTION ( 'NONE',  ( -0.1566598588826321192, 0.9876526153536342445, 7.798540720466731404E-17 ) ) ;
#12533=ORIENTED_EDGE ( 'NONE', *, *, #11006, .F. ) ;
#12534=DIRECTION ( 'NONE',  ( -0.1566598588826321192, 0.9876526153536342445, 7.798540720466730171E-17 ) ) ;
#12536=DIRECTION ( 'NONE',  ( -0.1566598588826321192, 0.9876526153536342445, 7.798540720466730171E-17 ) ) ;
#12537=EDGE_CURVE ( 'NONE', #12880, #14720, #15455, .T. ) ;
#12538=DIRECTION ( 'NONE',  ( -0.9876526153536341335, -0.1566598588826327021, 0.000000000000000000 ) ) ;
#12540=ORIENTED_EDGE ( 'NONE', *, *, #12052, .T. ) ;
#12542=ORIENTED_EDGE ( 'NONE', *, *, #8453, .T. ) ;
#12543=DIRECTION ( 'NONE',  ( -0.1566598588826321192, 0.9876526153536342445, 7.798540720466731404E-17 ) ) ;
#12544=ORIENTED_EDGE ( 'NONE', *, *, #12296, .T. ) ;
#12545=EDGE_CURVE ( 'NONE', #6414, #10326, #17588, .T. ) ;
#12546=ORIENTED_EDGE ( 'NONE', *, *, #9539, .F. ) ;
#12547=ORIENTED_EDGE ( 'NONE', *, *, #5814, .F. ) ;
#12548=DIRECTION ( 'NONE',  ( -0.1566598588826321747, 0.9876526153536343555, 0.000000000000000000 ) ) ;
#12550=DIRECTION ( 'NONE',  ( -0.1566598588826321747, 0.9876526153536343555, 0.000000000000000000 ) ) ;
#12551=VERTEX_POINT ( 'NONE', #4203 ) ;
#12552=CARTESIAN_POINT ( 'NONE',  ( -76.95392591297100182, -27.39358415274518066, 17.32050807568881723 ) ) ;
#12553=DIRECTION ( 'NONE',  ( -0.1566598588826321192, 0.9876526153536342445, 7.798540720466730171E-17 ) ) ;
#12554=CARTESIAN_POINT ( 'NONE',  ( -29.21749237908258223, -82.58968536893642920, 8.660254037844412167 ) ) ;
#12555=FACE_OUTER_BOUND ( 'NONE', #1260, .T. ) ;
#12556=EDGE_LOOP ( 'NONE', ( #17613, #18456 ) ) ;
#12557=CARTESIAN_POINT ( 'NONE',  ( -53.74408945216069355, -23.71207746900333291, 17.32050807568882078 ) ) ;
#12558=EDGE_LOOP ( 'NONE', ( #11839, #7362 ) ) ;
#12559=DIRECTION ( 'NONE',  ( -0.1566598588826321192, 0.9876526153536342445, 7.798540720466730171E-17 ) ) ;
#12563=CARTESIAN_POINT ( 'NONE',  ( 2.000000000000000000, 2.449293598294706414E-16, -24.99999999999999289 ) ) ;
#12564=ORIENTED_EDGE ( 'NONE', *, *, #15569, .F. ) ;
#12565=EDGE_LOOP ( 'NONE', ( #16436, #14506 ) ) ;
#12566=ADVANCED_FACE ( 'NONE', ( #9986 ), #15781, .F. ) ;
#12567=DIRECTION ( 'NONE',  ( -0.1566598588826321747, 0.9876526153536343555, 0.000000000000000000 ) ) ;
#12568=ORIENTED_EDGE ( 'NONE', *, *, #8503, .F. ) ;
#12569=ORIENTED_EDGE ( 'NONE', *, *, #10175, .F. ) ;
#12572=EDGE_CURVE ( 'NONE', #14170, #15556, #10284, .T. ) ;
#12573=VERTEX_POINT ( 'NONE', #14715 ) ;
#12574=DIRECTION ( 'NONE',  ( -0.1566598588826321192, 0.9876526153536342445, 7.798540720466731404E-17 ) ) ;
#12576=CARTESIAN_POINT ( 'NONE',  ( -28.22983976372896109, -82.43302551005379541, -4.330127018922185655 ) ) ;
#12577=CARTESIAN_POINT ( 'NONE',  ( -43.08426400421124924, -27.08374195694514341, 1.869203119972154228E-14 ) ) ;
#12578=LINE ( 'NONE', #18439, #2686 ) ;
#12579=DIRECTION ( 'NONE',  ( -0.9876526153536341335, -0.1566598588826327021, 0.000000000000000000 ) ) ;
#12581=DIRECTION ( 'NONE',  ( -0.9876526153536336894, -0.1566598588826350336, 0.000000000000000000 ) ) ;
#12583=CIRCLE ( 'NONE', #9574, 1.500000000000001332 ) ;
#12586=EDGE_CURVE ( 'NONE', #14892, #5886, #16236, .T. ) ;
#12587=CIRCLE ( 'NONE', #8968, 1.500000000000001332 ) ;
#12588=ORIENTED_EDGE ( 'NONE', *, *, #909, .T. ) ;
#12589=FACE_OUTER_BOUND ( 'NONE', #7394, .T. ) ;
#12590=EDGE_CURVE ( 'NONE', #14949, #18590, #7712, .T. ) ;
#12592=ORIENTED_EDGE ( 'NONE', *, *, #12450, .T. ) ;
#12593=FACE_BOUND ( 'NONE', #3426, .T. ) ;
#12594=EDGE_CURVE ( 'NONE', #9193, #13266, #9305, .T. ) ;
#12596=AXIS2_PLACEMENT_3D ( 'NONE', #18642, #9948, #14870 ) ;
#12598=ORIENTED_EDGE ( 'NONE', *, *, #5945, .T. ) ;
#12599=CIRCLE ( 'NONE', #15640, 1.500000000000001332 ) ;
#12601=EDGE_LOOP ( 'NONE', ( #10615, #1998 ) ) ;
#12602=AXIS2_PLACEMENT_3D ( 'NONE', #16875, #18326, #5205 ) ;
#12603=DIRECTION ( 'NONE',  ( -0.1566598588826321192, 0.9876526153536342445, 7.798540720466730171E-17 ) ) ;
#12604=FACE_OUTER_BOUND ( 'NONE', #2919, .T. ) ;
#12605=AXIS2_PLACEMENT_3D ( 'NONE', #12363, #12263, #7838 ) ;
#12606=CARTESIAN_POINT ( 'NONE',  ( -37.15834831208949396, -26.14378280364935137, -21.65063509461098334 ) ) ;
#12608=CYLINDRICAL_SURFACE ( 'NONE', #14187, 1.500000000000001554 ) ;
#12609=EDGE_LOOP ( 'NONE', ( #15306, #8146, #10336, #9968 ) ) ;
#12610=EDGE_CURVE ( 'NONE', #5860, #7782, #17972, .T. ) ;
#12611=CARTESIAN_POINT ( 'NONE',  ( -58.88670584986932255, -29.59029969906724133, 21.65063509461101887 ) ) ;
#12612=ORIENTED_EDGE ( 'NONE', *, *, #16728, .F. ) ;
#12613=EDGE_LOOP ( 'NONE', ( #4232, #6429, #8961, #16556 ) ) ;
#12615=EDGE_CURVE ( 'NONE', #12954, #14743, #18524, .T. ) ;
#12617=EDGE_LOOP ( 'NONE', ( #3360, #17726, #15543, #16466 ) ) ;
#12619=CIRCLE ( 'NONE', #7498, 1.499999999999999556 ) ;
#12622=DIRECTION ( 'NONE',  ( -0.1566598588826321192, 0.9876526153536342445, 7.798540720466730171E-17 ) ) ;
#12623=DIRECTION ( 'NONE',  ( -0.1566598588826321192, 0.9876526153536342445, 7.798540720466730171E-17 ) ) ;
#12624=AXIS2_PLACEMENT_3D ( 'NONE', #15721, #10119, #5954 ) ;
#12625=LINE ( 'NONE', #6793, #4480 ) ;
#12626=DIRECTION ( 'NONE',  ( -0.1566598588826321192, 0.9876526153536342445, 7.798540720466731404E-17 ) ) ;
#12627=ORIENTED_EDGE ( 'NONE', *, *, #8104, .F. ) ;
#12628=ORIENTED_EDGE ( 'NONE', *, *, #1191, .F. ) ;
#12629=DIRECTION ( 'NONE',  ( -0.1566598588826321192, 0.9876526153536342445, 7.798540720466731404E-17 ) ) ;
#12630=DIRECTION ( 'NONE',  ( 0.000000000000000000, 0.000000000000000000, 1.000000000000000000 ) ) ;
#12631=EDGE_LOOP ( 'NONE', ( #5327, #2291, #9473, #16767 ) ) ;
#12632=ORIENTED_EDGE ( 'NONE', *, *, #13759, .T. ) ;
#12633=VERTEX_POINT ( 'NONE', #3329 ) ;
#12636=DIRECTION ( 'NONE',  ( -0.1566598588826321192, 0.9876526153536342445, 7.798540720466730171E-17 ) ) ;
#12641=CIRCLE ( 'NONE', #15688, 1.500000000000000888 ) ;
#12642=VERTEX_POINT ( 'NONE', #13464 ) ;
#12643=DIRECTION ( 'NONE',  ( -0.1566598588826321192, 0.9876526153536342445, 7.798540720466731404E-17 ) ) ;
#12644=ADVANCED_FACE ( 'NONE', ( #18059 ), #1924, .F. ) ;
#12645=CARTESIAN_POINT ( 'NONE',  ( -14.40270314877813895, -80.23978748569695085, 17.32050807568881368 ) ) ;
#12646=PLANE ( 'NONE',  #10004 ) ;
#12647=CARTESIAN_POINT ( 'NONE',  ( -26.74836084069850983, -82.19803572172985184, 21.65063509461101532 ) ) ;
#12648=DIRECTION ( 'NONE',  ( -0.000000000000000000, -0.000000000000000000, -1.000000000000000000 ) ) ;
#12649=ORIENTED_EDGE ( 'NONE', *, *, #17635, .T. ) ;
#12650=VECTOR ( 'NONE', #11400, 1000.000000000000000 ) ;
#12651=DIRECTION ( 'NONE',  ( 0.000000000000000000, 0.000000000000000000, 1.000000000000000000 ) ) ;
#12652=AXIS2_PLACEMENT_3D ( 'NONE', #2746, #18628, #5597 ) ;
#12653=LINE ( 'NONE', #5668, #13542 ) ;
#12654=ORIENTED_EDGE ( 'NONE', *, *, #3481, .F. ) ;
#12655=DIRECTION ( 'NONE',  ( -0.1566598588826321192, 0.9876526153536342445, 7.798540720466730171E-17 ) ) ;
#12656=CYLINDRICAL_SURFACE ( 'NONE', #6963, 1.500000000000001554 ) ;
#12657=ORIENTED_EDGE ( 'NONE', *, *, #14128, .T. ) ;
#12659=ORIENTED_EDGE ( 'NONE', *, *, #6025, .F. ) ;
#12662=CARTESIAN_POINT ( 'NONE',  ( -27.73601345605213098, -82.35469558061248563, 17.32050807568881368 ) ) ;
#12663=EDGE_CURVE ( 'NONE', #1265, #12921, #506, .T. ) ;
#12665=CIRCLE ( 'NONE', #4510, 1.500000000000000888 ) ;
#12667=AXIS2_PLACEMENT_3D ( 'NONE', #6531, #14472, #4332 ) ;
#12668=ORIENTED_EDGE ( 'NONE', *, *, #2193, .T. ) ;
#12669=CYLINDRICAL_SURFACE ( 'NONE', #5519, 1.500000000000000666 ) ;
#12670=LINE ( 'NONE', #5307, #2049 ) ;
#12671=EDGE_CURVE ( 'NONE', #6385, #1601, #16335, .T. ) ;
#12673=DIRECTION ( 'NONE',  ( -0.9876526153536336894, -0.1566598588826350336, 0.000000000000000000 ) ) ;
#12674=CYLINDRICAL_SURFACE ( 'NONE', #7748, 1.500000000000001554 ) ;
#12676=FACE_OUTER_BOUND ( 'NONE', #3516, .T. ) ;
#12678=AXIS2_PLACEMENT_3D ( 'NONE', #15834, #9943, #11168 ) ;
#12679=ADVANCED_FACE ( 'NONE', ( #10714 ), #6300, .F. ) ;
#12681=VERTEX_POINT ( 'NONE', #4851 ) ;
#12685=AXIS2_PLACEMENT_3D ( 'NONE', #2649, #10124, #8440 ) ;
#12686=AXIS2_PLACEMENT_3D ( 'NONE', #15758, #1451, #10145 ) ;
#12687=ORIENTED_EDGE ( 'NONE', *, *, #15067, .T. ) ;
#12688=ORIENTED_EDGE ( 'NONE', *, *, #12138, .T. ) ;
#12690=CARTESIAN_POINT ( 'NONE',  ( 2.349859322727720023, -14.81454612788783898, -1.559688948638727718E-15 ) ) ;
#12692=LINE ( 'NONE', #7977, #8661 ) ;
#12694=CIRCLE ( 'NONE', #13002, 1.500000000000000444 ) ;
#12695=ORIENTED_EDGE ( 'NONE', *, *, #738, .F. ) ;
#12696=VECTOR ( 'NONE', #7521, 1000.000000000000000 ) ;
#12697=EDGE_CURVE ( 'NONE', #2990, #8283, #9027, .T. ) ;
#12698=AXIS2_PLACEMENT_3D ( 'NONE', #12107, #3575, #13717 ) ;
#12699=CARTESIAN_POINT ( 'NONE',  ( -37.15834831208948685, -26.14378280364935137, 21.65063509461101887 ) ) ;
#12701=EDGE_LOOP ( 'NONE', ( #624, #6202 ) ) ;
#12702=DIRECTION ( 'NONE',  ( -0.9876526153536341335, -0.1566598588826327021, 0.000000000000000000 ) ) ;
#12704=CARTESIAN_POINT ( 'NONE',  ( -9.997901389864651378, -21.83563668437698269, -17.32050807568878170 ) ) ;
#12705=EDGE_CURVE ( 'NONE', #16637, #14520, #3021, .T. ) ;
#12707=ORIENTED_EDGE ( 'NONE', *, *, #5337, .F. ) ;
#12708=DIRECTION ( 'NONE',  ( -0.1566598588826321192, 0.9876526153536342445, 7.798540720466730171E-17 ) ) ;
#12709=CIRCLE ( 'NONE', #5470, 1.500000000000000888 ) ;
#12710=VERTEX_POINT ( 'NONE', #11857 ) ;
#12711=ORIENTED_EDGE ( 'NONE', *, *, #12671, .T. ) ;
#12712=ORIENTED_EDGE ( 'NONE', *, *, #2238, .T. ) ;
#12713=AXIS2_PLACEMENT_3D ( 'NONE', #16033, #11283, #5715 ) ;
#12714=DIRECTION ( 'NONE',  ( -0.9876526153536336894, -0.1566598588826349503, 0.000000000000000000 ) ) ;
#12715=VERTEX_POINT ( 'NONE', #17694 ) ;
#12718=VECTOR ( 'NONE', #17135, 1000.000000000000000 ) ;
#12719=DIRECTION ( 'NONE',  ( -0.1566598588826321192, 0.9876526153536342445, 7.798540720466730171E-17 ) ) ;
#12721=DIRECTION ( 'NONE',  ( -0.1566598588826321192, 0.9876526153536342445, 7.798540720466730171E-17 ) ) ;
#12722=LINE ( 'NONE', #4090, #14232 ) ;
#12723=CIRCLE ( 'NONE', #12414, 1.500000000000000888 ) ;
#12724=AXIS2_PLACEMENT_3D ( 'NONE', #249, #6037, #8520 ) ;
#12725=DIRECTION ( 'NONE',  ( -0.1566598588826321192, 0.9876526153536342445, 7.798540720466731404E-17 ) ) ;
#12728=EDGE_CURVE ( 'NONE', #17816, #8900, #6688, .T. ) ;
#12729=CYLINDRICAL_SURFACE ( 'NONE', #7283, 1.500000000000001554 ) ;
#12730=CYLINDRICAL_SURFACE ( 'NONE', #9381, 1.500000000000001554 ) ;
#12731=FACE_OUTER_BOUND ( 'NONE', #6384, .T. ) ;
#12732=ADVANCED_FACE ( 'NONE', ( #7625 ), #13383, .F. ) ;
#12736=ORIENTED_EDGE ( 'NONE', *, *, #15864, .T. ) ;
#12737=CARTESIAN_POINT ( 'NONE',  ( -55.39028668595377525, -86.74117162932617475, 17.32050807568881368 ) ) ;
#12738=CARTESIAN_POINT ( 'NONE',  ( -57.85941822433786541, -87.13282127653273790, 4.330127018922213189 ) ) ;
#12739=ADVANCED_FACE ( 'NONE', ( #17011 ), #15366, .F. ) ;
#12740=LINE ( 'NONE', #10453, #6381 ) ;
#12742=VECTOR ( 'NONE', #4194, 1000.000000000000000 ) ;
#12743=CARTESIAN_POINT ( 'NONE',  ( -68.55887868246516348, -26.06197535224279349, -17.32050807568878170 ) ) ;
#12745=LINE ( 'NONE', #3733, #5496 ) ;
#12746=AXIS2_PLACEMENT_3D ( 'NONE', #2078, #16302, #7768 ) ;
#12747=CARTESIAN_POINT ( 'NONE',  ( -30.20514499443620338, -82.74634522781904877, 21.65063509461101532 ) ) ;
#12749=ORIENTED_EDGE ( 'NONE', *, *, #1298, .F. ) ;
#12751=FACE_OUTER_BOUND ( 'NONE', #7934, .T. ) ;
#12752=DIRECTION ( 'NONE',  ( 0.000000000000000000, 0.000000000000000000, 1.000000000000000000 ) ) ;
#12755=CIRCLE ( 'NONE', #15806, 1.499999999999999556 ) ;
#12756=EDGE_CURVE ( 'NONE', #16064, #9762, #17904, .T. ) ;
#12758=ORIENTED_EDGE ( 'NONE', *, *, #878, .T. ) ;
#12759=CARTESIAN_POINT ( 'NONE',  ( -37.44782129882580080, -21.12718979743990388, -8.660254037844380193 ) ) ;
#12760=DIRECTION ( 'NONE',  ( -0.1566598588826321747, 0.9876526153536343555, 0.000000000000000000 ) ) ;
#12762=ORIENTED_EDGE ( 'NONE', *, *, #145, .F. ) ;
#12764=CARTESIAN_POINT ( 'NONE',  ( -23.29157668696081629, -81.64972621564065491, 21.65063509461101532 ) ) ;
#12766=CARTESIAN_POINT ( 'NONE',  ( -79.91688375903190433, -27.86356372939306070, -8.660254037844380193 ) ) ;
#12767=CYLINDRICAL_SURFACE ( 'NONE', #16968, 1.500000000000001554 ) ;
#12768=EDGE_LOOP ( 'NONE', ( #15401, #542 ) ) ;
#12770=CIRCLE ( 'NONE', #1296, 1.500000000000000888 ) ;
#12771=EDGE_CURVE ( 'NONE', #8399, #968, #937, .T. ) ;
#12772=CARTESIAN_POINT ( 'NONE',  ( 1.360103686702108128, -20.03404830722672259, 8.660254037844412167 ) ) ;
#12773=ORIENTED_EDGE ( 'NONE', *, *, #1108, .T. ) ;
#12776=DIRECTION ( 'NONE',  ( -0.1566598588826321747, 0.9876526153536343555, 0.000000000000000000 ) ) ;
#12777=VERTEX_POINT ( 'NONE', #16817 ) ;
#12779=VECTOR ( 'NONE', #11278, 1000.000000000000000 ) ;
#12781=DIRECTION ( 'NONE',  ( -0.1566598588826321192, 0.9876526153536342445, 7.798540720466730171E-17 ) ) ;
#12783=CARTESIAN_POINT ( 'NONE',  ( -35.67686938905902849, -25.90879301532540779, 4.330127018922217630 ) ) ;
#12784=FACE_OUTER_BOUND ( 'NONE', #6735, .T. ) ;
#12785=VERTEX_POINT ( 'NONE', #6769 ) ;
#12787=DIRECTION ( 'NONE',  ( -0.1566598588826321192, 0.9876526153536342445, 7.798540720466731404E-17 ) ) ;
#12788=DIRECTION ( 'NONE',  ( -0.1566598588826321192, 0.9876526153536342445, 7.798540720466730171E-17 ) ) ;
#12789=CARTESIAN_POINT ( 'NONE',  ( -67.73594437787414790, -88.69941986535906153, 4.330127018922213189 ) ) ;
#12790=ORIENTED_EDGE ( 'NONE', *, *, #131, .T. ) ;
#12792=EDGE_LOOP ( 'NONE', ( #4733, #10227 ) ) ;
#12793=ORIENTED_EDGE ( 'NONE', *, *, #19, .T. ) ;
#12795=CARTESIAN_POINT ( 'NONE',  ( -39.09401853261888959, -84.15628395776273862, 1.424741226644455312E-14 ) ) ;
#12796=AXIS2_PLACEMENT_3D ( 'NONE', #17689, #6293, #696 ) ;
#12797=ORIENTED_EDGE ( 'NONE', *, *, #17686, .T. ) ;
#12798=ORIENTED_EDGE ( 'NONE', *, *, #12221, .T. ) ;
#12799=DIRECTION ( 'NONE',  ( -0.1566598588826321747, 0.9876526153536343555, 0.000000000000000000 ) ) ;
#12800=ADVANCED_FACE ( 'NONE', ( #2495 ), #6859, .F. ) ;
#12801=ORIENTED_EDGE ( 'NONE', *, *, #5302, .T. ) ;
#12802=DIRECTION ( 'NONE',  ( -0.9876526153536336894, -0.1566598588826349503, 0.000000000000000000 ) ) ;
#12803=CARTESIAN_POINT ( 'NONE',  ( -45.55339554259533230, -27.47539160415171722, -12.99038105676658006 ) ) ;
#12804=ORIENTED_EDGE ( 'NONE', *, *, #15064, .T. ) ;
#12805=CIRCLE ( 'NONE', #14325, 1.499999999999999556 ) ;
#12806=CARTESIAN_POINT ( 'NONE',  ( -63.78533391645962780, -88.07278042982854060, 17.32050807568881368 ) ) ;
#12807=FACE_BOUND ( 'NONE', #16221, .T. ) ;
#12808=CARTESIAN_POINT ( 'NONE',  ( -74.19532138785061193, -32.01852751174804013, 17.32050807568881723 ) ) ;
#12809=CARTESIAN_POINT ( 'NONE',  ( -57.36559191666103175, -87.05449134709142811, 17.32050807568881368 ) ) ;
#12810=CARTESIAN_POINT ( 'NONE',  ( -57.89905323451571206, -29.43363984018462176, -17.32050807568878170 ) ) ;
#12812=DIRECTION ( 'NONE',  ( -0.9876526153536336894, -0.1566598588826349503, 0.000000000000000000 ) ) ;
#12813=ORIENTED_EDGE ( 'NONE', *, *, #16350, .F. ) ;
#12814=ORIENTED_EDGE ( 'NONE', *, *, #13562, .F. ) ;
#12816=ORIENTED_EDGE ( 'NONE', *, *, #15768, .F. ) ;
#12817=CARTESIAN_POINT ( 'NONE',  ( -41.56315007100294423, -84.54793360496933019, 21.65063509461101532 ) ) ;
#12818=AXIS2_PLACEMENT_3D ( 'NONE', #7567, #1960, #7667 ) ;
#12819=EDGE_CURVE ( 'NONE', #13293, #7092, #1242, .T. ) ;
#12820=EDGE_LOOP ( 'NONE', ( #7535, #18568, #5348, #18251 ) ) ;
#12824=DIRECTION ( 'NONE',  ( 0.000000000000000000, 0.000000000000000000, 1.000000000000000000 ) ) ;
#12829=DIRECTION ( 'NONE',  ( -0.9876526153536341335, -0.1566598588826327021, 0.000000000000000000 ) ) ;
#12833=DIRECTION ( 'NONE',  ( -0.1566598588826321192, 0.9876526153536342445, 7.798540720466730171E-17 ) ) ;
#12834=CARTESIAN_POINT ( 'NONE',  ( -49.01017969633302584, -28.02370111024093191, 4.330127018922217630 ) ) ;
#12835=DIRECTION ( 'NONE',  ( -0.1566598588826321192, 0.9876526153536342445, 7.798540720466730171E-17 ) ) ;
#12837=ORIENTED_EDGE ( 'NONE', *, *, #8729, .T. ) ;
#12838=DIRECTION ( 'NONE',  ( -0.1566598588826321192, 0.9876526153536342445, 7.798540720466731404E-17 ) ) ;
#12840=EDGE_CURVE ( 'NONE', #4741, #10340, #5149, .T. ) ;
#12841=DIRECTION ( 'NONE',  ( 0.000000000000000000, 0.000000000000000000, 1.000000000000000000 ) ) ;
#12842=EDGE_CURVE ( 'NONE', #8644, #11461, #12427, .T. ) ;
#12844=FACE_OUTER_BOUND ( 'NONE', #14275, .T. ) ;
#12845=CIRCLE ( 'NONE', #8914, 1.499999999999999556 ) ;
#12846=FACE_OUTER_BOUND ( 'NONE', #11542, .T. ) ;
#12847=ORIENTED_EDGE ( 'NONE', *, *, #8465, .T. ) ;
#12848=DIRECTION ( 'NONE',  ( -0.9876526153536341335, -0.1566598588826327021, 0.000000000000000000 ) ) ;
#12849=EDGE_LOOP ( 'NONE', ( #1149, #4590, #16911, #15299 ) ) ;
#12850=LINE ( 'NONE', #18694, #1424 ) ;
#12851=DIRECTION ( 'NONE',  ( -0.1566598588826321747, 0.9876526153536343555, 0.000000000000000000 ) ) ;
#12852=DIRECTION ( 'NONE',  ( -0.9876526153536336894, -0.1566598588826349503, 0.000000000000000000 ) ) ;
#12853=ORIENTED_EDGE ( 'NONE', *, *, #9124, .F. ) ;
#12854=DIRECTION ( 'NONE',  ( -0.1566598588826321192, 0.9876526153536342445, 7.798540720466731404E-17 ) ) ;
#12855=VERTEX_POINT ( 'NONE', #891 ) ;
#12856=EDGE_CURVE ( 'NONE', #5835, #15309, #16363, .T. ) ;
#12857=LINE ( 'NONE', #18703, #4531 ) ;
#12858=VECTOR ( 'NONE', #13682, 1000.000000000000000 ) ;
#12859=ORIENTED_EDGE ( 'NONE', *, *, #17170, .T. ) ;
#12860=ADVANCED_FACE ( 'NONE', ( #18360 ), #1179, .F. ) ;
#12861=EDGE_CURVE ( 'NONE', #794, #7971, #16684, .T. ) ;
#12862=ORIENTED_EDGE ( 'NONE', *, *, #6874, .T. ) ;
#12863=DIRECTION ( 'NONE',  ( -0.1566598588826321747, 0.9876526153536343555, 0.000000000000000000 ) ) ;
#12866=CARTESIAN_POINT ( 'NONE',  ( -61.84966369593023217, -30.06027927571513914, 21.65063509461101887 ) ) ;
#12868=CYLINDRICAL_SURFACE ( 'NONE', #6637, 1.500000000000000888 ) ;
#12869=AXIS2_PLACEMENT_3D ( 'NONE', #10542, #16339, #8181 ) ;
#12870=CARTESIAN_POINT ( 'NONE',  ( -46.33669483700847280, -22.53712852738359373, 12.99038105676661736 ) ) ;
#12872=CARTESIAN_POINT ( 'NONE',  ( -70.20507591625822386, -89.09106951256563889, 1.424741226644455312E-14 ) ) ;
#12873=ORIENTED_EDGE ( 'NONE', *, *, #17387, .F. ) ;
#12874=VERTEX_POINT ( 'NONE', #18559 ) ;
#12876=CYLINDRICAL_SURFACE ( 'NONE', #17263, 1.500000000000001554 ) ;
#12880=VERTEX_POINT ( 'NONE', #1449 ) ;
#12881=AXIS2_PLACEMENT_3D ( 'NONE', #13236, #5598, #8542 ) ;
#12884=CARTESIAN_POINT ( 'NONE',  ( -21.64537945316773460, -18.62063205531779531, -4.330127018922180326 ) ) ;
#12886=EDGE_CURVE ( 'NONE', #13905, #3864, #5621, .T. ) ;
#12888=AXIS2_PLACEMENT_3D ( 'NONE', #6563, #5414, #3777 ) ;
#12889=FACE_BOUND ( 'NONE', #12295, .T. ) ;
#12890=CARTESIAN_POINT ( 'NONE',  ( -41.60278508118079799, -26.84875216862118918, 17.32050807568881723 ) ) ;
#12891=AXIS2_PLACEMENT_3D ( 'NONE', #5481, #11241, #7190 ) ;
#12892=DIRECTION ( 'NONE',  ( -0.9876526153536336894, -0.1566598588826349503, 0.000000000000000000 ) ) ;
#12893=FACE_OUTER_BOUND ( 'NONE', #3443, .T. ) ;
#12894=ORIENTED_EDGE ( 'NONE', *, *, #12594, .F. ) ;
#12895=ORIENTED_EDGE ( 'NONE', *, *, #11748, .F. ) ;
#12896=ORIENTED_EDGE ( 'NONE', *, *, #17096, .T. ) ;
#12897=VERTEX_POINT ( 'NONE', #12890 ) ;
#12898=DIRECTION ( 'NONE',  ( 0.000000000000000000, 0.000000000000000000, 1.000000000000000000 ) ) ;
#12899=VECTOR ( 'NONE', #13076, 1000.000000000000000 ) ;
#12900=DIRECTION ( 'NONE',  ( -0.1566598588826321192, 0.9876526153536342445, 7.798540720466730171E-17 ) ) ;
#12901=CARTESIAN_POINT ( 'NONE',  ( 55.85952145814821534, 6.938893903907228378E-15, 30.00000000000000000 ) ) ;
#12904=CARTESIAN_POINT ( 'NONE',  ( -19.87442754340095519, -23.40223527320329922, -8.660254037844380193 ) ) ;
#12906=AXIS2_PLACEMENT_3D ( 'NONE', #3452, #7937, #3647 ) ;
#12907=DIRECTION ( 'NONE',  ( -0.1566598588826321192, 0.9876526153536342445, 7.798540720466730171E-17 ) ) ;
#12909=AXIS2_PLACEMENT_3D ( 'NONE', #9526, #15298, #8100 ) ;
#12912=CARTESIAN_POINT ( 'NONE',  ( -43.86756329862440396, -22.14547888017701283, 8.660254037844417496 ) ) ;
#12916=FACE_BOUND ( 'NONE', #16156, .T. ) ;
#12917=CARTESIAN_POINT ( 'NONE',  ( -37.61253960958842413, -83.92129416943879505, 8.660254037844412167 ) ) ;
#12918=AXIS2_PLACEMENT_3D ( 'NONE', #11585, #17406, #18759 ) ;
#12919=ADVANCED_FACE ( 'NONE', ( #7414 ), #18735, .F. ) ;
#12920=FACE_OUTER_BOUND ( 'NONE', #11649, .T. ) ;
#12921=VERTEX_POINT ( 'NONE', #17197 ) ;
#12922=ORIENTED_EDGE ( 'NONE', *, *, #14304, .F. ) ;
#12923=DIRECTION ( 'NONE',  ( 0.000000000000000000, 0.000000000000000000, 1.000000000000000000 ) ) ;
#12924=VECTOR ( 'NONE', #15604, 1000.000000000000000 ) ;
#12925=CARTESIAN_POINT ( 'NONE',  ( -28.26947477390680774, -24.73384407370567217, -17.32050807568878170 ) ) ;
#12926=CARTESIAN_POINT ( 'NONE',  ( -75.96627329761737712, -27.23692429386253266, -12.99038105676658006 ) ) ;
#12927=CARTESIAN_POINT ( 'NONE',  ( 2.058283315319403783, -14.86079544213463066, 1.406148482768655632E-14 ) ) ;
#12929=DIRECTION ( 'NONE',  ( -0.9876526153536341335, -0.1566598588826327021, 0.000000000000000000 ) ) ;
#12931=CIRCLE ( 'NONE', #15966, 1.500000000000001332 ) ;
#12932=ADVANCED_FACE ( 'NONE', ( #15643 ), #1636, .F. ) ;
#12933=CARTESIAN_POINT ( 'NONE',  ( -44.03228160938704860, -84.93958325217589334, -17.32050807568878525 ) ) ;
#12935=CARTESIAN_POINT ( 'NONE',  ( -44.03228160938704860, -84.93958325217589334, -8.660254037844385522 ) ) ;
#12936=DIRECTION ( 'NONE',  ( -0.1566598588826321192, 0.9876526153536342445, 7.798540720466730171E-17 ) ) ;
#12938=DIRECTION ( 'NONE',  ( -0.1566598588826321192, 0.9876526153536342445, 7.798540720466730171E-17 ) ) ;
#12940=ORIENTED_EDGE ( 'NONE', *, *, #3450, .F. ) ;
#12941=FACE_OUTER_BOUND ( 'NONE', #7321, .T. ) ;
#12943=EDGE_CURVE ( 'NONE', #13071, #5613, #633, .T. ) ;
#12944=AXIS2_PLACEMENT_3D ( 'NONE', #14289, #8604, #5767 ) ;
#12945=CARTESIAN_POINT ( 'NONE',  ( 3.133606229046292935, -19.12225244224100962, 24.99999999999998934 ) ) ;
#12946=ADVANCED_FACE ( 'NONE', ( #12987 ), #8734, .F. ) ;
#12947=EDGE_LOOP ( 'NONE', ( #13302, #397 ) ) ;
#12951=CARTESIAN_POINT ( 'NONE',  ( -20.16390053013728334, -18.38564226699385529, 21.65063509461101177 ) ) ;
#12952=EDGE_CURVE ( 'NONE', #626, #18004, #4458, .T. ) ;
#12953=CIRCLE ( 'NONE', #4180, 1.500000000000000888 ) ;
#12954=VERTEX_POINT ( 'NONE', #2670 ) ;
#12956=CARTESIAN_POINT ( 'NONE',  ( -7.034943543803747090, -21.36565710772908488, -8.660254037844380193 ) ) ;
#12957=VECTOR ( 'NONE', #4002, 1000.000000000000000 ) ;
#12958=LINE ( 'NONE', #7393, #6333 ) ;
#12959=AXIS2_PLACEMENT_3D ( 'NONE', #4099, #7084, #18294 ) ;
#12960=DIRECTION ( 'NONE',  ( -0.9876526153536341335, -0.1566598588826327021, 0.000000000000000000 ) ) ;
#12961=EDGE_CURVE ( 'NONE', #9249, #3229, #15149, .T. ) ;
#12962=DIRECTION ( 'NONE',  ( -0.9876526153536344665, -0.1566598588826304539, 0.000000000000000000 ) ) ;
#12963=EDGE_CURVE ( 'NONE', #15692, #4549, #17601, .T. ) ;
#12964=CARTESIAN_POINT ( 'NONE',  ( -48.80582637539256297, -22.92877817459016754, 1.908195823574487804E-14 ) ) ;
#12965=DIRECTION ( 'NONE',  ( -0.1566598588826321192, 0.9876526153536342445, 7.798540720466730171E-17 ) ) ;
#12966=DIRECTION ( 'NONE',  ( -0.1566598588826321192, 0.9876526153536342445, 7.798540720466731404E-17 ) ) ;
#12967=ORIENTED_EDGE ( 'NONE', *, *, #2271, .F. ) ;
#12968=EDGE_CURVE ( 'NONE', #14954, #2218, #5473, .T. ) ;
#12969=VECTOR ( 'NONE', #5978, 1000.000000000000000 ) ;
#12970=ORIENTED_EDGE ( 'NONE', *, *, #81, .T. ) ;
#12971=CARTESIAN_POINT ( 'NONE',  ( -79.24244631363546887, 32.81909429640987952, 35.00000000000000000 ) ) ;
#12972=EDGE_LOOP ( 'NONE', ( #17165, #2029, #7733, #11254 ) ) ;
#12973=VERTEX_POINT ( 'NONE', #1548 ) ;
#12974=ORIENTED_EDGE ( 'NONE', *, *, #7447, .T. ) ;
#12975=CARTESIAN_POINT ( 'NONE',  ( -23.33121169713865584, -23.95054477929251036, -17.32050807568878170 ) ) ;
#12977=FACE_BOUND ( 'NONE', #3742, .T. ) ;
#12978=CARTESIAN_POINT ( 'NONE',  ( -24.11451099155181055, -19.01228170252437977, 8.660254037844417496 ) ) ;
#12979=AXIS2_PLACEMENT_3D ( 'NONE', #16144, #3057, #3137 ) ;
#12981=AXIS2_PLACEMENT_3D ( 'NONE', #11445, #8634, #2841 ) ;
#12982=DIRECTION ( 'NONE',  ( 0.000000000000000000, 0.000000000000000000, 1.000000000000000000 ) ) ;
#12983=EDGE_LOOP ( 'NONE', ( #16768, #8182 ) ) ;
#12984=AXIS2_PLACEMENT_3D ( 'NONE', #15518, #16967, #1228 ) ;
#12985=EDGE_CURVE ( 'NONE', #18075, #6856, #14252, .T. ) ;
#12986=VERTEX_POINT ( 'NONE', #10239 ) ;
#12987=FACE_OUTER_BOUND ( 'NONE', #17059, .T. ) ;
#12988=CIRCLE ( 'NONE', #10808, 1.500000000000000888 ) ;
#12989=VECTOR ( 'NONE', #1109, 1000.000000000000000 ) ;
#12991=DIRECTION ( 'NONE',  ( -0.1566598588826321192, 0.9876526153536342445, 7.798540720466730171E-17 ) ) ;
#12993=CARTESIAN_POINT ( 'NONE',  ( -64.31879523431432233, -30.45192892292171294, 8.660254037844417496 ) ) ;
#12995=ADVANCED_FACE ( 'NONE', ( #8833 ), #9869, .F. ) ;
#12996=ADVANCED_FACE ( 'NONE', ( #8563 ), #1908, .F. ) ;
#12997=EDGE_LOOP ( 'NONE', ( #7366, #13299, #11194, #1022 ) ) ;
#12998=VECTOR ( 'NONE', #7163, 1000.000000000000000 ) ;
#12999=ORIENTED_EDGE ( 'NONE', *, *, #13245, .T. ) ;
#13000=DIRECTION ( 'NONE',  ( 0.000000000000000000, 0.000000000000000000, 1.000000000000000000 ) ) ;
#13001=ORIENTED_EDGE ( 'NONE', *, *, #7255, .F. ) ;
#13002=AXIS2_PLACEMENT_3D ( 'NONE', #4580, #2015, #7434 ) ;
#13003=LINE ( 'NONE', #5992, #13661 ) ;
#13004=CARTESIAN_POINT ( 'NONE',  ( -68.76323200340563346, -31.15689828789355786, 4.330127018922217630 ) ) ;
#13005=AXIS2_PLACEMENT_3D ( 'NONE', #3256, #9159, #6421 ) ;
#13006=ORIENTED_EDGE ( 'NONE', *, *, #4968, .F. ) ;
#13009=DIRECTION ( 'NONE',  ( -0.1566598588826321747, 0.9876526153536343555, 0.000000000000000000 ) ) ;
#13011=DIRECTION ( 'NONE',  ( -0.9876526153536336894, -0.1566598588826350336, 0.000000000000000000 ) ) ;
#13012=CIRCLE ( 'NONE', #5780, 1.500000000000000000 ) ;
#13013=DIRECTION ( 'NONE',  ( -0.1566598588826321747, 0.9876526153536343555, 0.000000000000000000 ) ) ;
#13014=AXIS2_PLACEMENT_3D ( 'NONE', #3505, #7897, #10641 ) ;
#13015=ORIENTED_EDGE ( 'NONE', *, *, #4340, .F. ) ;
#13016=ORIENTED_EDGE ( 'NONE', *, *, #10173, .T. ) ;
#13017=FACE_BOUND ( 'NONE', #4939, .T. ) ;
#13018=CYLINDRICAL_SURFACE ( 'NONE', #14173, 1.500000000000001554 ) ;
#13019=ORIENTED_EDGE ( 'NONE', *, *, #13395, .F. ) ;
#13020=AXIS2_PLACEMENT_3D ( 'NONE', #7091, #1484, #13024 ) ;
#13022=CARTESIAN_POINT ( 'NONE',  ( -36.46016868347218320, -20.97052993855728076, 21.65063509461102242 ) ) ;
#13023=EDGE_CURVE ( 'NONE', #3313, #10907, #18356, .T. ) ;
#13024=DIRECTION ( 'NONE',  ( -0.9876526153536336894, -0.1566598588826349503, 0.000000000000000000 ) ) ;
#13025=EDGE_LOOP ( 'NONE', ( #510, #7558, #13825, #5782 ) ) ;
#13026=LINE ( 'NONE', #10276, #3056 ) ;
#13027=AXIS2_PLACEMENT_3D ( 'NONE', #15288, #7915, #4949 ) ;
#13028=EDGE_CURVE ( 'NONE', #4155, #14517, #446, .T. ) ;
#13029=AXIS2_PLACEMENT_3D ( 'NONE', #4785, #9059, #15021 ) ;
#13030=DIRECTION ( 'NONE',  ( -0.1566598588826321192, 0.9876526153536342445, 7.798540720466731404E-17 ) ) ;
#13032=DIRECTION ( 'NONE',  ( 0.000000000000000000, 0.000000000000000000, 1.000000000000000000 ) ) ;
#13034=ORIENTED_EDGE ( 'NONE', *, *, #3694, .F. ) ;
#13035=CYLINDRICAL_SURFACE ( 'NONE', #14203, 1.500000000000001554 ) ;
#13037=VECTOR ( 'NONE', #14352, 1000.000000000000000 ) ;
#13038=CARTESIAN_POINT ( 'NONE',  ( -40.57549745564935506, -84.39127374608668219, -17.32050807568878525 ) ) ;
#13039=EDGE_LOOP ( 'NONE', ( #10625, #18661, #3643, #13831 ) ) ;
#13040=DIRECTION ( 'NONE',  ( 0.000000000000000000, 0.000000000000000000, 1.000000000000000000 ) ) ;
#13041=FACE_OUTER_BOUND ( 'NONE', #2345, .T. ) ;
#13042=VERTEX_POINT ( 'NONE', #6091 ) ;
#13043=AXIS2_PLACEMENT_3D ( 'NONE', #7994, #18370, #801 ) ;
#13045=DIRECTION ( 'NONE',  ( -0.1566598588826321470, 0.9876526153536342445, 4.523475108491707377E-17 ) ) ;
#13046=EDGE_LOOP ( 'NONE', ( #11737, #140, #461, #18350 ) ) ;
#13048=AXIS2_PLACEMENT_3D ( 'NONE', #10814, #3246, #16357 ) ;
#13049=EDGE_LOOP ( 'NONE', ( #5696, #18328 ) ) ;
#13050=EDGE_CURVE ( 'NONE', #17941, #4280, #1814, .T. ) ;
#13052=CIRCLE ( 'NONE', #15487, 1.499999999999999556 ) ;
#13055=CARTESIAN_POINT ( 'NONE',  ( -26.74836084069850983, -82.19803572172985184, 4.330127018922213189 ) ) ;
#13057=ADVANCED_FACE ( 'NONE', ( #587 ), #10619, .F. ) ;
#13058=CARTESIAN_POINT ( 'NONE',  ( -17.40529600501687923, -23.01058562599671831, -12.99038105676658006 ) ) ;
#13060=CARTESIAN_POINT ( 'NONE',  ( -68.76323200340563346, -31.15689828789355786, -12.99038105676658006 ) ) ;
#13061=ORIENTED_EDGE ( 'NONE', *, *, #4294, .F. ) ;
#13063=AXIS2_PLACEMENT_3D ( 'NONE', #8479, #1460, #8745 ) ;
#13064=CARTESIAN_POINT ( 'NONE',  ( -1.109027851681973598, -20.42569795443330349, -21.65063509461098334 ) ) ;
#13067=DIRECTION ( 'NONE',  ( -0.9876526153536341335, -0.1566598588826327021, 0.000000000000000000 ) ) ;
#13068=EDGE_LOOP ( 'NONE', ( #16658, #17769 ) ) ;
#13069=STYLED_ITEM ( 'NONE', ( #9285 ), #2591 ) ;
#13070=VERTEX_POINT ( 'NONE', #7502 ) ;
#13071=VERTEX_POINT ( 'NONE', #16135 ) ;
#13072=DIRECTION ( 'NONE',  ( -0.1566598588826321192, 0.9876526153536342445, 7.798540720466730171E-17 ) ) ;
#13073=ORIENTED_EDGE ( 'NONE', *, *, #957, .T. ) ;
#13074=ORIENTED_EDGE ( 'NONE', *, *, #11854, .F. ) ;
#13075=VERTEX_POINT ( 'NONE', #16313 ) ;
#13076=DIRECTION ( 'NONE',  ( -0.1566598588826321192, 0.9876526153536342445, 7.798540720466730171E-17 ) ) ;
#13077=AXIS2_PLACEMENT_3D ( 'NONE', #2834, #7390, #1425 ) ;
#13078=ORIENTED_EDGE ( 'NONE', *, *, #11613, .F. ) ;
#13079=ORIENTED_EDGE ( 'NONE', *, *, #1759, .T. ) ;
#13080=CARTESIAN_POINT ( 'NONE',  ( -21.64537945316773460, -18.62063205531779886, 12.99038105676661736 ) ) ;
#13081=ORIENTED_EDGE ( 'NONE', *, *, #704, .F. ) ;
#13085=EDGE_CURVE ( 'NONE', #13701, #3470, #7127, .T. ) ;
#13086=CYLINDRICAL_SURFACE ( 'NONE', #9041, 1.500000000000001554 ) ;
#13087=EDGE_LOOP ( 'NONE', ( #929, #6454, #16733, #17718 ) ) ;
#13088=VERTEX_POINT ( 'NONE', #17852 ) ;
#13090=DIRECTION ( 'NONE',  ( 0.000000000000000000, 0.000000000000000000, 1.000000000000000000 ) ) ;
#13091=CARTESIAN_POINT ( 'NONE',  ( -65.10209452872746283, -25.51366584615359301, 8.660254037844417496 ) ) ;
#13095=EDGE_LOOP ( 'NONE', ( #17045, #7116 ) ) ;
#13096=EDGE_LOOP ( 'NONE', ( #1057, #448 ) ) ;
#13097=DIRECTION ( 'NONE',  ( -0.1566598588826321747, 0.9876526153536343555, 0.000000000000000000 ) ) ;
#13098=EDGE_LOOP ( 'NONE', ( #5745, #16174 ) ) ;
#13100=DIRECTION ( 'NONE',  ( 1.000000000000000000, 0.000000000000000000, -2.995206001686573514E-16 ) ) ;
#13101=EDGE_CURVE ( 'NONE', #8447, #403, #13540, .T. ) ;
#13102=VERTEX_POINT ( 'NONE', #16422 ) ;
#13103=CIRCLE ( 'NONE', #14630, 1.500000000000000888 ) ;
#13104=DIRECTION ( 'NONE',  ( -0.1566598588826321747, 0.9876526153536343555, 0.000000000000000000 ) ) ;
#13106=CARTESIAN_POINT ( 'NONE',  ( 2.881217619910392269, -77.49823995525089515, -21.65063509461098690 ) ) ;
#13108=ORIENTED_EDGE ( 'NONE', *, *, #16861, .T. ) ;
#13110=AXIS2_PLACEMENT_3D ( 'NONE', #9174, #365, #6052 ) ;
#13113=ORIENTED_EDGE ( 'NONE', *, *, #1759, .F. ) ;
#13114=CYLINDRICAL_SURFACE ( 'NONE', #13230, 1.500000000000001554 ) ;
#13115=EDGE_LOOP ( 'NONE', ( #14930, #5153, #2974, #16124 ) ) ;
#13116=ORIENTED_EDGE ( 'NONE', *, *, #9023, .F. ) ;
#13117=CARTESIAN_POINT ( 'NONE',  ( -21.64537945316773460, -18.62063205531779886, 4.330127018922218518 ) ) ;
#13118=ORIENTED_EDGE ( 'NONE', *, *, #4367, .T. ) ;
#13120=CARTESIAN_POINT ( 'NONE',  ( -6.830590222863280658, -16.27073417207831696, -4.330127018922183879 ) ) ;
#13121=CARTESIAN_POINT ( 'NONE',  ( -39.13365354279673625, -26.45710252141460828, -12.99038105676658006 ) ) ;
#13123=EDGE_CURVE ( 'NONE', #12715, #7418, #17722, .T. ) ;
#13124=EDGE_CURVE ( 'NONE', #13600, #14719, #4922, .T. ) ;
#13125=CARTESIAN_POINT ( 'NONE',  ( -20.65772683781411345, -18.46397219643516507, 8.660254037844417496 ) ) ;
#13126=DIRECTION ( 'NONE',  ( 0.000000000000000000, 0.000000000000000000, 1.000000000000000000 ) ) ;
#13128=CARTESIAN_POINT ( 'NONE',  ( -58.84707083969148300, -87.28948113541535747, -17.32050807568878525 ) ) ;
#13129=DIRECTION ( 'NONE',  ( -0.9876526153536336894, -0.1566598588826350336, 0.000000000000000000 ) ) ;
#13130=ORIENTED_EDGE ( 'NONE', *, *, #8322, .T. ) ;
#13133=ORIENTED_EDGE ( 'NONE', *, *, #17118, .T. ) ;
#13135=DIRECTION ( 'NONE',  ( -0.9876526153536336894, -0.1566598588826349503, 0.000000000000000000 ) ) ;
#13136=ORIENTED_EDGE ( 'NONE', *, *, #5236, .F. ) ;
#13137=ORIENTED_EDGE ( 'NONE', *, *, #12447, .F. ) ;
#13138=CARTESIAN_POINT ( 'NONE',  ( -13.25033222266188915, -17.28902325481542235, -4.330127018922180326 ) ) ;
#13139=CARTESIAN_POINT ( 'NONE',  ( -45.55339554259534651, -27.47539160415172432, -21.65063509461098334 ) ) ;
#13140=DIRECTION ( 'NONE',  ( -0.9876526153536341335, -0.1566598588826327021, 0.000000000000000000 ) ) ;
#13141=DIRECTION ( 'NONE',  ( -0.9876526153536336894, -0.1566598588826350336, 0.000000000000000000 ) ) ;
#13142=DIRECTION ( 'NONE',  ( -1.000000000000000000, 0.000000000000000000, 0.000000000000000000 ) ) ;
#13143=DIRECTION ( 'NONE',  ( -0.1566598588826321192, 0.9876526153536342445, 7.798540720466730171E-17 ) ) ;
#13144=ORIENTED_EDGE ( 'NONE', *, *, #4744, .F. ) ;
#13145=LINE ( 'NONE', #178, #11362 ) ;
#13146=FACE_BOUND ( 'NONE', #4559, .T. ) ;
#13147=CARTESIAN_POINT ( 'NONE',  ( 3.231158466157551423, 19.73726462726227737, 30.00000000000000000 ) ) ;
#13149=EDGE_CURVE ( 'NONE', #10517, #5280, #15880, .T. ) ;
#13150=AXIS2_PLACEMENT_3D ( 'NONE', #8053, #12760, #18142 ) ;
#13151=VERTEX_POINT ( 'NONE', #4560 ) ;
#13152=EDGE_LOOP ( 'NONE', ( #18788, #10787, #4919, #12006 ) ) ;
#13153=EDGE_LOOP ( 'NONE', ( #14302, #10980, #14648, #17100 ) ) ;
#13154=CARTESIAN_POINT ( 'NONE',  ( -25.80034323552273179, -24.34219442649909126, -4.330127018922181215 ) ) ;
#13155=VERTEX_POINT ( 'NONE', #13261 ) ;
#13156=EDGE_CURVE ( 'NONE', #15511, #11621, #8003, .T. ) ;
#13157=ORIENTED_EDGE ( 'NONE', *, *, #11679, .T. ) ;
#13158=ORIENTED_EDGE ( 'NONE', *, *, #17291, .T. ) ;
#13160=EDGE_CURVE ( 'NONE', #10405, #6575, #11016, .T. ) ;
#13161=CYLINDRICAL_SURFACE ( 'NONE', #6128, 1.500000000000001554 ) ;
#13162=ORIENTED_EDGE ( 'NONE', *, *, #17168, .F. ) ;
#13165=DIRECTION ( 'NONE',  ( -0.1566598588826321747, 0.9876526153536343555, 0.000000000000000000 ) ) ;
#13166=ORIENTED_EDGE ( 'NONE', *, *, #8662, .T. ) ;
#13167=ORIENTED_EDGE ( 'NONE', *, *, #11115, .T. ) ;
#13169=CARTESIAN_POINT ( 'NONE',  ( -65.30644784966793281, -30.60858878180435738, 12.99038105676661736 ) ) ;
#13171=FACE_BOUND ( 'NONE', #5516, .T. ) ;
#13172=DIRECTION ( 'NONE',  ( -0.9876526153536341335, -0.1566598588826327021, 0.000000000000000000 ) ) ;
#13173=CIRCLE ( 'NONE', #4990, 1.499999999999999556 ) ;
#13174=VERTEX_POINT ( 'NONE', #3684 ) ;
#13175=EDGE_CURVE ( 'NONE', #13731, #5249, #14664, .T. ) ;
#13176=ORIENTED_EDGE ( 'NONE', *, *, #5661, .F. ) ;
#13177=ORIENTED_EDGE ( 'NONE', *, *, #16228, .F. ) ;
#13178=FACE_OUTER_BOUND ( 'NONE', #16375, .T. ) ;
#13180=VERTEX_POINT ( 'NONE', #6470 ) ;
#13181=FACE_BOUND ( 'NONE', #6200, .T. ) ;
#13183=EDGE_LOOP ( 'NONE', ( #8058, #5391, #12197, #16179 ) ) ;
#13184=DIRECTION ( 'NONE',  ( -0.1566598588826321747, 0.9876526153536343555, 0.000000000000000000 ) ) ;
#13187=ORIENTED_EDGE ( 'NONE', *, *, #10826, .T. ) ;
#13193=EDGE_CURVE ( 'NONE', #18229, #14892, #18029, .T. ) ;
#13194=EDGE_LOOP ( 'NONE', ( #2520, #5320 ) ) ;
#13195=ORIENTED_EDGE ( 'NONE', *, *, #13835, .F. ) ;
#13196=FACE_BOUND ( 'NONE', #9116, .T. ) ;
#13197=CYLINDRICAL_SURFACE ( 'NONE', #4477, 1.500000000000001554 ) ;
#13198=EDGE_CURVE ( 'NONE', #11470, #15920, #1231, .T. ) ;
#13200=CARTESIAN_POINT ( 'NONE',  ( -57.20087360589840131, -24.26038697509254760, 17.32050807568881723 ) ) ;
#13201=DIRECTION ( 'NONE',  ( -0.9876526153536341335, -0.1566598588826327021, 0.000000000000000000 ) ) ;
#13202=ORIENTED_EDGE ( 'NONE', *, *, #3770, .T. ) ;
#13203=CIRCLE ( 'NONE', #2620, 1.500000000000000000 ) ;
#13204=ORIENTED_EDGE ( 'NONE', *, *, #463, .F. ) ;
#13206=DIRECTION ( 'NONE',  ( 0.000000000000000000, 0.000000000000000000, 1.000000000000000000 ) ) ;
#13208=CARTESIAN_POINT ( 'NONE',  ( -26.58364252993588650, -19.40393134973096068, 21.65063509461102242 ) ) ;
#13211=DIRECTION ( 'NONE',  ( -0.1566598588826321192, 0.9876526153536342445, 7.798540720466730171E-17 ) ) ;
#13212=DIRECTION ( 'NONE',  ( -0.1566598588826321747, 0.9876526153536343555, 0.000000000000000000 ) ) ;
#13214=DIRECTION ( 'NONE',  ( -0.1566598588826321192, 0.9876526153536342445, 7.798540720466730171E-17 ) ) ;
#13215=VECTOR ( 'NONE', #13797, 1000.000000000000000 ) ;
#13218=ORIENTED_EDGE ( 'NONE', *, *, #15365, .T. ) ;
#13221=ORIENTED_EDGE ( 'NONE', *, *, #13050, .F. ) ;
#13222=ORIENTED_EDGE ( 'NONE', *, *, #15913, .F. ) ;
#13223=VECTOR ( 'NONE', #11591, 1000.000000000000000 ) ;
#13224=VERTEX_POINT ( 'NONE', #12205 ) ;
#13225=EDGE_CURVE ( 'NONE', #13042, #2286, #18662, .T. ) ;
#13226=ORIENTED_EDGE ( 'NONE', *, *, #22, .T. ) ;
#13230=AXIS2_PLACEMENT_3D ( 'NONE', #5925, #4491, #7174 ) ;
#13231=CARTESIAN_POINT ( 'NONE',  ( -8.312069145893737243, -16.50572396040226053, 12.99038105676661026 ) ) ;
#13232=CARTESIAN_POINT ( 'NONE',  ( -73.70149508017375695, -31.94019758230671258, -21.65063509461098334 ) ) ;
#13233=DIRECTION ( 'NONE',  ( -0.1566598588826321192, 0.9876526153536342445, 7.798540720466730171E-17 ) ) ;
#13235=DIRECTION ( 'NONE',  ( -0.1566598588826321747, 0.9876526153536343555, 0.000000000000000000 ) ) ;
#13236=CARTESIAN_POINT ( 'NONE',  ( -63.78533391645962780, -88.07278042982852639, -8.660254037844385522 ) ) ;
#13237=DIRECTION ( 'NONE',  ( -0.1566598588826321747, 0.9876526153536343555, 0.000000000000000000 ) ) ;
#13238=DIRECTION ( 'NONE',  ( -0.1566598588826321747, 0.9876526153536343555, 0.000000000000000000 ) ) ;
#13240=ORIENTED_EDGE ( 'NONE', *, *, #51, .F. ) ;
#13241=VECTOR ( 'NONE', #2835, 1000.000000000000000 ) ;
#13242=EDGE_LOOP ( 'NONE', ( #17658, #5222, #13801, #12277 ) ) ;
#13244=ORIENTED_EDGE ( 'NONE', *, *, #6879, .T. ) ;
#13245=EDGE_CURVE ( 'NONE', #9271, #17419, #15264, .T. ) ;
#13246=VERTEX_POINT ( 'NONE', #18255 ) ;
#13247=DIRECTION ( 'NONE',  ( -0.9876526153536341335, -0.1566598588826327576, 0.000000000000000000 ) ) ;
#13248=CIRCLE ( 'NONE', #12028, 1.500000000000000888 ) ;
#13249=DIRECTION ( 'NONE',  ( -0.1566598588826321747, 0.9876526153536343555, 0.000000000000000000 ) ) ;
#13250=AXIS2_PLACEMENT_3D ( 'NONE', #3623, #13762, #8199 ) ;
#13251=EDGE_CURVE ( 'NONE', #983, #3927, #8517, .T. ) ;
#13252=CARTESIAN_POINT ( 'NONE',  ( -9.464440072009985272, -79.45648819128378193, -17.32050807568878525 ) ) ;
#13254=AXIS2_PLACEMENT_3D ( 'NONE', #17927, #12179, #13505 ) ;
#13255=CARTESIAN_POINT ( 'NONE',  ( -35.14340807120434818, -83.52964452223221770, 12.99038105676661203 ) ) ;
#13256=ORIENTED_EDGE ( 'NONE', *, *, #18250, .F. ) ;
#13257=FACE_BOUND ( 'NONE', #4865, .T. ) ;
#13258=AXIS2_PLACEMENT_3D ( 'NONE', #2490, #12423, #18266 ) ;
#13260=ORIENTED_EDGE ( 'NONE', *, *, #3328, .T. ) ;
#13261=CARTESIAN_POINT ( 'NONE',  ( -76.95392591297100182, -27.39358415274517000, -8.660254037844380193 ) ) ;
#13263=AXIS2_PLACEMENT_3D ( 'NONE', #17728, #14763, #8801 ) ;
#13264=CARTESIAN_POINT ( 'NONE',  ( -7.982961148979534016, -79.22149840295983836, -8.660254037844385522 ) ) ;
#13265=CIRCLE ( 'NONE', #14492, 1.500000000000000888 ) ;
#13266=VERTEX_POINT ( 'NONE', #3584 ) ;
#13267=ORIENTED_EDGE ( 'NONE', *, *, #3347, .F. ) ;
#13268=ORIENTED_EDGE ( 'NONE', *, *, #10970, .F. ) ;
#13269=EDGE_LOOP ( 'NONE', ( #9647, #15374, #13226, #4881 ) ) ;
#13270=CARTESIAN_POINT ( 'NONE',  ( 10.28861223506262412, -76.32329101363113466, 8.660254037844406838 ) ) ;
#13272=FACE_BOUND ( 'NONE', #2804, .T. ) ;
#13273=CIRCLE ( 'NONE', #14214, 1.500000000000000888 ) ;
#13274=CARTESIAN_POINT ( 'NONE',  ( -52.96079015774756726, -28.65034054577146705, -8.660254037844380193 ) ) ;
#13275=ORIENTED_EDGE ( 'NONE', *, *, #18576, .T. ) ;
#13276=EDGE_CURVE ( 'NONE', #6476, #11377, #10722, .T. ) ;
#13277=LINE ( 'NONE', #17867, #11853 ) ;
#13278=AXIS2_PLACEMENT_3D ( 'NONE', #10128, #6842, #18542 ) ;
#13280=AXIS2_PLACEMENT_3D ( 'NONE', #8954, #13212, #12848 ) ;
#13281=CIRCLE ( 'NONE', #1752, 1.500000000000000444 ) ;
#13282=AXIS2_PLACEMENT_3D ( 'NONE', #18046, #6752, #18636 ) ;
#13283=AXIS2_PLACEMENT_3D ( 'NONE', #13308, #342, #3251 ) ;
#13285=EDGE_CURVE ( 'NONE', #2423, #3127, #9825, .T. ) ;
#13286=DIRECTION ( 'NONE',  ( -0.1566598588826321192, 0.9876526153536342445, 7.798540720466730171E-17 ) ) ;
#13287=DIRECTION ( 'NONE',  ( -0.9876526153536341335, -0.1566598588826327021, 0.000000000000000000 ) ) ;
#13288=CARTESIAN_POINT ( 'NONE',  ( -31.52190560670403841, -20.18723064414411894, 12.99038105676661736 ) ) ;
#13289=DIRECTION ( 'NONE',  ( -0.1566598588826321192, 0.9876526153536342445, 7.798540720466730171E-17 ) ) ;
#13290=AXIS2_PLACEMENT_3D ( 'NONE', #6435, #18008, #4967 ) ;
#13291=LINE ( 'NONE', #10543, #16570 ) ;
#13292=VERTEX_POINT ( 'NONE', #9391 ) ;
#13293=VERTEX_POINT ( 'NONE', #15169 ) ;
#13294=FACE_BOUND ( 'NONE', #9800, .T. ) ;
#13295=DIRECTION ( 'NONE',  ( -0.000000000000000000, -0.000000000000000000, -1.000000000000000000 ) ) ;
#13296=CIRCLE ( 'NONE', #5129, 1.499999999999999556 ) ;
#13297=CARTESIAN_POINT ( 'NONE',  ( 0.5768043922889515285, -15.09578523045857601, -17.32050807568878170 ) ) ;
#13298=DIRECTION ( 'NONE',  ( -0.1566598588826321192, 0.9876526153536342445, 7.798540720466731404E-17 ) ) ;
#13299=ORIENTED_EDGE ( 'NONE', *, *, #15821, .F. ) ;
#13301=AXIS2_PLACEMENT_3D ( 'NONE', #1987, #12004, #7773 ) ;
#13302=ORIENTED_EDGE ( 'NONE', *, *, #4285, .F. ) ;
#13303=CYLINDRICAL_SURFACE ( 'NONE', #5186, 1.500000000000001554 ) ;
#13304=AXIS2_PLACEMENT_3D ( 'NONE', #12772, #11332, #1413 ) ;
#13305=EDGE_CURVE ( 'NONE', #5271, #17224, #11625, .T. ) ;
#13306=CARTESIAN_POINT ( 'NONE',  ( -73.49714175923330117, -26.84527464665596241, 8.660254037844417496 ) ) ;
#13307=EDGE_CURVE ( 'NONE', #2732, #14342, #14060, .T. ) ;
#13308=CARTESIAN_POINT ( 'NONE',  ( -16.70711637639958269, -17.83733276090463349, -21.65063509461097979 ) ) ;
#13310=EDGE_CURVE ( 'NONE', #13701, #8275, #1323, .T. ) ;
#13311=ORIENTED_EDGE ( 'NONE', *, *, #13101, .F. ) ;
#13312=AXIS2_PLACEMENT_3D ( 'NONE', #5135, #1087, #12702 ) ;
#13313=CARTESIAN_POINT ( 'NONE',  ( -0.9046745307415022808, -15.33077501878252136, 8.660254037844412167 ) ) ;
#13314=AXIS2_PLACEMENT_3D ( 'NONE', #10742, #16660, #9532 ) ;
#13315=CARTESIAN_POINT ( 'NONE',  ( -2.000000000000000000, 0.000000000000000000, -30.00000000000000000 ) ) ;
#13316=DIRECTION ( 'NONE',  ( -0.9876526153536341335, -0.1566598588826327021, 0.000000000000000000 ) ) ;
#13317=DIRECTION ( 'NONE',  ( -0.1566598588826321192, 0.9876526153536342445, 7.798540720466730171E-17 ) ) ;
#13319=DIRECTION ( 'NONE',  ( 0.000000000000000000, 0.000000000000000000, 1.000000000000000000 ) ) ;
#13320=ORIENTED_EDGE ( 'NONE', *, *, #9097, .F. ) ;
#13321=AXIS2_PLACEMENT_3D ( 'NONE', #5281, #13693, #10949 ) ;
#13322=AXIS2_PLACEMENT_3D ( 'NONE', #2041, #4688, #2140 ) ;
#13323=ORIENTED_EDGE ( 'NONE', *, *, #1970, .F. ) ;
#13324=ORIENTED_EDGE ( 'NONE', *, *, #12501, .F. ) ;
#13325=CIRCLE ( 'NONE', #1257, 1.500000000000001332 ) ;
#13326=DIRECTION ( 'NONE',  ( 0.000000000000000000, 0.000000000000000000, 1.000000000000000000 ) ) ;
#13327=AXIS2_PLACEMENT_3D ( 'NONE', #4110, #2526, #8313 ) ;
#13328=EDGE_CURVE ( 'NONE', #15786, #16387, #2568, .T. ) ;
#13330=CYLINDRICAL_SURFACE ( 'NONE', #13110, 1.500000000000001554 ) ;
#13331=ORIENTED_EDGE ( 'NONE', *, *, #174, .T. ) ;
#13332=CYLINDRICAL_SURFACE ( 'NONE', #12421, 1.500000000000001554 ) ;
#13333=DIRECTION ( 'NONE',  ( -0.1566598588826321192, 0.9876526153536342445, 7.798540720466731404E-17 ) ) ;
#13335=ORIENTED_EDGE ( 'NONE', *, *, #15064, .F. ) ;
#13336=AXIS2_PLACEMENT_3D ( 'NONE', #1126, #7182, #15689 ) ;
#13337=EDGE_CURVE ( 'NONE', #8644, #9857, #1660, .T. ) ;
#13338=LINE ( 'NONE', #17363, #571 ) ;
#13339=ORIENTED_EDGE ( 'NONE', *, *, #9297, .T. ) ;
#13340=CIRCLE ( 'NONE', #8521, 1.500000000000000888 ) ;
#13341=CARTESIAN_POINT ( 'NONE',  ( -1.892327146095121204, -15.48743487766515337, -12.99038105676658361 ) ) ;
#13343=CARTESIAN_POINT ( 'NONE',  ( -81.73462711737164454, 33.01666666666666572, -35.00000000000000000 ) ) ;
#13344=EDGE_LOOP ( 'NONE', ( #10193, #13176 ) ) ;
#13346=LINE ( 'NONE', #561, #18184 ) ;
#13347=EDGE_LOOP ( 'NONE', ( #4508, #12814 ) ) ;
#13348=AXIS2_PLACEMENT_3D ( 'NONE', #3798, #18284, #2217 ) ;
#13349=EDGE_LOOP ( 'NONE', ( #17399, #3816 ) ) ;
#13350=CARTESIAN_POINT ( 'NONE',  ( -8.312069145893737243, -16.50572396040226053, -4.330127018922183879 ) ) ;
#13352=ORIENTED_EDGE ( 'NONE', *, *, #2238, .F. ) ;
#13353=AXIS2_PLACEMENT_3D ( 'NONE', #18624, #2832, #15715 ) ;
#13354=CYLINDRICAL_SURFACE ( 'NONE', #6577, 1.500000000000000888 ) ;
#13355=CARTESIAN_POINT ( 'NONE',  ( -54.73174206751431115, -23.86873732788597025, 21.65063509461101887 ) ) ;
#13356=VECTOR ( 'NONE', #8623, 1000.000000000000000 ) ;
#13357=CARTESIAN_POINT ( 'NONE',  ( -60.36818477289977380, -29.82528948739119556, 21.65063509461101887 ) ) ;
#13358=CARTESIAN_POINT ( 'NONE',  ( -70.24471092643608472, -31.39188807621751209, 12.99038105676661736 ) ) ;
#13359=DIRECTION ( 'NONE',  ( -0.1566598588826321192, 0.9876526153536342445, 7.798540720466730171E-17 ) ) ;
#13360=DIRECTION ( 'NONE',  ( -0.1566598588826321192, 0.9876526153536342445, 7.798540720466731404E-17 ) ) ;
#13361=ORIENTED_EDGE ( 'NONE', *, *, #3645, .F. ) ;
#13362=EDGE_CURVE ( 'NONE', #8019, #5828, #12845, .T. ) ;
#13363=VECTOR ( 'NONE', #15469, 1000.000000000000000 ) ;
#13364=EDGE_CURVE ( 'NONE', #931, #10329, #1593, .T. ) ;
#13366=ORIENTED_EDGE ( 'NONE', *, *, #12332, .F. ) ;
#13367=CARTESIAN_POINT ( 'NONE',  ( -34.15575545585073058, -83.37298466334958391, 17.32050807568881368 ) ) ;
#13368=CARTESIAN_POINT ( 'NONE',  ( -67.24211807019732134, -88.62108993591775175, 8.660254037844412167 ) ) ;
#13369=CIRCLE ( 'NONE', #13077, 1.500000000000000888 ) ;
#13370=ADVANCED_FACE ( 'NONE', ( #7192 ), #3085, .F. ) ;
#13371=ORIENTED_EDGE ( 'NONE', *, *, #10708, .F. ) ;
#13372=EDGE_LOOP ( 'NONE', ( #18539, #4701, #9636, #2019 ) ) ;
#13373=ORIENTED_EDGE ( 'NONE', *, *, #10660, .F. ) ;
#13374=ORIENTED_EDGE ( 'NONE', *, *, #7474, .T. ) ;
#13375=CYLINDRICAL_SURFACE ( 'NONE', #10462, 1.500000000000001554 ) ;
#13376=ORIENTED_EDGE ( 'NONE', *, *, #10351, .T. ) ;
#13377=FACE_BOUND ( 'NONE', #14794, .T. ) ;
#13378=VECTOR ( 'NONE', #5982, 1000.000000000000000 ) ;
#13379=FACE_OUTER_BOUND ( 'NONE', #17048, .T. ) ;
#13380=ORIENTED_EDGE ( 'NONE', *, *, #7889, .F. ) ;
#13382=ORIENTED_EDGE ( 'NONE', *, *, #7970, .F. ) ;
#13383=CYLINDRICAL_SURFACE ( 'NONE', #10883, 1.500000000000001554 ) ;
#13384=DIRECTION ( 'NONE',  ( -0.9876526153536341335, -0.1566598588826327576, 0.000000000000000000 ) ) ;
#13385=FACE_OUTER_BOUND ( 'NONE', #8860, .T. ) ;
#13386=DIRECTION ( 'NONE',  ( -0.1566598588826321747, 0.9876526153536343555, 0.000000000000000000 ) ) ;
#13387=ORIENTED_EDGE ( 'NONE', *, *, #2552, .T. ) ;
#13388=ORIENTED_EDGE ( 'NONE', *, *, #17570, .T. ) ;
#13389=CYLINDRICAL_SURFACE ( 'NONE', #14776, 1.500000000000001554 ) ;
#13390=ADVANCED_FACE ( 'NONE', ( #14383 ), #17716, .F. ) ;
#13392=CIRCLE ( 'NONE', #16448, 1.499999999999999556 ) ;
#13393=EDGE_LOOP ( 'NONE', ( #5036, #8011 ) ) ;
#13394=DIRECTION ( 'NONE',  ( -0.1566598588826321747, 0.9876526153536343555, 0.000000000000000000 ) ) ;
#13395=EDGE_CURVE ( 'NONE', #2096, #3287, #2892, .T. ) ;
#13397=CARTESIAN_POINT ( 'NONE',  ( -24.11451099155181055, -19.01228170252437621, 1.908195823574487804E-14 ) ) ;
#13399=AXIS2_PLACEMENT_3D ( 'NONE', #4614, #17818, #11887 ) ;
#13403=CARTESIAN_POINT ( 'NONE',  ( -49.79347899074618056, -23.08543803347280488, 4.330127018922218518 ) ) ;
#13405=ORIENTED_EDGE ( 'NONE', *, *, #14726, .T. ) ;
#13407=ORIENTED_EDGE ( 'NONE', *, *, #12728, .F. ) ;
#13408=EDGE_CURVE ( 'NONE', #10248, #11883, #1969, .T. ) ;
#13410=VERTEX_POINT ( 'NONE', #2819 ) ;
#13411=EDGE_CURVE ( 'NONE', #9589, #11831, #9850, .T. ) ;
#13413=DIRECTION ( 'NONE',  ( -0.9876526153536341335, -0.1566598588826327021, 0.000000000000000000 ) ) ;
#13414=CARTESIAN_POINT ( 'NONE',  ( -52.92115514756970640, -86.34952198211959740, 21.65063509461101532 ) ) ;
#13415=DIRECTION ( 'NONE',  ( 0.000000000000000000, 0.000000000000000000, 1.000000000000000000 ) ) ;
#13416=CARTESIAN_POINT ( 'NONE',  ( -62.63296299034339398, -25.12201619894700144, -21.65063509461098334 ) ) ;
#13417=DIRECTION ( 'NONE',  ( -0.1566598588826321747, 0.9876526153536343555, 0.000000000000000000 ) ) ;
#13420=DIRECTION ( 'NONE',  ( -0.9876526153536336894, -0.1566598588826349503, 0.000000000000000000 ) ) ;
#13421=DIRECTION ( 'NONE',  ( -0.9876526153536336894, -0.1566598588826349503, 0.000000000000000000 ) ) ;
#13422=ORIENTED_EDGE ( 'NONE', *, *, #8473, .F. ) ;
#13423=DIRECTION ( 'NONE',  ( 0.000000000000000000, 0.000000000000000000, 1.000000000000000000 ) ) ;
#13424=EDGE_CURVE ( 'NONE', #3317, #12090, #15895, .T. ) ;
#13425=CYLINDRICAL_SURFACE ( 'NONE', #3276, 1.500000000000001554 ) ;
#13426=VERTEX_POINT ( 'NONE', #14467 ) ;
#13427=EDGE_CURVE ( 'NONE', #14148, #1617, #1498, .T. ) ;
#13429=ADVANCED_FACE ( 'NONE', ( #17522 ), #10288, .F. ) ;
#13431=ORIENTED_EDGE ( 'NONE', *, *, #6857, .T. ) ;
#13432=CYLINDRICAL_SURFACE ( 'NONE', #5356, 1.500000000000001554 ) ;
#13433=LINE ( 'NONE', #14962, #5522 ) ;
#13435=FACE_OUTER_BOUND ( 'NONE', #13153, .T. ) ;
#13436=VERTEX_POINT ( 'NONE', #5859 ) ;
#13437=DIRECTION ( 'NONE',  ( 0.000000000000000000, 0.000000000000000000, 1.000000000000000000 ) ) ;
#13438=CYLINDRICAL_SURFACE ( 'NONE', #16714, 1.500000000000001554 ) ;
#13440=AXIS2_PLACEMENT_3D ( 'NONE', #13721, #5483, #5004 ) ;
#13442=DIRECTION ( 'NONE',  ( 0.000000000000000000, 0.000000000000000000, 1.000000000000000000 ) ) ;
#13443=ORIENTED_EDGE ( 'NONE', *, *, #12055, .T. ) ;
#13444=DIRECTION ( 'NONE',  ( -0.1566598588826321747, 0.9876526153536343555, 0.000000000000000000 ) ) ;
#13445=ORIENTED_EDGE ( 'NONE', *, *, #18250, .T. ) ;
#13447=DIRECTION ( 'NONE',  ( -0.1566598588826321192, 0.9876526153536342445, 7.798540720466731404E-17 ) ) ;
#13448=ORIENTED_EDGE ( 'NONE', *, *, #5885, .T. ) ;
#13449=EDGE_LOOP ( 'NONE', ( #12180, #12592, #7244, #11757 ) ) ;
#13450=ORIENTED_EDGE ( 'NONE', *, *, #1465, .F. ) ;
#13451=ORIENTED_EDGE ( 'NONE', *, *, #8242, .T. ) ;
#13452=CARTESIAN_POINT ( 'NONE',  ( -24.27922930231443743, -81.80638607452327449, 17.32050807568881368 ) ) ;
#13453=ORIENTED_EDGE ( 'NONE', *, *, #17570, .F. ) ;
#13454=VERTEX_POINT ( 'NONE', #11605 ) ;
#13455=CIRCLE ( 'NONE', #17433, 1.499999999999999556 ) ;
#13456=FACE_BOUND ( 'NONE', #13689, .T. ) ;
#13457=ADVANCED_FACE ( 'NONE', ( #349 ), #17427, .F. ) ;
#13459=DIRECTION ( 'NONE',  ( -0.9876526153536341335, -0.1566598588826327021, 0.000000000000000000 ) ) ;
#13460=VERTEX_POINT ( 'NONE', #8780 ) ;
#13461=EDGE_LOOP ( 'NONE', ( #15822, #5240 ) ) ;
#13462=DIRECTION ( 'NONE',  ( -0.1566598588826321747, 0.9876526153536343555, 0.000000000000000000 ) ) ;
#13463=FACE_BOUND ( 'NONE', #3094, .T. ) ;
#13464=CARTESIAN_POINT ( 'NONE',  ( -84.16561914167408531, -33.59999999999994458, 30.00000000000000000 ) ) ;
#13466=DIRECTION ( 'NONE',  ( -0.9876526153536344665, -0.1566598588826304539, 0.000000000000000000 ) ) ;
#13467=LINE ( 'NONE', #4937, #15906 ) ;
#13468=DIRECTION ( 'NONE',  ( -0.1566598588826321747, 0.9876526153536343555, 0.000000000000000000 ) ) ;
#13469=ORIENTED_EDGE ( 'NONE', *, *, #1172, .T. ) ;
#13470=ORIENTED_EDGE ( 'NONE', *, *, #18448, .T. ) ;
#13472=FACE_OUTER_BOUND ( 'NONE', #15564, .T. ) ;
#13474=EDGE_LOOP ( 'NONE', ( #164, #1861 ) ) ;
#13475=CARTESIAN_POINT ( 'NONE',  ( -45.01993422474066620, -85.09624311105851291, -12.99038105676658539 ) ) ;
#13476=EDGE_LOOP ( 'NONE', ( #15666, #6469 ) ) ;
#13480=ORIENTED_EDGE ( 'NONE', *, *, #8911, .F. ) ;
#13483=EDGE_CURVE ( 'NONE', #12253, #15050, #767, .T. ) ;
#13484=DIRECTION ( 'NONE',  ( -0.1566598588826321192, 0.9876526153536342445, 7.798540720466730171E-17 ) ) ;
#13485=DIRECTION ( 'NONE',  ( -0.1566598588826321192, 0.9876526153536342445, 7.798540720466731404E-17 ) ) ;
#13486=EDGE_LOOP ( 'NONE', ( #7365, #13073 ) ) ;
#13487=ORIENTED_EDGE ( 'NONE', *, *, #16832, .F. ) ;
#13488=DIRECTION ( 'NONE',  ( -0.1566598588826321192, 0.9876526153536342445, 7.798540720466730171E-17 ) ) ;
#13489=CIRCLE ( 'NONE', #5019, 1.500000000000001332 ) ;
#13491=DIRECTION ( 'NONE',  ( -0.9876526153536341335, -0.1566598588826327021, 0.000000000000000000 ) ) ;
#13493=ORIENTED_EDGE ( 'NONE', *, *, #7664, .T. ) ;
#13495=AXIS2_PLACEMENT_3D ( 'NONE', #11545, #2926, #4163 ) ;
#13496=DIRECTION ( 'NONE',  ( -0.9876526153536336894, -0.1566598588826349503, 0.000000000000000000 ) ) ;
#13497=CARTESIAN_POINT ( 'NONE',  ( -61.35583738825340561, -29.98194934627382224, -8.660254037844380193 ) ) ;
#13498=ORIENTED_EDGE ( 'NONE', *, *, #16533, .F. ) ;
#13499=DIRECTION ( 'NONE',  ( -0.1566598588826321192, 0.9876526153536342445, 7.798540720466730171E-17 ) ) ;
#13500=CARTESIAN_POINT ( 'NONE',  ( -81.73462711737164454, 33.01666666666666572, 30.00000000000000000 ) ) ;
#13501=EDGE_CURVE ( 'NONE', #8368, #17125, #11511, .T. ) ;
#13502=DIRECTION ( 'NONE',  ( -0.9876526153536341335, -0.1566598588826327021, 0.000000000000000000 ) ) ;
#13504=CARTESIAN_POINT ( 'NONE',  ( -29.75095369693726255, -24.96883386202961574, -17.32050807568878170 ) ) ;
#13505=DIRECTION ( 'NONE',  ( -0.9876526153536344665, -0.1566598588826304539, 0.000000000000000000 ) ) ;
#13506=AXIS2_PLACEMENT_3D ( 'NONE', #11053, #956, #1974 ) ;
#13508=CARTESIAN_POINT ( 'NONE',  ( -26.58364252993588650, -19.40393134973095712, 4.330127018922218518 ) ) ;
#13509=CARTESIAN_POINT ( 'NONE',  ( -3.373806069125576901, -15.72242466598909871, 12.99038105676661026 ) ) ;
#13511=EDGE_CURVE ( 'NONE', #17176, #6871, #6597, .T. ) ;
#13512=CYLINDRICAL_SURFACE ( 'NONE', #553, 1.500000000000001554 ) ;
#13513=CARTESIAN_POINT ( 'NONE',  ( -20.86208015875458344, -23.55889513208593655, -4.330127018922181215 ) ) ;
#13514=FACE_OUTER_BOUND ( 'NONE', #5434, .T. ) ;
#13515=ORIENTED_EDGE ( 'NONE', *, *, #128, .F. ) ;
#13516=DIRECTION ( 'NONE',  ( -0.9876526153536341335, -0.1566598588826327021, 0.000000000000000000 ) ) ;
#13518=VERTEX_POINT ( 'NONE', #3258 ) ;
#13519=AXIS2_PLACEMENT_3D ( 'NONE', #1746, #13298, #17789 ) ;
#13522=EDGE_CURVE ( 'NONE', #10673, #14246, #7732, .T. ) ;
#13524=AXIS2_PLACEMENT_3D ( 'NONE', #3840, #8325, #18517 ) ;
#13526=DIRECTION ( 'NONE',  ( 0.000000000000000000, 0.000000000000000000, 1.000000000000000000 ) ) ;
#13527=EDGE_LOOP ( 'NONE', ( #2679, #6796, #539, #415 ) ) ;
#13528=CARTESIAN_POINT ( 'NONE',  ( -79.91688375903190433, -27.86356372939307136, 17.32050807568881723 ) ) ;
#13529=ADVANCED_FACE ( 'NONE', ( #818 ), #5172, .F. ) ;
#13530=ADVANCED_FACE ( 'NONE', ( #13589 ), #3441, .F. ) ;
#13531=CARTESIAN_POINT ( 'NONE',  ( -67.77557938805200877, -31.00023842901093118, 1.869203119972154228E-14 ) ) ;
#13532=DIRECTION ( 'NONE',  ( -0.9876526153536341335, -0.1566598588826327021, 0.000000000000000000 ) ) ;
#13533=DIRECTION ( 'NONE',  ( -0.9876526153536341335, -0.1566598588826330907, 0.000000000000000000 ) ) ;
#13534=EDGE_LOOP ( 'NONE', ( #4838, #12224 ) ) ;
#13535=FACE_BOUND ( 'NONE', #15381, .T. ) ;
#13538=FILL_AREA_STYLE ('',( #15251 ) ) ;
#13539=EDGE_LOOP ( 'NONE', ( #4528, #4751, #18679, #5574 ) ) ;
#13540=LINE ( 'NONE', #12010, #4053 ) ;
#13541=DIRECTION ( 'NONE',  ( 0.000000000000000000, 0.000000000000000000, 1.000000000000000000 ) ) ;
#13542=VECTOR ( 'NONE', #12559, 1000.000000000000000 ) ;
#13543=ORIENTED_EDGE ( 'NONE', *, *, #131, .F. ) ;
#13544=ORIENTED_EDGE ( 'NONE', *, *, #17175, .F. ) ;
#13545=ORIENTED_EDGE ( 'NONE', *, *, #12119, .T. ) ;
#13546=DIRECTION ( 'NONE',  ( -0.1566598588826321192, 0.9876526153536342445, 7.798540720466730171E-17 ) ) ;
#13548=ORIENTED_EDGE ( 'NONE', *, *, #16091, .F. ) ;
#13549=FACE_BOUND ( 'NONE', #2042, .T. ) ;
#13551=DIRECTION ( 'NONE',  ( -0.1566598588826321192, 0.9876526153536342445, 7.798540720466730171E-17 ) ) ;
#13553=EDGE_CURVE ( 'NONE', #15511, #16506, #17908, .T. ) ;
#13555=ORIENTED_EDGE ( 'NONE', *, *, #7206, .F. ) ;
#13556=CIRCLE ( 'NONE', #251, 1.500000000000000888 ) ;
#13557=CIRCLE ( 'NONE', #12652, 1.500000000000000888 ) ;
#13558=CARTESIAN_POINT ( 'NONE',  ( -38.92930022185625205, -21.36217958576384746, -8.660254037844380193 ) ) ;
#13559=AXIS2_PLACEMENT_3D ( 'NONE', #5184, #646, #7936 ) ;
#13560=EDGE_LOOP ( 'NONE', ( #14729, #7143, #6203, #3888 ) ) ;
#13561=CARTESIAN_POINT ( 'NONE',  ( -1.109027851681966492, -20.42569795443330349, 12.99038105676661026 ) ) ;
#13562=EDGE_CURVE ( 'NONE', #2420, #15025, #16824, .T. ) ;
#13564=EDGE_CURVE ( 'NONE', #7429, #12177, #6226, .T. ) ;
#13565=DIRECTION ( 'NONE',  ( -0.1566598588826321192, 0.9876526153536342445, 7.798540720466731404E-17 ) ) ;
#13567=ORIENTED_EDGE ( 'NONE', *, *, #8014, .F. ) ;
#13568=VERTEX_POINT ( 'NONE', #10664 ) ;
#13569=CARTESIAN_POINT ( 'NONE',  ( -68.72359699322777260, -88.85607972424169532, 17.32050807568881368 ) ) ;
#13570=CARTESIAN_POINT ( 'NONE',  ( -45.51376053241748565, -85.17457304049985112, 1.424741226644455312E-14 ) ) ;
#13571=DIRECTION ( 'NONE',  ( -0.9876526153536336894, -0.1566598588826349503, 0.000000000000000000 ) ) ;
#13572=DIRECTION ( 'NONE',  ( -0.1566598588826321192, 0.9876526153536342445, 7.798540720466731404E-17 ) ) ;
#13573=AXIS2_PLACEMENT_3D ( 'NONE', #17951, #13165, #13532 ) ;
#13574=AXIS2_PLACEMENT_3D ( 'NONE', #7697, #200, #13541 ) ;
#13575=VERTEX_POINT ( 'NONE', #15018 ) ;
#13576=CARTESIAN_POINT ( 'NONE',  ( -24.31886431249228053, -24.10720463817513703, 4.330127018922217630 ) ) ;
#13577=CIRCLE ( 'NONE', #13280, 1.500000000000000888 ) ;
#13578=ORIENTED_EDGE ( 'NONE', *, *, #3267, .F. ) ;
#13579=CIRCLE ( 'NONE', #12667, 1.500000000000000888 ) ;
#13580=DIRECTION ( 'NONE',  ( -0.9876526153536336894, -0.1566598588826349503, 0.000000000000000000 ) ) ;
#13581=DIRECTION ( 'NONE',  ( -0.1566598588826321192, 0.9876526153536342445, 7.798540720466730171E-17 ) ) ;
#13582=CARTESIAN_POINT ( 'NONE',  ( -51.97313754239394257, -28.49368068688882971, -12.99038105676658006 ) ) ;
#13586=CIRCLE ( 'NONE', #7857, 1.500000000000000000 ) ;
#13588=ADVANCED_FACE ( 'NONE', ( #4782 ), #6425, .F. ) ;
#13589=FACE_OUTER_BOUND ( 'NONE', #13269, .T. ) ;
#13590=AXIS2_PLACEMENT_3D ( 'NONE', #11874, #16650, #17713 ) ;
#13591=EDGE_LOOP ( 'NONE', ( #15214, #38, #5064, #3539 ) ) ;
#13595=CIRCLE ( 'NONE', #18511, 1.499999999999999556 ) ;
#13597=ORIENTED_EDGE ( 'NONE', *, *, #17202, .T. ) ;
#13598=EDGE_CURVE ( 'NONE', #7971, #794, #13455, .T. ) ;
#13599=DIRECTION ( 'NONE',  ( -0.9876526153536341335, -0.1566598588826327576, 0.000000000000000000 ) ) ;
#13600=VERTEX_POINT ( 'NONE', #13771 ) ;
#13601=AXIS2_PLACEMENT_3D ( 'NONE', #222, #3233, #4853 ) ;
#13602=CARTESIAN_POINT ( 'NONE',  ( -2.096680467035594297, -20.58235781331593017, 1.540628126764003082E-14 ) ) ;
#13603=LINE ( 'NONE', #9640, #17795 ) ;
#13604=AXIS2_PLACEMENT_3D ( 'NONE', #2799, #8586, #14357 ) ;
#13605=CARTESIAN_POINT ( 'NONE',  ( -62.79768130110601021, -87.91612057094590682, -12.99038105676658539 ) ) ;
#13607=ORIENTED_EDGE ( 'NONE', *, *, #17809, .F. ) ;
#13608=DIRECTION ( 'NONE',  ( -0.1566598588826321192, 0.9876526153536342445, 7.798540720466730171E-17 ) ) ;
#13609=VECTOR ( 'NONE', #12475, 1000.000000000000000 ) ;
#13611=CARTESIAN_POINT ( 'NONE',  ( 0.000000000000000000, 0.000000000000000000, 0.000000000000000000 ) ) ;
#13612=CARTESIAN_POINT ( 'NONE',  ( -49.95819730150879678, -85.87954240547168183, 12.99038105676661203 ) ) ;
#13613=DIRECTION ( 'NONE',  ( -0.9876526153536336894, -0.1566598588826350336, 0.000000000000000000 ) ) ;
#13614=AXIS2_PLACEMENT_3D ( 'NONE', #7295, #8018, #10843 ) ;
#13615=FACE_OUTER_BOUND ( 'NONE', #5744, .T. ) ;
#13616=DIRECTION ( 'NONE',  ( -0.1566598588826321747, 0.9876526153536343555, 0.000000000000000000 ) ) ;
#13617=DIRECTION ( 'NONE',  ( -0.9876526153536336894, -0.1566598588826350336, 0.000000000000000000 ) ) ;
#13618=DIRECTION ( 'NONE',  ( -0.1566598588826321747, 0.9876526153536343555, 0.000000000000000000 ) ) ;
#13619=ORIENTED_EDGE ( 'NONE', *, *, #18600, .F. ) ;
#13620=ORIENTED_EDGE ( 'NONE', *, *, #12119, .F. ) ;
#13621=VECTOR ( 'NONE', #28, 1000.000000000000000 ) ;
#13623=EDGE_CURVE ( 'NONE', #3731, #5983, #11333, .T. ) ;
#13624=AXIS2_PLACEMENT_3D ( 'NONE', #11125, #9446, #13599 ) ;
#13625=CARTESIAN_POINT ( 'NONE',  ( -7.528769851480577202, -21.44398703717040888, 21.65063509461101177 ) ) ;
#13629=EDGE_CURVE ( 'NONE', #8364, #16586, #16509, .T. ) ;
#13631=CIRCLE ( 'NONE', #17302, 1.499999999999999556 ) ;
#13632=DIRECTION ( 'NONE',  ( -0.1566598588826321192, 0.9876526153536342445, 7.798540720466730171E-17 ) ) ;
#13633=CIRCLE ( 'NONE', #17618, 1.500000000000001332 ) ;
#13636=DIRECTION ( 'NONE',  ( -0.1566598588826321192, 0.9876526153536342445, 7.798540720466730171E-17 ) ) ;
#13637=CARTESIAN_POINT ( 'NONE',  ( -16.70711637639958269, -17.83733276090463704, 21.65063509461101532 ) ) ;
#13640=FACE_OUTER_BOUND ( 'NONE', #6395, .T. ) ;
#13641=AXIS2_PLACEMENT_3D ( 'NONE', #9172, #9072, #170 ) ;
#13643=ORIENTED_EDGE ( 'NONE', *, *, #17194, .F. ) ;
#13644=ORIENTED_EDGE ( 'NONE', *, *, #14501, .T. ) ;
#13645=ORIENTED_EDGE ( 'NONE', *, *, #17369, .F. ) ;
#13646=CARTESIAN_POINT ( 'NONE',  ( -81.73462711737164454, 33.01666666666666572, 35.00000000000000000 ) ) ;
#13647=EDGE_CURVE ( 'NONE', #9148, #16586, #12250, .T. ) ;
#13648=VECTOR ( 'NONE', #11380, 1000.000000000000000 ) ;
#13650=FACE_BOUND ( 'NONE', #7580, .T. ) ;
#13652=FACE_OUTER_BOUND ( 'NONE', #6182, .T. ) ;
#13653=CIRCLE ( 'NONE', #2170, 1.500000000000001332 ) ;
#13654=APPLICATION_CONTEXT ( 'automotive_design' ) ;
#13655=CARTESIAN_POINT ( 'NONE',  ( -36.46016868347218320, -20.97052993855728076, 21.65063509461102242 ) ) ;
#13656=VERTEX_POINT ( 'NONE', #17039 ) ;
#13658=CARTESIAN_POINT ( 'NONE',  ( -55.39028668595378946, -86.74117162932616054, -8.660254037844385522 ) ) ;
#13659=DIRECTION ( 'NONE',  ( -0.1566598588826321192, 0.9876526153536342445, 7.798540720466730171E-17 ) ) ;
#13660=CARTESIAN_POINT ( 'NONE',  ( 2.841582609732560272, -19.79905851890276836, 1.367155779166322214E-14 ) ) ;
#13661=VECTOR ( 'NONE', #12900, 1000.000000000000000 ) ;
#13662=CARTESIAN_POINT ( 'NONE',  ( -51.27495791377664602, -23.32042782179674134, -12.99038105676658006 ) ) ;
#13663=ORIENTED_EDGE ( 'NONE', *, *, #5464, .F. ) ;
#13665=LINE ( 'NONE', #13952, #6344 ) ;
#13666=EDGE_CURVE ( 'NONE', #13460, #7022, #15279, .T. ) ;
#13667=CARTESIAN_POINT ( 'NONE',  ( -29.05277406831996245, -19.79558099693753803, 8.660254037844417496 ) ) ;
#13671=DIRECTION ( 'NONE',  ( -0.1566598588826321747, 0.9876526153536343555, 0.000000000000000000 ) ) ;
#13674=ORIENTED_EDGE ( 'NONE', *, *, #16114, .F. ) ;
#13676=DIRECTION ( 'NONE',  ( 0.000000000000000000, 0.000000000000000000, 1.000000000000000000 ) ) ;
#13677=DIRECTION ( 'NONE',  ( -0.000000000000000000, -0.000000000000000000, -1.000000000000000000 ) ) ;
#13678=DIRECTION ( 'NONE',  ( -0.1566598588826321747, 0.9876526153536343555, 0.000000000000000000 ) ) ;
#13679=FACE_OUTER_BOUND ( 'NONE', #13836, .T. ) ;
#13680=DIRECTION ( 'NONE',  ( 0.000000000000000000, 0.000000000000000000, 1.000000000000000000 ) ) ;
#13681=CARTESIAN_POINT ( 'NONE',  ( -18.39294862037050393, -23.16724548487935564, -17.32050807568878170 ) ) ;
#13682=DIRECTION ( 'NONE',  ( -0.1566598588826321192, 0.9876526153536342445, 7.798540720466730171E-17 ) ) ;
#13683=ORIENTED_EDGE ( 'NONE', *, *, #12572, .F. ) ;
#13684=EDGE_LOOP ( 'NONE', ( #4017, #10789, #9329, #4325 ) ) ;
#13685=AXIS2_PLACEMENT_3D ( 'NONE', #602, #15185, #17773 ) ;
#13688=ORIENTED_EDGE ( 'NONE', *, *, #7708, .F. ) ;
#13689=EDGE_LOOP ( 'NONE', ( #13034, #9293 ) ) ;
#13690=VERTEX_POINT ( 'NONE', #6888 ) ;
#13691=CARTESIAN_POINT ( 'NONE',  ( -16.70711637639958269, -17.83733276090463704, -4.330127018922180326 ) ) ;
#13692=ADVANCED_FACE ( 'NONE', ( #15395 ), #1207, .F. ) ;
#13693=DIRECTION ( 'NONE',  ( -0.1566598588826321192, 0.9876526153536342445, 7.798540720466730171E-17 ) ) ;
#13694=EDGE_CURVE ( 'NONE', #18004, #15166, #17734, .T. ) ;
#13695=ORIENTED_EDGE ( 'NONE', *, *, #15526, .F. ) ;
#13697=CYLINDRICAL_SURFACE ( 'NONE', #7640, 1.500000000000001554 ) ;
#13699=DIRECTION ( 'NONE',  ( -0.9876526153536341335, -0.1566598588826327021, 0.000000000000000000 ) ) ;
#13701=VERTEX_POINT ( 'NONE', #2698 ) ;
#13702=FACE_OUTER_BOUND ( 'NONE', #640, .T. ) ;
#13704=VERTEX_POINT ( 'NONE', #9734 ) ;
#13705=EDGE_LOOP ( 'NONE', ( #10148, #7716 ) ) ;
#13707=AXIS2_PLACEMENT_3D ( 'NONE', #13713, #2256, #16795 ) ;
#13708=FACE_OUTER_BOUND ( 'NONE', #9822, .T. ) ;
#13709=ORIENTED_EDGE ( 'NONE', *, *, #18707, .F. ) ;
#13710=ORIENTED_EDGE ( 'NONE', *, *, #17153, .F. ) ;
#13711=CARTESIAN_POINT ( 'NONE',  ( -11.76885329963143079, -17.05403346649147878, 21.65063509461101532 ) ) ;
#13712=CARTESIAN_POINT ( 'NONE',  ( -18.35331361019266794, -80.86642692122748599, 21.65063509461101532 ) ) ;
#13713=CARTESIAN_POINT ( 'NONE',  ( -66.08974714408107332, -25.67032570503623035, 21.65063509461102242 ) ) ;
#13715=EDGE_CURVE ( 'NONE', #4657, #12177, #14392, .T. ) ;
#13716=DIRECTION ( 'NONE',  ( 0.000000000000000000, 0.000000000000000000, 1.000000000000000000 ) ) ;
#13717=DIRECTION ( 'NONE',  ( -0.9876526153536336894, -0.1566598588826349503, 0.000000000000000000 ) ) ;
#13718=CYLINDRICAL_SURFACE ( 'NONE', #1175, 1.500000000000001554 ) ;
#13719=VERTEX_POINT ( 'NONE', #4007 ) ;
#13720=DIRECTION ( 'NONE',  ( 0.000000000000000000, 0.000000000000000000, 1.000000000000000000 ) ) ;
#13721=CARTESIAN_POINT ( 'NONE',  ( -1.109027851681973598, -20.42569795443330349, -21.65063509461098334 ) ) ;
#13722=EDGE_CURVE ( 'NONE', #14919, #12166, #5913, .T. ) ;
#13724=VERTEX_POINT ( 'NONE', #18588 ) ;
#13726=ORIENTED_EDGE ( 'NONE', *, *, #5544, .F. ) ;
#13727=EDGE_LOOP ( 'NONE', ( #7578, #7982 ) ) ;
#13728=ORIENTED_EDGE ( 'NONE', *, *, #14044, .F. ) ;
#13729=CARTESIAN_POINT ( 'NONE',  ( -22.34355908178503469, -23.79388492040988012, 12.99038105676661736 ) ) ;
#13730=ORIENTED_EDGE ( 'NONE', *, *, #9598, .F. ) ;
#13731=VERTEX_POINT ( 'NONE', #11019 ) ;
#13732=FACE_BOUND ( 'NONE', #7765, .T. ) ;
#13733=ORIENTED_EDGE ( 'NONE', *, *, #4273, .F. ) ;
#13735=VECTOR ( 'NONE', #684, 1000.000000000000000 ) ;
#13736=VERTEX_POINT ( 'NONE', #6704 ) ;
#13739=EDGE_LOOP ( 'NONE', ( #5062, #954, #13469, #8369 ) ) ;
#13740=CYLINDRICAL_SURFACE ( 'NONE', #1870, 1.500000000000001554 ) ;
#13743=DIRECTION ( 'NONE',  ( -0.1566598588826321192, 0.9876526153536342445, 7.798540720466731404E-17 ) ) ;
#13744=DIRECTION ( 'NONE',  ( 0.000000000000000000, 0.000000000000000000, 1.000000000000000000 ) ) ;
#13745=EDGE_CURVE ( 'NONE', #4400, #8333, #11930, .T. ) ;
#13747=ORIENTED_EDGE ( 'NONE', *, *, #128, .T. ) ;
#13748=EDGE_LOOP ( 'NONE', ( #8922, #3729 ) ) ;
#13749=DIRECTION ( 'NONE',  ( -0.9876526153536341335, -0.1566598588826327021, 0.000000000000000000 ) ) ;
#13751=FACE_OUTER_BOUND ( 'NONE', #7761, .T. ) ;
#13753=ORIENTED_EDGE ( 'NONE', *, *, #13424, .F. ) ;
#13755=ORIENTED_EDGE ( 'NONE', *, *, #17637, .T. ) ;
#13759=EDGE_CURVE ( 'NONE', #18515, #10629, #921, .T. ) ;
#13760=CARTESIAN_POINT ( 'NONE',  ( -66.25446545484369665, -88.46443007703511796, -4.330127018922185655 ) ) ;
#13761=VECTOR ( 'NONE', #15783, 1000.000000000000000 ) ;
#13762=DIRECTION ( 'NONE',  ( -0.1566598588826321747, 0.9876526153536343555, 0.000000000000000000 ) ) ;
#13764=EDGE_CURVE ( 'NONE', #6194, #15676, #1689, .T. ) ;
#13765=EDGE_CURVE ( 'NONE', #14520, #16637, #4693, .T. ) ;
#13766=EDGE_CURVE ( 'NONE', #697, #6194, #18387, .T. ) ;
#13767=LINE ( 'NONE', #3805, #14221 ) ;
#13769=CARTESIAN_POINT ( 'NONE',  ( -1.109027851681966492, -20.42569795443330349, 4.330127018922212301 ) ) ;
#13771=CARTESIAN_POINT ( 'NONE',  ( -71.23236354178969520, -31.54854793510013877, -8.660254037844380193 ) ) ;
#13772=ORIENTED_EDGE ( 'NONE', *, *, #6220, .T. ) ;
#13774=DIRECTION ( 'NONE',  ( -0.9876526153536341335, -0.1566598588826327021, 0.000000000000000000 ) ) ;
#13777=VECTOR ( 'NONE', #8258, 1000.000000000000000 ) ;
#13779=CYLINDRICAL_SURFACE ( 'NONE', #15341, 1.500000000000001554 ) ;
#13780=DIRECTION ( 'NONE',  ( -0.9876526153536344665, -0.1566598588826304539, 0.000000000000000000 ) ) ;
#13783=ORIENTED_EDGE ( 'NONE', *, *, #17071, .F. ) ;
#13785=EDGE_CURVE ( 'NONE', #14796, #13180, #17600, .T. ) ;
#13786=LINE ( 'NONE', #455, #1199 ) ;
#13787=AXIS2_PLACEMENT_3D ( 'NONE', #18319, #8024, #18513 ) ;
#13788=ORIENTED_EDGE ( 'NONE', *, *, #6994, .T. ) ;
#13789=CARTESIAN_POINT ( 'NONE',  ( -4.526176995241833367, -78.67318889687062722, -8.660254037844385522 ) ) ;
#13790=DIRECTION ( 'NONE',  ( -0.9876526153536336894, -0.1566598588826349503, 0.000000000000000000 ) ) ;
#13791=VERTEX_POINT ( 'NONE', #14638 ) ;
#13793=DIRECTION ( 'NONE',  ( -0.1566598588826321192, 0.9876526153536342445, 7.798540720466730171E-17 ) ) ;
#13795=ORIENTED_EDGE ( 'NONE', *, *, #17511, .T. ) ;
#13796=EDGE_CURVE ( 'NONE', #5804, #11671, #15289, .T. ) ;
#13797=DIRECTION ( 'NONE',  ( -0.1566598588826321192, 0.9876526153536342445, 7.798540720466730171E-17 ) ) ;
#13798=VERTEX_POINT ( 'NONE', #14448 ) ;
#13799=AXIS2_PLACEMENT_3D ( 'NONE', #10406, #5970, #11719 ) ;
#13800=EDGE_LOOP ( 'NONE', ( #1559, #12687, #17896, #9424 ) ) ;
#13801=ORIENTED_EDGE ( 'NONE', *, *, #6633, .T. ) ;
#13802=AXIS2_PLACEMENT_3D ( 'NONE', #11683, #17625, #11955 ) ;
#13804=ORIENTED_EDGE ( 'NONE', *, *, #5088, .T. ) ;
#13805=EDGE_LOOP ( 'NONE', ( #12026, #3797, #12588, #1352 ) ) ;
#13806=CARTESIAN_POINT ( 'NONE',  ( 55.85952145814821534, 6.938893903907228378E-15, 24.99999999999998224 ) ) ;
#13807=FACE_OUTER_BOUND ( 'NONE', #9016, .T. ) ;
#13808=ORIENTED_EDGE ( 'NONE', *, *, #11491, .F. ) ;
#13809=DIRECTION ( 'NONE',  ( -0.1566598588826321747, 0.9876526153536343555, 0.000000000000000000 ) ) ;
#13811=DIRECTION ( 'NONE',  ( -0.9876526153536341335, -0.1566598588826327021, 0.000000000000000000 ) ) ;
#13813=AXIS2_PLACEMENT_3D ( 'NONE', #14655, #7551, #1594 ) ;
#13814=AXIS2_PLACEMENT_3D ( 'NONE', #12472, #3824, #7837 ) ;
#13815=CARTESIAN_POINT ( 'NONE',  ( -67.77557938805200877, -31.00023842901093118, -17.32050807568878170 ) ) ;
#13816=VERTEX_POINT ( 'NONE', #7526 ) ;
#13817=DIRECTION ( 'NONE',  ( -0.9876526153536341335, -0.1566598588826327021, 0.000000000000000000 ) ) ;
#13819=LINE ( 'NONE', #12008, #6438 ) ;
#13821=AXIS2_PLACEMENT_3D ( 'NONE', #8489, #2961, #15782 ) ;
#13823=EDGE_CURVE ( 'NONE', #15970, #5513, #11397, .T. ) ;
#13825=ORIENTED_EDGE ( 'NONE', *, *, #15389, .T. ) ;
#13826=DIRECTION ( 'NONE',  ( 1.000000000000000000, 0.000000000000000000, -2.887450008416415878E-16 ) ) ;
#13827=EDGE_CURVE ( 'NONE', #13088, #12921, #14094, .T. ) ;
#13828=ORIENTED_EDGE ( 'NONE', *, *, #1446, .F. ) ;
#13829=CARTESIAN_POINT ( 'NONE',  ( -10.28737437660097775, -16.81904367816753165, 12.99038105676661381 ) ) ;
#13831=ORIENTED_EDGE ( 'NONE', *, *, #3146, .F. ) ;
#13832=ORIENTED_EDGE ( 'NONE', *, *, #7142, .F. ) ;
#13833=FACE_OUTER_BOUND ( 'NONE', #4511, .T. ) ;
#13834=VECTOR ( 'NONE', #9838, 1000.000000000000000 ) ;
#13835=EDGE_CURVE ( 'NONE', #6362, #6405, #4093, .T. ) ;
#13836=EDGE_LOOP ( 'NONE', ( #6783, #14977, #923, #15432 ) ) ;
#13837=FACE_BOUND ( 'NONE', #16344, .T. ) ;
#13838=LINE ( 'NONE', #2567, #6754 ) ;
#13839=FACE_OUTER_BOUND ( 'NONE', #3051, .T. ) ;
#13840=DIRECTION ( 'NONE',  ( -0.1566598588826321192, 0.9876526153536342445, 7.798540720466731404E-17 ) ) ;
#13841=ORIENTED_EDGE ( 'NONE', *, *, #11766, .F. ) ;
#13842=LINE ( 'NONE', #9590, #16045 ) ;
#13843=DIRECTION ( 'NONE',  ( -0.1566598588826321192, 0.9876526153536342445, 7.798540720466730171E-17 ) ) ;
#13844=AXIS2_PLACEMENT_3D ( 'NONE', #14651, #13211, #7102 ) ;
#13845=VERTEX_POINT ( 'NONE', #8588 ) ;
#13846=ORIENTED_EDGE ( 'NONE', *, *, #1522, .F. ) ;
#13847=DIRECTION ( 'NONE',  ( -0.1566598588826321747, 0.9876526153536343555, 0.000000000000000000 ) ) ;
#13848=CIRCLE ( 'NONE', #5993, 1.500000000000001332 ) ;
#13852=CARTESIAN_POINT ( 'NONE',  ( -84.23462711737164454, 33.01666666666666572, -35.00000000000000000 ) ) ;
#13854=ORIENTED_EDGE ( 'NONE', *, *, #7682, .T. ) ;
#13855=ORIENTED_EDGE ( 'NONE', *, *, #9686, .T. ) ;
#13860=DIRECTION ( 'NONE',  ( -0.1566598588826321192, 0.9876526153536342445, 7.798540720466730171E-17 ) ) ;
#13862=CIRCLE ( 'NONE', #12337, 1.500000000000000888 ) ;
#13863=CARTESIAN_POINT ( 'NONE',  ( -31.52190560670403841, -20.18723064414411184, -4.330127018922180326 ) ) ;
#13865=CIRCLE ( 'NONE', #13254, 1.500000000000000444 ) ;
#13868=CIRCLE ( 'NONE', #5732, 1.500000000000000888 ) ;
#13870=CARTESIAN_POINT ( 'NONE',  ( -74.19532138785061193, -32.01852751174804013, -8.660254037844380193 ) ) ;
#13871=ORIENTED_EDGE ( 'NONE', *, *, #11793, .F. ) ;
#13872=ORIENTED_EDGE ( 'NONE', *, *, #6910, .T. ) ;
#13873=PLANE ( 'NONE',  #15727 ) ;
#13874=FACE_OUTER_BOUND ( 'NONE', #10840, .T. ) ;
#13876=AXIS2_PLACEMENT_3D ( 'NONE', #4737, #13447, #4648 ) ;
#13878=VECTOR ( 'NONE', #10033, 1000.000000000000000 ) ;
#13879=AXIS2_PLACEMENT_3D ( 'NONE', #3562, #848, #6626 ) ;
#13880=ORIENTED_EDGE ( 'NONE', *, *, #17707, .T. ) ;
#13882=VERTEX_POINT ( 'NONE', #15961 ) ;
#13883=CARTESIAN_POINT ( 'NONE',  ( -74.97862068226375243, -27.08026443497990599, 1.908195823574487804E-14 ) ) ;
#13884=CARTESIAN_POINT ( 'NONE',  ( -56.91140061916208026, -29.27697998130198442, 12.99038105676661736 ) ) ;
#13885=ADVANCED_FACE ( 'NONE', ( #1386 ), #7168, .F. ) ;
#13887=DIRECTION ( 'NONE',  ( -0.1566598588826321747, 0.9876526153536343555, 0.000000000000000000 ) ) ;
#13889=DIRECTION ( 'NONE',  ( -0.1566598588826321192, 0.9876526153536342445, 7.798540720466730171E-17 ) ) ;
#13892=ORIENTED_EDGE ( 'NONE', *, *, #5305, .T. ) ;
#13893=CARTESIAN_POINT ( 'NONE',  ( -8.516422466834198346, -21.60064689605303911, 8.660254037844413944 ) ) ;
#13895=CIRCLE ( 'NONE', #12944, 1.500000000000001332 ) ;
#13896=FACE_OUTER_BOUND ( 'NONE', #2142, .T. ) ;
#13897=AXIS2_PLACEMENT_3D ( 'NONE', #726, #13238, #14767 ) ;
#13899=DIRECTION ( 'NONE',  ( -0.1566598588826321192, 0.9876526153536342445, 7.798540720466730171E-17 ) ) ;
#13900=ORIENTED_EDGE ( 'NONE', *, *, #14368, .T. ) ;
#13901=DIRECTION ( 'NONE',  ( -0.1566598588826321192, 0.9876526153536342445, 7.798540720466730171E-17 ) ) ;
#13902=CARTESIAN_POINT ( 'NONE',  ( -4.361458684479201153, -15.87908452487173427, -17.32050807568878170 ) ) ;
#13903=EDGE_LOOP ( 'NONE', ( #18552, #9365 ) ) ;
#13904=AXIS2_PLACEMENT_3D ( 'NONE', #15239, #5300, #6455 ) ;
#13905=VERTEX_POINT ( 'NONE', #4665 ) ;
#13906=AXIS2_PLACEMENT_3D ( 'NONE', #16956, #12550, #1219 ) ;
#13907=LINE ( 'NONE', #667, #13215 ) ;
#13908=EDGE_LOOP ( 'NONE', ( #6780, #14390 ) ) ;
#13909=ORIENTED_EDGE ( 'NONE', *, *, #3653, .T. ) ;
#13910=CIRCLE ( 'NONE', #6670, 1.499999999999999556 ) ;
#13911=ADVANCED_FACE ( 'NONE', ( #2204 ), #12137, .F. ) ;
#13912=VECTOR ( 'NONE', #13359, 1000.000000000000000 ) ;
#13913=CARTESIAN_POINT ( 'NONE',  ( -34.68921677370540380, -25.75213315644277046, -8.660254037844380193 ) ) ;
#13914=CYLINDRICAL_SURFACE ( 'NONE', #17701, 1.500000000000001554 ) ;
#13916=DIRECTION ( 'NONE',  ( -0.1566598588826321192, 0.9876526153536342445, 7.798540720466731404E-17 ) ) ;
#13917=EDGE_CURVE ( 'NONE', #9536, #491, #16239, .T. ) ;
#13918=CIRCLE ( 'NONE', #1250, 1.499999999999999556 ) ;
#13920=DIRECTION ( 'NONE',  ( -0.9876526153536336894, -0.1566598588826349503, 0.000000000000000000 ) ) ;
#13921=AXIS2_PLACEMENT_3D ( 'NONE', #14423, #8564, #5427 ) ;
#13922=CARTESIAN_POINT ( 'NONE',  ( -47.81817376003892406, -22.77211831570753731, 4.330127018922218518 ) ) ;
#13923=LINE ( 'NONE', #973, #13777 ) ;
#13926=CARTESIAN_POINT ( 'NONE',  ( -73.49714175923330117, -26.84527464665596597, 17.32050807568882078 ) ) ;
#13927=CIRCLE ( 'NONE', #6690, 1.500000000000000888 ) ;
#13928=CARTESIAN_POINT ( 'NONE',  ( -6.830590222863280658, -16.27073417207831696, 21.65063509461101532 ) ) ;
#13929=ORIENTED_EDGE ( 'NONE', *, *, #1377, .T. ) ;
#13931=CIRCLE ( 'NONE', #10901, 1.500000000000001332 ) ;
#13933=DIRECTION ( 'NONE',  ( -0.9876526153536336894, -0.1566598588826349503, 0.000000000000000000 ) ) ;
#13935=ORIENTED_EDGE ( 'NONE', *, *, #2761, .T. ) ;
#13936=FACE_BOUND ( 'NONE', #10899, .T. ) ;
#13937=CARTESIAN_POINT ( 'NONE',  ( -61.35583738825340561, -29.98194934627382224, -17.32050807568878170 ) ) ;
#13938=EDGE_CURVE ( 'NONE', #16948, #15907, #11933, .T. ) ;
#13939=AXIS2_PLACEMENT_3D ( 'NONE', #7178, #17420, #17234 ) ;
#13940=EDGE_CURVE ( 'NONE', #9536, #16948, #1395, .T. ) ;
#13941=FACE_OUTER_BOUND ( 'NONE', #10201, .T. ) ;
#13942=AXIS2_PLACEMENT_3D ( 'NONE', #8091, #15493, #5547 ) ;
#13943=DIRECTION ( 'NONE',  ( -0.1566598588826321192, 0.9876526153536342445, 7.798540720466731404E-17 ) ) ;
#13946=EDGE_LOOP ( 'NONE', ( #7227, #14011, #12282, #18725 ) ) ;
#13947=AXIS2_PLACEMENT_3D ( 'NONE', #15503, #15399, #16657 ) ;
#13948=DIRECTION ( 'NONE',  ( 0.000000000000000000, 0.000000000000000000, 1.000000000000000000 ) ) ;
#13949=CARTESIAN_POINT ( 'NONE',  ( -17.85948730251583783, -80.78809699178616199, 1.443110928631665584E-14 ) ) ;
#13950=DIRECTION ( 'NONE',  ( -0.1566598588826321192, 0.9876526153536342445, 7.798540720466731404E-17 ) ) ;
#13952=CARTESIAN_POINT ( 'NONE',  ( -67.73594437787414790, -88.69941986535906153, 12.99038105676661203 ) ) ;
#13953=AXIS2_PLACEMENT_3D ( 'NONE', #7072, #18659, #4189 ) ;
#13954=DIRECTION ( 'NONE',  ( -0.1566598588826321747, 0.9876526153536343555, 0.000000000000000000 ) ) ;
#13955=ORIENTED_EDGE ( 'NONE', *, *, #18523, .T. ) ;
#13957=ORIENTED_EDGE ( 'NONE', *, *, #10860, .T. ) ;
#13958=ORIENTED_EDGE ( 'NONE', *, *, #11227, .F. ) ;
#13959=FACE_OUTER_BOUND ( 'NONE', #8839, .T. ) ;
#13961=ORIENTED_EDGE ( 'NONE', *, *, #353, .F. ) ;
#13965=LINE ( 'NONE', #6980, #8211 ) ;
#13966=AXIS2_PLACEMENT_3D ( 'NONE', #16887, #3855, #17442 ) ;
#13967=CARTESIAN_POINT ( 'NONE',  ( -47.48906576312472794, -85.48789275826510448, 8.660254037844412167 ) ) ;
#13968=LINE ( 'NONE', #8376, #865 ) ;
#13970=EDGE_LOOP ( 'NONE', ( #1154, #17178, #4713, #14144 ) ) ;
#13971=EDGE_CURVE ( 'NONE', #2873, #1264, #13467, .T. ) ;
#13973=DIRECTION ( 'NONE',  ( -0.1566598588826321192, 0.9876526153536342445, 7.798540720466730171E-17 ) ) ;
#13975=DIRECTION ( 'NONE',  ( -0.1566598588826321747, 0.9876526153536343555, 0.000000000000000000 ) ) ;
#13977=DIRECTION ( 'NONE',  ( 0.000000000000000000, 0.000000000000000000, 1.000000000000000000 ) ) ;
#13978=ORIENTED_EDGE ( 'NONE', *, *, #7059, .T. ) ;
#13979=ORIENTED_EDGE ( 'NONE', *, *, #9840, .F. ) ;
#13980=DIRECTION ( 'NONE',  ( -0.9876526153536341335, -0.1566598588826327021, 0.000000000000000000 ) ) ;
#13981=ORIENTED_EDGE ( 'NONE', *, *, #1850, .F. ) ;
#13982=EDGE_CURVE ( 'NONE', #5011, #9895, #12242, .T. ) ;
#13983=VECTOR ( 'NONE', #11134, 1000.000000000000000 ) ;
#13984=ORIENTED_EDGE ( 'NONE', *, *, #13647, .T. ) ;
#13986=EDGE_LOOP ( 'NONE', ( #9554, #17606, #16189, #12544 ) ) ;
#13987=ORIENTED_EDGE ( 'NONE', *, *, #16437, .F. ) ;
#13988=DIRECTION ( 'NONE',  ( -0.9876526153536341335, -0.1566598588826327021, 0.000000000000000000 ) ) ;
#13990=AXIS2_PLACEMENT_3D ( 'NONE', #12502, #11068, #16893 ) ;
#13992=DIRECTION ( 'NONE',  ( -0.1566598588826321747, 0.9876526153536343555, 0.000000000000000000 ) ) ;
#13993=CARTESIAN_POINT ( 'NONE',  ( -47.03487446562579066, -27.71038139247566079, -12.99038105676658006 ) ) ;
#13995=DIRECTION ( 'NONE',  ( -0.1566598588826321192, 0.9876526153536342445, 7.798540720466730171E-17 ) ) ;
#13997=EDGE_CURVE ( 'NONE', #11883, #4233, #4855, .T. ) ;
#13998=CARTESIAN_POINT ( 'NONE',  ( -36.66452200441265319, -26.06545287420802737, 17.32050807568881723 ) ) ;
#13999=VERTEX_POINT ( 'NONE', #15001 ) ;
#14000=LINE ( 'NONE', #3939, #502 ) ;
#14002=ORIENTED_EDGE ( 'NONE', *, *, #8796, .T. ) ;
#14003=CARTESIAN_POINT ( 'NONE',  ( -84.16561914167408531, 33.59999999999999432, 30.00000000000000000 ) ) ;
#14004=EDGE_CURVE ( 'NONE', #2756, #10533, #12227, .T. ) ;
#14005=CARTESIAN_POINT ( 'NONE',  ( -45.01993422474065198, -85.09624311105852712, 12.99038105676661203 ) ) ;
#14006=VERTEX_POINT ( 'NONE', #7803 ) ;
#14007=EDGE_CURVE ( 'NONE', #5362, #3259, #16210, .T. ) ;
#14008=LINE ( 'NONE', #60, #10499 ) ;
#14009=DIRECTION ( 'NONE',  ( -0.9876526153536336894, -0.1566598588826350336, 0.000000000000000000 ) ) ;
#14010=DIRECTION ( 'NONE',  ( -0.1566598588826321192, 0.9876526153536342445, 7.798540720466730171E-17 ) ) ;
#14011=ORIENTED_EDGE ( 'NONE', *, *, #18162, .T. ) ;
#14012=ORIENTED_EDGE ( 'NONE', *, *, #4930, .F. ) ;
#14013=AXIS2_PLACEMENT_3D ( 'NONE', #17461, #4365, #7137 ) ;
#14014=LINE ( 'NONE', #758, #16730 ) ;
#14015=DIRECTION ( 'NONE',  ( 0.000000000000000000, 0.000000000000000000, 1.000000000000000000 ) ) ;
#14016=DIRECTION ( 'NONE',  ( -0.1566598588826321747, 0.9876526153536343555, 0.000000000000000000 ) ) ;
#14017=DIRECTION ( 'NONE',  ( -0.9876526153536341335, -0.1566598588826327021, 0.000000000000000000 ) ) ;
#14019=DIRECTION ( 'NONE',  ( -0.1566598588826321747, 0.9876526153536343555, 0.000000000000000000 ) ) ;
#14020=CARTESIAN_POINT ( 'NONE',  ( -39.09401853261887538, -84.15628395776273862, 17.32050807568881368 ) ) ;
#14021=CARTESIAN_POINT ( 'NONE',  ( -36.62488699423481364, -83.76463431055616127, -12.99038105676658539 ) ) ;
#14022=ADVANCED_FACE ( 'NONE', ( #17884 ), #14815, .F. ) ;
#14023=ADVANCED_FACE ( 'NONE', ( #13385 ), #4762, .F. ) ;
#14024=CARTESIAN_POINT ( 'NONE',  ( -26.74836084069850983, -82.19803572172985184, 12.99038105676661203 ) ) ;
#14025=CARTESIAN_POINT ( 'NONE',  ( 55.85952145814821534, 6.938893903907228378E-15, -30.00000000000000000 ) ) ;
#14026=AXIS2_PLACEMENT_3D ( 'NONE', #8967, #451, #13502 ) ;
#14027=EDGE_CURVE ( 'NONE', #18222, #10290, #7446, .T. ) ;
#14028=CYLINDRICAL_SURFACE ( 'NONE', #1510, 1.500000000000001554 ) ;
#14029=ORIENTED_EDGE ( 'NONE', *, *, #16792, .F. ) ;
#14030=ORIENTED_EDGE ( 'NONE', *, *, #7308, .T. ) ;
#14031=CYLINDRICAL_SURFACE ( 'NONE', #5346, 139.0000000000000000 ) ;
#14032=FACE_BOUND ( 'NONE', #8551, .T. ) ;
#14033=FACE_OUTER_BOUND ( 'NONE', #7457, .T. ) ;
#14034=EDGE_CURVE ( 'NONE', #9121, #7348, #1101, .T. ) ;
#14035=DIRECTION ( 'NONE',  ( -0.1566598588826321192, 0.9876526153536342445, 7.798540720466730171E-17 ) ) ;
#14037=DIRECTION ( 'NONE',  ( -0.1566598588826321747, 0.9876526153536343555, 0.000000000000000000 ) ) ;
#14038=DIRECTION ( 'NONE',  ( -0.9876526153536336894, -0.1566598588826349503, 0.000000000000000000 ) ) ;
#14039=CYLINDRICAL_SURFACE ( 'NONE', #13921, 1.500000000000001554 ) ;
#14040=CARTESIAN_POINT ( 'NONE',  ( -14.23798483801550674, -17.44568311369805969, 8.660254037844413944 ) ) ;
#14041=CARTESIAN_POINT ( 'NONE',  ( -44.03228160938704860, -84.93958325217589334, -17.32050807568878525 ) ) ;
#14042=CYLINDRICAL_SURFACE ( 'NONE', #3554, 1.500000000000000666 ) ;
#14043=DIRECTION ( 'NONE',  ( -0.1566598588826321192, 0.9876526153536342445, 7.798540720466731404E-17 ) ) ;
#14044=EDGE_CURVE ( 'NONE', #17286, #17191, #12431, .T. ) ;
#14045=DIRECTION ( 'NONE',  ( -0.000000000000000000, -0.000000000000000000, -1.000000000000000000 ) ) ;
#14048=CARTESIAN_POINT ( 'NONE',  ( -14.40270314877813895, -80.23978748569695085, -8.660254037844385522 ) ) ;
#14049=EDGE_CURVE ( 'NONE', #16555, #5480, #17748, .T. ) ;
#14050=EDGE_LOOP ( 'NONE', ( #17681, #2427 ) ) ;
#14051=VERTEX_POINT ( 'NONE', #15475 ) ;
#14055=CARTESIAN_POINT ( 'NONE',  ( -2.057045456857760524, -78.28153924966404986, -21.65063509461098690 ) ) ;
#14056=CARTESIAN_POINT ( 'NONE',  ( -55.39028668595378946, -86.74117162932614633, -17.32050807568878525 ) ) ;
#14060=CIRCLE ( 'NONE', #5907, 1.500000000000000888 ) ;
#14061=CARTESIAN_POINT ( 'NONE',  ( -67.57122606711153878, -25.90531549336016681, -4.330127018922180326 ) ) ;
#14065=ORIENTED_EDGE ( 'NONE', *, *, #13501, .T. ) ;
#14066=DIRECTION ( 'NONE',  ( -0.1566598588826321192, 0.9876526153536342445, 7.798540720466730171E-17 ) ) ;
#14067=DIRECTION ( 'NONE',  ( 0.000000000000000000, 0.000000000000000000, 1.000000000000000000 ) ) ;
#14068=EDGE_CURVE ( 'NONE', #3602, #13155, #1982, .T. ) ;
#14070=DIRECTION ( 'NONE',  ( -0.9876526153536336894, -0.1566598588826349503, 0.000000000000000000 ) ) ;
#14071=ORIENTED_EDGE ( 'NONE', *, *, #17095, .F. ) ;
#14072=ORIENTED_EDGE ( 'NONE', *, *, #9814, .T. ) ;
#14074=LINE ( 'NONE', #4018, #12110 ) ;
#14075=EDGE_CURVE ( 'NONE', #1785, #2756, #3477, .T. ) ;
#14076=VECTOR ( 'NONE', #4506, 1000.000000000000000 ) ;
#14077=CARTESIAN_POINT ( 'NONE',  ( -52.42732883989288695, -86.27119205267825919, -8.660254037844385522 ) ) ;
#14078=EDGE_LOOP ( 'NONE', ( #11926, #3410, #11001, #3237 ) ) ;
#14080=CARTESIAN_POINT ( 'NONE',  ( -52.96079015774756726, -28.65034054577146705, -8.660254037844380193 ) ) ;
#14081=DIRECTION ( 'NONE',  ( -0.1566598588826321747, 0.9876526153536343555, 0.000000000000000000 ) ) ;
#14088=ORIENTED_EDGE ( 'NONE', *, *, #878, .F. ) ;
#14089=CARTESIAN_POINT ( 'NONE',  ( -58.68235252892886678, -24.49537676341647696, -17.32050807568878170 ) ) ;
#14090=CARTESIAN_POINT ( 'NONE',  ( -6.995308533625909320, -79.06483854407720457, -12.99038105676658539 ) ) ;
#14091=ORIENTED_EDGE ( 'NONE', *, *, #11233, .T. ) ;
#14093=DIRECTION ( 'NONE',  ( 0.000000000000000000, 0.000000000000000000, 1.000000000000000000 ) ) ;
#14094=CIRCLE ( 'NONE', #18683, 1.499999999999999556 ) ;
#14096=VERTEX_POINT ( 'NONE', #6573 ) ;
#14097=DIRECTION ( 'NONE',  ( -0.1566598588826321192, 0.9876526153536342445, 7.798540720466730171E-17 ) ) ;
#14098=ORIENTED_EDGE ( 'NONE', *, *, #4343, .T. ) ;
#14099=VECTOR ( 'NONE', #5619, 1000.000000000000000 ) ;
#14100=EDGE_CURVE ( 'NONE', #14196, #16138, #13173, .T. ) ;
#14101=LINE ( 'NONE', #12662, #11815 ) ;
#14103=DIRECTION ( 'NONE',  ( -0.1566598588826321192, 0.9876526153536342445, 7.798540720466730171E-17 ) ) ;
#14107=CARTESIAN_POINT ( 'NONE',  ( -47.03487446562579066, -27.71038139247566079, -4.330127018922181215 ) ) ;
#14108=DIRECTION ( 'NONE',  ( -0.1566598588826321192, 0.9876526153536342445, 7.798540720466730171E-17 ) ) ;
#14109=FACE_OUTER_BOUND ( 'NONE', #10871, .T. ) ;
#14111=CARTESIAN_POINT ( 'NONE',  ( -30.04042668367358360, -19.95224085582016826, -4.330127018922180326 ) ) ;
#14114=CARTESIAN_POINT ( 'NONE',  ( -13.45468554360235203, -22.38394619046619383, 8.660254037844413944 ) ) ;
#14115=CIRCLE ( 'NONE', #6877, 1.500000000000001332 ) ;
#14116=ORIENTED_EDGE ( 'NONE', *, *, #16402, .T. ) ;
#14117=ORIENTED_EDGE ( 'NONE', *, *, #6302, .F. ) ;
#14118=FACE_OUTER_BOUND ( 'NONE', #17978, .T. ) ;
#14119=ORIENTED_EDGE ( 'NONE', *, *, #15384, .T. ) ;
#14120=CARTESIAN_POINT ( 'NONE',  ( -62.83731631128386397, -30.21693913459777647, 1.869203119972154228E-14 ) ) ;
#14121=ORIENTED_EDGE ( 'NONE', *, *, #18125, .F. ) ;
#14122=FACE_BOUND ( 'NONE', #779, .T. ) ;
#14123=AXIS2_PLACEMENT_3D ( 'NONE', #8518, #18321, #6915 ) ;
#14124=ADVANCED_FACE ( 'NONE', ( #12521 ), #16917, .F. ) ;
#14125=DIRECTION ( 'NONE',  ( -0.1566598588826321192, 0.9876526153536342445, 7.798540720466730171E-17 ) ) ;
#14126=EDGE_CURVE ( 'NONE', #537, #17063, #11347, .T. ) ;
#14127=VECTOR ( 'NONE', #9190, 1000.000000000000000 ) ;
#14128=EDGE_CURVE ( 'NONE', #15897, #10670, #16532, .T. ) ;
#14131=EDGE_CURVE ( 'NONE', #11609, #4488, #2896, .T. ) ;
#14132=CARTESIAN_POINT ( 'NONE',  ( -40.57549745564932664, -84.39127374608669641, 17.32050807568881368 ) ) ;
#14133=ORIENTED_EDGE ( 'NONE', *, *, #13411, .T. ) ;
#14134=EDGE_CURVE ( 'NONE', #14620, #9571, #9258, .T. ) ;
#14135=AXIS2_PLACEMENT_3D ( 'NONE', #13154, #8814, #4631 ) ;
#14136=EDGE_LOOP ( 'NONE', ( #3916, #13371, #15625, #2737 ) ) ;
#14137=CYLINDRICAL_SURFACE ( 'NONE', #8357, 1.500000000000000666 ) ;
#14138=DIRECTION ( 'NONE',  ( -0.1566598588826321192, 0.9876526153536342445, 7.798540720466730171E-17 ) ) ;
#14139=DIRECTION ( 'NONE',  ( -0.1566598588826321192, 0.9876526153536342445, 7.798540720466730171E-17 ) ) ;
#14140=CIRCLE ( 'NONE', #12605, 1.499999999999999556 ) ;
#14141=CARTESIAN_POINT ( 'NONE',  ( -49.50400600400985240, -28.10203103968224880, 8.660254037844417496 ) ) ;
#14142=AXIS2_PLACEMENT_3D ( 'NONE', #17936, #3466, #13617 ) ;
#14144=ORIENTED_EDGE ( 'NONE', *, *, #12142, .F. ) ;
#14145=ORIENTED_EDGE ( 'NONE', *, *, #18581, .F. ) ;
#14146=ORIENTED_EDGE ( 'NONE', *, *, #10173, .F. ) ;
#14148=VERTEX_POINT ( 'NONE', #10974 ) ;
#14150=DIRECTION ( 'NONE',  ( -0.1566598588826321192, 0.9876526153536342445, 7.798540720466730171E-17 ) ) ;
#14151=VECTOR ( 'NONE', #3793, 1000.000000000000000 ) ;
#14152=FACE_OUTER_BOUND ( 'NONE', #16782, .T. ) ;
#14153=EDGE_CURVE ( 'NONE', #9188, #15027, #6938, .T. ) ;
#14154=DIRECTION ( 'NONE',  ( -0.1566598588826321192, 0.9876526153536342445, 7.798540720466730171E-17 ) ) ;
#14155=CARTESIAN_POINT ( 'NONE',  ( -43.04462899403340970, -84.78292339329327376, -4.330127018922185655 ) ) ;
#14159=EDGE_CURVE ( 'NONE', #16087, #5366, #16802, .T. ) ;
#14160=VERTEX_POINT ( 'NONE', #12403 ) ;
#14161=CARTESIAN_POINT ( 'NONE',  ( -72.71384246482016067, -31.78353772342409300, -8.660254037844380193 ) ) ;
#14162=DIRECTION ( 'NONE',  ( -0.1566598588826321747, 0.9876526153536343555, 0.000000000000000000 ) ) ;
#14163=CIRCLE ( 'NONE', #3254, 1.500000000000000444 ) ;
#14164=CARTESIAN_POINT ( 'NONE',  ( -2.057045456857756971, -78.28153924966404986, 21.65063509461100821 ) ) ;
#14165=CARTESIAN_POINT ( 'NONE',  ( -50.49165861936349131, -28.25869089856488614, -21.65063509461098334 ) ) ;
#14166=ORIENTED_EDGE ( 'NONE', *, *, #15667, .F. ) ;
#14169=DIRECTION ( 'NONE',  ( -0.1566598588826321192, 0.9876526153536342445, 7.798540720466731404E-17 ) ) ;
#14170=VERTEX_POINT ( 'NONE', #9676 ) ;
#14171=CIRCLE ( 'NONE', #9008, 1.500000000000000444 ) ;
#14172=DIRECTION ( 'NONE',  ( -0.1566598588826321747, 0.9876526153536343555, 0.000000000000000000 ) ) ;
#14173=AXIS2_PLACEMENT_3D ( 'NONE', #5558, #16066, #14363 ) ;
#14174=ORIENTED_EDGE ( 'NONE', *, *, #12886, .T. ) ;
#14175=DIRECTION ( 'NONE',  ( -0.1566598588826321192, 0.9876526153536342445, 7.798540720466730171E-17 ) ) ;
#14176=AXIS2_PLACEMENT_3D ( 'NONE', #2866, #8484, #15660 ) ;
#14177=AXIS2_PLACEMENT_3D ( 'NONE', #5454, #3909, #15498 ) ;
#14178=DIRECTION ( 'NONE',  ( -0.1566598588826321192, 0.9876526153536342445, 7.798540720466730171E-17 ) ) ;
#14179=( GEOMETRIC_REPRESENTATION_CONTEXT ( 3 ) GLOBAL_UNCERTAINTY_ASSIGNED_CONTEXT ( ( #6464 ) ) GLOBAL_UNIT_ASSIGNED_CONTEXT ( ( #8318, #10180, #15595 ) ) REPRESENTATION_CONTEXT ( 'NONE', 'WORKASPACE' ) );
#14180=VERTEX_POINT ( 'NONE', #11163 ) ;
#14181=CARTESIAN_POINT ( 'NONE',  ( -88.14047854185180597, 6.938893903907228378E-15, -30.00000000000000000 ) ) ;
#14183=CARTESIAN_POINT ( 'NONE',  ( -2.057045456857760524, -78.28153924966404986, -12.99038105676658539 ) ) ;
#14185=CYLINDRICAL_SURFACE ( 'NONE', #14805, 1.500000000000001554 ) ;
#14187=AXIS2_PLACEMENT_3D ( 'NONE', #7904, #15196, #3789 ) ;
#14188=DIRECTION ( 'NONE',  ( -0.9876526153536341335, -0.1566598588826327021, 0.000000000000000000 ) ) ;
#14189=DIRECTION ( 'NONE',  ( -0.1566598588826321192, 0.9876526153536342445, 7.798540720466730171E-17 ) ) ;
#14190=VECTOR ( 'NONE', #6526, 1000.000000000000000 ) ;
#14192=ORIENTED_EDGE ( 'NONE', *, *, #12697, .F. ) ;
#14194=ADVANCED_FACE ( 'NONE', ( #3961 ), #12674, .F. ) ;
#14195=CIRCLE ( 'NONE', #3869, 1.499999999999999556 ) ;
#14196=VERTEX_POINT ( 'NONE', #8152 ) ;
#14197=CARTESIAN_POINT ( 'NONE',  ( -43.08426400421126345, -27.08374195694514341, -8.660254037844380193 ) ) ;
#14198=EDGE_LOOP ( 'NONE', ( #3412, #5381 ) ) ;
#14199=ORIENTED_EDGE ( 'NONE', *, *, #18121, .T. ) ;
#14200=ORIENTED_EDGE ( 'NONE', *, *, #14901, .F. ) ;
#14201=AXIS2_PLACEMENT_3D ( 'NONE', #7058, #17190, #8731 ) ;
#14202=CARTESIAN_POINT ( 'NONE',  ( -67.24211807019732134, -88.62108993591775175, 17.32050807568881368 ) ) ;
#14203=AXIS2_PLACEMENT_3D ( 'NONE', #16082, #1591, #72 ) ;
#14204=CARTESIAN_POINT ( 'NONE',  ( -15.22563745336913144, -17.60234297258069347, 21.65063509461101177 ) ) ;
#14205=AXIS2_PLACEMENT_3D ( 'NONE', #10732, #4951, #14736 ) ;
#14206=DIRECTION ( 'NONE',  ( 0.000000000000000000, 0.000000000000000000, 1.000000000000000000 ) ) ;
#14207=CYLINDRICAL_SURFACE ( 'NONE', #15490, 1.500000000000001554 ) ;
#14209=FACE_OUTER_BOUND ( 'NONE', #15003, .T. ) ;
#14210=FACE_OUTER_BOUND ( 'NONE', #9043, .T. ) ;
#14211=CARTESIAN_POINT ( 'NONE',  ( -4.526176995241833367, -78.67318889687062722, 8.660254037844408614 ) ) ;
#14212=ORIENTED_EDGE ( 'NONE', *, *, #14791, .T. ) ;
#14214=AXIS2_PLACEMENT_3D ( 'NONE', #18750, #4298, #3999 ) ;
#14215=AXIS2_PLACEMENT_3D ( 'NONE', #647, #9538, #2327 ) ;
#14216=DIRECTION ( 'NONE',  ( -0.9876526153536341335, -0.1566598588826327021, 0.000000000000000000 ) ) ;
#14217=DIRECTION ( 'NONE',  ( -0.1566598588826321747, 0.9876526153536343555, 0.000000000000000000 ) ) ;
#14218=EDGE_CURVE ( 'NONE', #17604, #3060, #13923, .T. ) ;
#14219=CIRCLE ( 'NONE', #13601, 1.500000000000000888 ) ;
#14221=VECTOR ( 'NONE', #917, 1000.000000000000000 ) ;
#14222=DIRECTION ( 'NONE',  ( -0.9876526153536336894, -0.1566598588826349503, 0.000000000000000000 ) ) ;
#14223=VERTEX_POINT ( 'NONE', #8048 ) ;
#14226=AXIS2_PLACEMENT_3D ( 'NONE', #16644, #432, #17798 ) ;
#14227=EDGE_LOOP ( 'NONE', ( #13487, #17327 ) ) ;
#14230=DIRECTION ( 'NONE',  ( -0.9876526153536341335, -0.1566598588826327021, 0.000000000000000000 ) ) ;
#14231=DIRECTION ( 'NONE',  ( 0.000000000000000000, 0.000000000000000000, 1.000000000000000000 ) ) ;
#14232=VECTOR ( 'NONE', #15658, 1000.000000000000000 ) ;
#14233=DIRECTION ( 'NONE',  ( 0.000000000000000000, 0.000000000000000000, 1.000000000000000000 ) ) ;
#14234=AXIS2_PLACEMENT_3D ( 'NONE', #18560, #7064, #15757 ) ;
#14235=VECTOR ( 'NONE', #6204, 1000.000000000000000 ) ;
#14238=FACE_BOUND ( 'NONE', #6162, .T. ) ;
#14239=CARTESIAN_POINT ( 'NONE',  ( -35.67686938905902849, -25.90879301532540779, -12.99038105676658006 ) ) ;
#14240=DIRECTION ( 'NONE',  ( -0.1566598588826321192, 0.9876526153536342445, 7.798540720466730171E-17 ) ) ;
#14241=CARTESIAN_POINT ( 'NONE',  ( -3.373806069125576901, -15.72242466598909871, 4.330127018922213189 ) ) ;
#14242=AXIS2_PLACEMENT_3D ( 'NONE', #6825, #5390, #7023 ) ;
#14243=ADVANCED_FACE ( 'NONE', ( #15452 ), #18346, .F. ) ;
#14244=CARTESIAN_POINT ( 'NONE',  ( -48.97054468615519340, -85.72288254658904805, 1.424741226644455312E-14 ) ) ;
#14245=EDGE_CURVE ( 'NONE', #730, #14, #6860, .T. ) ;
#14246=VERTEX_POINT ( 'NONE', #18630 ) ;
#14247=CIRCLE ( 'NONE', #3609, 1.500000000000000888 ) ;
#14248=EDGE_LOOP ( 'NONE', ( #4239, #17692 ) ) ;
#14251=ORIENTED_EDGE ( 'NONE', *, *, #15177, .F. ) ;
#14252=CIRCLE ( 'NONE', #6212, 1.500000000000001332 ) ;
#14253=DIRECTION ( 'NONE',  ( -0.9876526153536341335, -0.1566598588826327021, 0.000000000000000000 ) ) ;
#14254=ORIENTED_EDGE ( 'NONE', *, *, #13307, .T. ) ;
#14257=FACE_BOUND ( 'NONE', #12322, .T. ) ;
#14260=LINE ( 'NONE', #15857, #7262 ) ;
#14262=AXIS2_PLACEMENT_3D ( 'NONE', #12926, #17241, #2527 ) ;
#14263=DIRECTION ( 'NONE',  ( -0.1566598588826321192, 0.9876526153536342445, 7.798540720466731404E-17 ) ) ;
#14266=ORIENTED_EDGE ( 'NONE', *, *, #3222, .T. ) ;
#14268=LINE ( 'NONE', #136, #7875 ) ;
#14269=CARTESIAN_POINT ( 'NONE',  ( -74.97862068226375243, -27.08026443497990243, -8.660254037844380193 ) ) ;
#14271=CARTESIAN_POINT ( 'NONE',  ( -3.578159390066044665, -20.81734760163988440, -17.32050807568878170 ) ) ;
#14272=CIRCLE ( 'NONE', #9421, 1.500000000000000888 ) ;
#14275=EDGE_LOOP ( 'NONE', ( #17316, #17464, #15071, #1285 ) ) ;
#14276=ORIENTED_EDGE ( 'NONE', *, *, #3876, .T. ) ;
#14277=DIRECTION ( 'NONE',  ( 0.000000000000000000, 0.000000000000000000, 1.000000000000000000 ) ) ;
#14278=CARTESIAN_POINT ( 'NONE',  ( -8.516422466834198346, -21.60064689605303911, 1.522258424776792809E-14 ) ) ;
#14280=CIRCLE ( 'NONE', #10026, 1.500000000000001332 ) ;
#14281=ORIENTED_EDGE ( 'NONE', *, *, #13149, .T. ) ;
#14283=ORIENTED_EDGE ( 'NONE', *, *, #12856, .T. ) ;
#14284=DIRECTION ( 'NONE',  ( 0.000000000000000000, 0.000000000000000000, 1.000000000000000000 ) ) ;
#14285=AXIS2_PLACEMENT_3D ( 'NONE', #6369, #16491, #863 ) ;
#14286=DIRECTION ( 'NONE',  ( -0.1566598588826321747, 0.9876526153536343555, 0.000000000000000000 ) ) ;
#14287=CIRCLE ( 'NONE', #1867, 1.499999999999999556 ) ;
#14288=ORIENTED_EDGE ( 'NONE', *, *, #15308, .T. ) ;
#14289=CARTESIAN_POINT ( 'NONE',  ( -41.39843176024032800, -21.75382923297043902, 21.65063509461102242 ) ) ;
#14290=CARTESIAN_POINT ( 'NONE',  ( -58.84707083969148300, -87.28948113541537168, 8.660254037844412167 ) ) ;
#14291=EDGE_LOOP ( 'NONE', ( #12540, #618 ) ) ;
#14292=CARTESIAN_POINT ( 'NONE',  ( -21.81009776393036503, -81.41473642731668292, -12.99038105676658539 ) ) ;
#14293=CARTESIAN_POINT ( 'NONE',  ( -25.26688191766805858, -81.96304593340589406, -4.330127018922185655 ) ) ;
#14295=ORIENTED_EDGE ( 'NONE', *, *, #15274, .T. ) ;
#14296=AXIS2_PLACEMENT_3D ( 'NONE', #12647, #839, #5283 ) ;
#14297=LINE ( 'NONE', #1328, #17304 ) ;
#14298=LINE ( 'NONE', #1676, #15123 ) ;
#14299=ORIENTED_EDGE ( 'NONE', *, *, #7421, .T. ) ;
#14302=ORIENTED_EDGE ( 'NONE', *, *, #8088, .F. ) ;
#14303=ORIENTED_EDGE ( 'NONE', *, *, #10244, .T. ) ;
#14304=EDGE_CURVE ( 'NONE', #13246, #11126, #10754, .T. ) ;
#14305=AXIS2_PLACEMENT_3D ( 'NONE', #11558, #11728, #8916 ) ;
#14306=EDGE_CURVE ( 'NONE', #1263, #11861, #3, .T. ) ;
#14307=DIRECTION ( 'NONE',  ( -0.1566598588826321192, 0.9876526153536342445, 7.798540720466730171E-17 ) ) ;
#14308=EDGE_LOOP ( 'NONE', ( #6431, #17661, #691, #1776 ) ) ;
#14309=DIRECTION ( 'NONE',  ( -0.9876526153536341335, -0.1566598588826327021, 0.000000000000000000 ) ) ;
#14310=AXIS2_PLACEMENT_3D ( 'NONE', #14990, #15079, #4658 ) ;
#14311=ADVANCED_FACE ( 'NONE', ( #11622 ), #5691, .F. ) ;
#14312=CARTESIAN_POINT ( 'NONE',  ( -57.36559191666103175, -87.05449134709142811, -8.660254037844385522 ) ) ;
#14318=CARTESIAN_POINT ( 'NONE',  ( -73.49714175923330117, -26.84527464665595886, 1.908195823574487804E-14 ) ) ;
#14319=ORIENTED_EDGE ( 'NONE', *, *, #3693, .F. ) ;
#14320=DIRECTION ( 'NONE',  ( 0.000000000000000000, 0.000000000000000000, 1.000000000000000000 ) ) ;
#14321=DIRECTION ( 'NONE',  ( -0.1566598588826321192, 0.9876526153536342445, 7.798540720466730171E-17 ) ) ;
#14322=EDGE_LOOP ( 'NONE', ( #18743, #7376 ) ) ;
#14323=VERTEX_POINT ( 'NONE', #15831 ) ;
#14324=DIRECTION ( 'NONE',  ( -0.1566598588826321192, 0.9876526153536342445, 7.798540720466730171E-17 ) ) ;
#14325=AXIS2_PLACEMENT_3D ( 'NONE', #3120, #3202, #13437 ) ;
#14326=ORIENTED_EDGE ( 'NONE', *, *, #14131, .F. ) ;
#14327=CYLINDRICAL_SURFACE ( 'NONE', #15918, 1.500000000000001554 ) ;
#14329=DIRECTION ( 'NONE',  ( -0.9876526153536341335, -0.1566598588826327021, 0.000000000000000000 ) ) ;
#14330=FACE_BOUND ( 'NONE', #3708, .T. ) ;
#14332=DIRECTION ( 'NONE',  ( 2.887450008416415878E-16, 0.000000000000000000, 1.000000000000000000 ) ) ;
#14334=DIRECTION ( 'NONE',  ( -0.1566598588826321192, 0.9876526153536342445, 7.798540720466730171E-17 ) ) ;
#14335=EDGE_CURVE ( 'NONE', #6017, #12067, #2837, .T. ) ;
#14336=ORIENTED_EDGE ( 'NONE', *, *, #5448, .F. ) ;
#14338=CARTESIAN_POINT ( 'NONE',  ( -68.72359699322777260, -88.85607972424168111, -17.32050807568878525 ) ) ;
#14339=ORIENTED_EDGE ( 'NONE', *, *, #10421, .F. ) ;
#14340=CARTESIAN_POINT ( 'NONE',  ( -70.04035760549561473, -26.29696514056674062, -17.32050807568878170 ) ) ;
#14341=VERTEX_POINT ( 'NONE', #1429 ) ;
#14342=VERTEX_POINT ( 'NONE', #11348 ) ;
#14343=EDGE_LOOP ( 'NONE', ( #4566, #107 ) ) ;
#14344=DIRECTION ( 'NONE',  ( -0.1566598588826321192, 0.9876526153536342445, 7.798540720466731404E-17 ) ) ;
#14345=VECTOR ( 'NONE', #3650, 1000.000000000000000 ) ;
#14346=ORIENTED_EDGE ( 'NONE', *, *, #13785, .T. ) ;
#14347=FACE_BOUND ( 'NONE', #5174, .T. ) ;
#14348=DIRECTION ( 'NONE',  ( -0.9876526153536336894, -0.1566598588826349503, 0.000000000000000000 ) ) ;
#14349=ORIENTED_EDGE ( 'NONE', *, *, #4150, .T. ) ;
#14351=CARTESIAN_POINT ( 'NONE',  ( -66.25446545484369665, -88.46443007703511796, 12.99038105676661203 ) ) ;
#14352=DIRECTION ( 'NONE',  ( -0.1566598588826321192, 0.9876526153536342445, 7.798540720466730171E-17 ) ) ;
#14356=VERTEX_POINT ( 'NONE', #2911 ) ;
#14357=DIRECTION ( 'NONE',  ( -0.9876526153536336894, -0.1566598588826349503, 0.000000000000000000 ) ) ;
#14358=FACE_BOUND ( 'NONE', #5944, .T. ) ;
#14361=ORIENTED_EDGE ( 'NONE', *, *, #952, .F. ) ;
#14363=DIRECTION ( 'NONE',  ( -0.9876526153536336894, -0.1566598588826349503, 0.000000000000000000 ) ) ;
#14364=VERTEX_POINT ( 'NONE', #8712 ) ;
#14365=DIRECTION ( 'NONE',  ( 0.000000000000000000, 0.000000000000000000, 1.000000000000000000 ) ) ;
#14366=CARTESIAN_POINT ( 'NONE',  ( -55.22556837519115902, -23.94706725732727293, 1.908195823574487804E-14 ) ) ;
#14367=ORIENTED_EDGE ( 'NONE', *, *, #18025, .F. ) ;
#14368=EDGE_CURVE ( 'NONE', #9239, #16068, #18076, .T. ) ;
#14369=ORIENTED_EDGE ( 'NONE', *, *, #7861, .T. ) ;
#14370=ORIENTED_EDGE ( 'NONE', *, *, #2335, .F. ) ;
#14371=CARTESIAN_POINT ( 'NONE',  ( -84.23462711737164454, 33.01666666666666572, 35.00000000000000000 ) ) ;
#14372=CYLINDRICAL_SURFACE ( 'NONE', #9406, 1.500000000000001554 ) ;
#14374=EDGE_CURVE ( 'NONE', #18673, #13460, #17446, .T. ) ;
#14378=LINE ( 'NONE', #8772, #6656 ) ;
#14379=EDGE_CURVE ( 'NONE', #311, #7400, #13145, .T. ) ;
#14380=DIRECTION ( 'NONE',  ( -0.9876526153536341335, -0.1566598588826327576, 0.000000000000000000 ) ) ;
#14381=VERTEX_POINT ( 'NONE', #15726 ) ;
#14383=FACE_OUTER_BOUND ( 'NONE', #11940, .T. ) ;
#14384=LINE ( 'NONE', #16086, #1722 ) ;
#14385=ORIENTED_EDGE ( 'NONE', *, *, #18305, .T. ) ;
#14388=LINE ( 'NONE', #15893, #6039 ) ;
#14389=ORIENTED_EDGE ( 'NONE', *, *, #6436, .F. ) ;
#14390=ORIENTED_EDGE ( 'NONE', *, *, #1612, .F. ) ;
#14391=DIRECTION ( 'NONE',  ( -0.1566598588826321192, 0.9876526153536342445, 7.798540720466730171E-17 ) ) ;
#14392=CIRCLE ( 'NONE', #3465, 1.500000000000001332 ) ;
#14393=CARTESIAN_POINT ( 'NONE',  ( -18.18859529943003750, -18.07232254922858417, 12.99038105676661381 ) ) ;
#14395=DIRECTION ( 'NONE',  ( -0.1566598588826321192, 0.9876526153536342445, 7.798540720466730171E-17 ) ) ;
#14396=ADVANCED_FACE ( 'NONE', ( #11708 ), #17549, .F. ) ;
#14397=DIRECTION ( 'NONE',  ( 0.000000000000000000, 0.000000000000000000, 1.000000000000000000 ) ) ;
#14399=DIRECTION ( 'NONE',  ( -0.1566598588826321192, 0.9876526153536342445, 7.798540720466730171E-17 ) ) ;
#14400=FACE_OUTER_BOUND ( 'NONE', #4489, .T. ) ;
#14401=DIRECTION ( 'NONE',  ( 0.000000000000000000, 0.000000000000000000, 1.000000000000000000 ) ) ;
#14404=DIRECTION ( 'NONE',  ( -0.1566598588826321192, 0.9876526153536342445, 7.798540720466730171E-17 ) ) ;
#14405=EDGE_CURVE ( 'NONE', #306, #17592, #8043, .T. ) ;
#14406=DIRECTION ( 'NONE',  ( -0.9876526153536341335, -0.1566598588826327021, 0.000000000000000000 ) ) ;
#14408=EDGE_LOOP ( 'NONE', ( #14088, #10426 ) ) ;
#14409=DIRECTION ( 'NONE',  ( -0.9876526153536342445, -0.1566598588826321192, -3.168663947239273463E-17 ) ) ;
#14412=CARTESIAN_POINT ( 'NONE',  ( -70.24471092643608472, -31.39188807621751209, 4.330127018922217630 ) ) ;
#14414=LINE ( 'NONE', #7230, #66 ) ;
#14415=DIRECTION ( 'NONE',  ( -0.1566598588826321192, 0.9876526153536342445, 7.798540720466730171E-17 ) ) ;
#14416=LINE ( 'NONE', #6763, #17271 ) ;
#14418=FACE_BOUND ( 'NONE', #1817, .T. ) ;
#14419=ADVANCED_FACE ( 'NONE', ( #1690 ), #7476, .F. ) ;
#14421=CARTESIAN_POINT ( 'NONE',  ( -55.42992169613162190, -29.04199019297804085, 4.330127018922217630 ) ) ;
#14423=CARTESIAN_POINT ( 'NONE',  ( -6.995308533625909320, -79.06483854407721878, 4.330127018922213189 ) ) ;
#14424=FACE_BOUND ( 'NONE', #9946, .T. ) ;
#14426=EDGE_CURVE ( 'NONE', #4160, #4382, #4706, .T. ) ;
#14427=CARTESIAN_POINT ( 'NONE',  ( -4.361458684479201153, -15.87908452487173427, -8.660254037844383745 ) ) ;
#14429=EDGE_LOOP ( 'NONE', ( #13374, #11810 ) ) ;
#14430=ORIENTED_EDGE ( 'NONE', *, *, #10801, .T. ) ;
#14431=DIRECTION ( 'NONE',  ( -0.1566598588826321192, 0.9876526153536342445, 7.798540720466731404E-17 ) ) ;
#14433=ORIENTED_EDGE ( 'NONE', *, *, #13722, .T. ) ;
#14435=DIRECTION ( 'NONE',  ( -0.1566598588826321747, 0.9876526153536343555, 0.000000000000000000 ) ) ;
#14436=ORIENTED_EDGE ( 'NONE', *, *, #1740, .F. ) ;
#14437=AXIS2_PLACEMENT_3D ( 'NONE', #3722, #9523, #5452 ) ;
#14438=CIRCLE ( 'NONE', #7191, 1.499999999999999556 ) ;
#14439=AXIS2_PLACEMENT_3D ( 'NONE', #17643, #15995, #3366 ) ;
#14440=CARTESIAN_POINT ( 'NONE',  ( 0.000000000000000000, 0.000000000000000000, 30.00000000000000000 ) ) ;
#14441=CARTESIAN_POINT ( 'NONE',  ( -75.18297400320422241, -32.17518737063066681, 12.99038105676661736 ) ) ;
#14442=LINE ( 'NONE', #2957, #12998 ) ;
#14444=CARTESIAN_POINT ( 'NONE',  ( -74.19532138785061193, -32.01852751174804013, 1.869203119972154228E-14 ) ) ;
#14446=FACE_OUTER_BOUND ( 'NONE', #16370, .T. ) ;
#14448=CARTESIAN_POINT ( 'NONE',  ( -54.73174206751433957, -23.86873732788595959, -4.330127018922180326 ) ) ;
#14449=EDGE_LOOP ( 'NONE', ( #15121, #7431, #5669, #17228 ) ) ;
#14450=VERTEX_POINT ( 'NONE', #1966 ) ;
#14452=ADVANCED_FACE ( 'NONE', ( #4800 ), #14948, .F. ) ;
#14453=AXIS2_PLACEMENT_3D ( 'NONE', #5551, #17037, #2694 ) ;
#14455=AXIS2_PLACEMENT_3D ( 'NONE', #2119, #7906, #4672 ) ;
#14456=CARTESIAN_POINT ( 'NONE',  ( -53.90880776292333820, -86.50618184100220276, -17.32050807568878525 ) ) ;
#14457=CYLINDRICAL_SURFACE ( 'NONE', #13020, 1.500000000000001554 ) ;
#14458=VERTEX_POINT ( 'NONE', #6159 ) ;
#14459=CARTESIAN_POINT ( 'NONE',  ( -33.00338452973448966, -20.42222043246806962, 21.65063509461101887 ) ) ;
#14461=VECTOR ( 'NONE', #4262, 1000.000000000000000 ) ;
#14462=CARTESIAN_POINT ( 'NONE',  ( 0.000000000000000000, 0.000000000000000000, -30.00000000000000000 ) ) ;
#14463=CARTESIAN_POINT ( 'NONE',  ( -18.18859529943003750, -18.07232254922857706, -21.65063509461098334 ) ) ;
#14464=CIRCLE ( 'NONE', #17829, 1.500000000000000888 ) ;
#14465=CYLINDRICAL_SURFACE ( 'NONE', #9351, 1.500000000000001554 ) ;
#14466=DIRECTION ( 'NONE',  ( -0.9876526153536336894, -0.1566598588826349503, 0.000000000000000000 ) ) ;
#14467=CARTESIAN_POINT ( 'NONE',  ( -8.312069145893737243, -16.50572396040226053, -21.65063509461098334 ) ) ;
#14468=VERTEX_POINT ( 'NONE', #16195 ) ;
#14469=CARTESIAN_POINT ( 'NONE',  ( -14.44233815895597672, -22.54060604934882051, -12.99038105676658006 ) ) ;
#14470=AXIS2_PLACEMENT_3D ( 'NONE', #4623, #17732, #16112 ) ;
#14471=EDGE_LOOP ( 'NONE', ( #12151, #18710, #1100, #9489 ) ) ;
#14472=DIRECTION ( 'NONE',  ( -0.1566598588826321747, 0.9876526153536343555, 0.000000000000000000 ) ) ;
#14474=ADVANCED_FACE ( 'NONE', ( #3555 ), #18018, .F. ) ;
#14476=ADVANCED_FACE ( 'NONE', ( #15038 ), #10681, .F. ) ;
#14477=DIRECTION ( 'NONE',  ( 0.000000000000000000, 0.000000000000000000, 1.000000000000000000 ) ) ;
#14478=ORIENTED_EDGE ( 'NONE', *, *, #8806, .T. ) ;
#14479=ADVANCED_FACE ( 'NONE', ( #4976 ), #9355, .F. ) ;
#14480=ORIENTED_EDGE ( 'NONE', *, *, #8703, .T. ) ;
#14482=ORIENTED_EDGE ( 'NONE', *, *, #7081, .T. ) ;
#14483=DIRECTION ( 'NONE',  ( -0.1566598588826321192, 0.9876526153536342445, 7.798540720466731404E-17 ) ) ;
#14486=ORIENTED_EDGE ( 'NONE', *, *, #10638, .F. ) ;
#14487=CARTESIAN_POINT ( 'NONE',  ( -2.879979761448749009, -15.64409473654778893, -17.32050807568878170 ) ) ;
#14488=CARTESIAN_POINT ( 'NONE',  ( -10.28737437660098131, -16.81904367816753165, -4.330127018922180326 ) ) ;
#14489=CIRCLE ( 'NONE', #13263, 1.500000000000000888 ) ;
#14490=CYLINDRICAL_SURFACE ( 'NONE', #9375, 1.500000000000001554 ) ;
#14492=AXIS2_PLACEMENT_3D ( 'NONE', #11189, #17013, #3985 ) ;
#14493=ORIENTED_EDGE ( 'NONE', *, *, #7308, .F. ) ;
#14494=CARTESIAN_POINT ( 'NONE',  ( -21.64537945316773460, -18.62063205531779886, 21.65063509461101532 ) ) ;
#14496=DIRECTION ( 'NONE',  ( -0.9876526153536336894, -0.1566598588826349503, 0.000000000000000000 ) ) ;
#14497=DIRECTION ( 'NONE',  ( -0.1566598588826321747, 0.9876526153536343555, 0.000000000000000000 ) ) ;
#14499=DIRECTION ( 'NONE',  ( -0.1566598588826321747, 0.9876526153536343555, 0.000000000000000000 ) ) ;
#14500=ORIENTED_EDGE ( 'NONE', *, *, #14580, .T. ) ;
#14501=EDGE_CURVE ( 'NONE', #13816, #1601, #7763, .T. ) ;
#14502=ORIENTED_EDGE ( 'NONE', *, *, #10746, .T. ) ;
#14503=CARTESIAN_POINT ( 'NONE',  ( -59.38053215754616332, -29.66862962850856533, -17.32050807568878170 ) ) ;
#14504=AXIS2_PLACEMENT_3D ( 'NONE', #18739, #12708, #18563 ) ;
#14506=ORIENTED_EDGE ( 'NONE', *, *, #12149, .F. ) ;
#14507=CYLINDRICAL_SURFACE ( 'NONE', #8052, 1.500000000000000666 ) ;
#14508=VECTOR ( 'NONE', #15320, 1000.000000000000000 ) ;
#14509=EDGE_CURVE ( 'NONE', #719, #8415, #8960, .T. ) ;
#14510=VECTOR ( 'NONE', #7221, 1000.000000000000000 ) ;
#14511=DIRECTION ( 'NONE',  ( 0.9876526153536342445, 0.1566598588826321192, 0.000000000000000000 ) ) ;
#14512=ORIENTED_EDGE ( 'NONE', *, *, #14539, .T. ) ;
#14514=CIRCLE ( 'NONE', #8755, 1.500000000000000888 ) ;
#14515=CIRCLE ( 'NONE', #11167, 1.500000000000000888 ) ;
#14516=FACE_OUTER_BOUND ( 'NONE', #1111, .T. ) ;
#14517=VERTEX_POINT ( 'NONE', #17931 ) ;
#14518=AXIS2_PLACEMENT_3D ( 'NONE', #14928, #3627, #9433 ) ;
#14520=VERTEX_POINT ( 'NONE', #10395 ) ;
#14521=DIRECTION ( 'NONE',  ( 1.000000000000000000, 0.000000000000000000, 0.000000000000000000 ) ) ;
#14522=CIRCLE ( 'NONE', #6364, 1.500000000000000888 ) ;
#14525=CYLINDRICAL_SURFACE ( 'NONE', #3897, 1.500000000000001554 ) ;
#14526=FACE_BOUND ( 'NONE', #6778, .T. ) ;
#14527=DIRECTION ( 'NONE',  ( -0.1566598588826321192, 0.9876526153536342445, 7.798540720466731404E-17 ) ) ;
#14531=VERTEX_POINT ( 'NONE', #3462 ) ;
#14532=CARTESIAN_POINT ( 'NONE',  ( -38.14600092744309734, -26.30044266253198160, 1.175313729581431390E-14 ) ) ;
#14533=VERTEX_POINT ( 'NONE', #8974 ) ;
#14534=VECTOR ( 'NONE', #3065, 1000.000000000000000 ) ;
#14535=FACE_BOUND ( 'NONE', #7741, .T. ) ;
#14536=ADVANCED_FACE ( 'NONE', ( #2160 ), #4897, .F. ) ;
#14537=CARTESIAN_POINT ( 'NONE',  ( -3.538524379888208227, -78.51652903798800764, 12.99038105676660848 ) ) ;
#14538=AXIS2_PLACEMENT_3D ( 'NONE', #18758, #10442, #10537 ) ;
#14539=EDGE_CURVE ( 'NONE', #8813, #16572, #17470, .T. ) ;
#14540=ORIENTED_EDGE ( 'NONE', *, *, #2559, .F. ) ;
#14543=ORIENTED_EDGE ( 'NONE', *, *, #15297, .F. ) ;
#14545=AXIS2_PLACEMENT_3D ( 'NONE', #18652, #4179, #9964 ) ;
#14546=CARTESIAN_POINT ( 'NONE',  ( -88.14047854185180597, -33.59999999999994458, -24.99999999999999645 ) ) ;
#14548=AXIS2_PLACEMENT_3D ( 'NONE', #5021, #12603, #9501 ) ;
#14550=ORIENTED_EDGE ( 'NONE', *, *, #8815, .F. ) ;
#14551=EDGE_LOOP ( 'NONE', ( #5375, #9601 ) ) ;
#14552=CARTESIAN_POINT ( 'NONE',  ( -8.312069145893737243, -16.50572396040226053, 4.330127018922214965 ) ) ;
#14553=DIRECTION ( 'NONE',  ( -0.9876526153536336894, -0.1566598588826349503, 0.000000000000000000 ) ) ;
#14555=EDGE_LOOP ( 'NONE', ( #13709, #7352, #11970, #9316 ) ) ;
#14556=CARTESIAN_POINT ( 'NONE',  ( -57.85941822433786541, -87.13282127653275211, 12.99038105676661203 ) ) ;
#14557=FACE_BOUND ( 'NONE', #1013, .T. ) ;
#14558=EDGE_CURVE ( 'NONE', #6040, #17749, #9272, .T. ) ;
#14559=DIRECTION ( 'NONE',  ( 0.000000000000000000, 0.000000000000000000, 1.000000000000000000 ) ) ;
#14560=AXIS2_PLACEMENT_3D ( 'NONE', #8947, #1582, #6019 ) ;
#14561=ORIENTED_EDGE ( 'NONE', *, *, #10177, .T. ) ;
#14562=DIRECTION ( 'NONE',  ( -0.1566598588826321747, 0.9876526153536343555, 0.000000000000000000 ) ) ;
#14563=CARTESIAN_POINT ( 'NONE',  ( -79.91688375903190433, -27.86356372939306425, 1.908195823574487804E-14 ) ) ;
#14564=EDGE_CURVE ( 'NONE', #12921, #13088, #4426, .T. ) ;
#14566=CARTESIAN_POINT ( 'NONE',  ( -10.94591899504043830, -79.69147797960773971, -17.32050807568878525 ) ) ;
#14568=ORIENTED_EDGE ( 'NONE', *, *, #5125, .F. ) ;
#14569=DIRECTION ( 'NONE',  ( -0.1566598588826321747, 0.9876526153536343555, 0.000000000000000000 ) ) ;
#14570=ORIENTED_EDGE ( 'NONE', *, *, #11353, .T. ) ;
#14571=AXIS2_PLACEMENT_3D ( 'NONE', #5629, #2678, #1458 ) ;
#14572=ORIENTED_EDGE ( 'NONE', *, *, #5661, .T. ) ;
#14573=ORIENTED_EDGE ( 'NONE', *, *, #16560, .F. ) ;
#14574=VECTOR ( 'NONE', #4866, 1000.000000000000000 ) ;
#14577=VECTOR ( 'NONE', #5681, 1000.000000000000000 ) ;
#14578=AXIS2_PLACEMENT_3D ( 'NONE', #995, #6766, #5133 ) ;
#14580=EDGE_CURVE ( 'NONE', #1802, #10598, #1881, .T. ) ;
#14581=CARTESIAN_POINT ( 'NONE',  ( -56.91140061916208026, -29.27697998130198442, 4.330127018922217630 ) ) ;
#14582=VERTEX_POINT ( 'NONE', #13509 ) ;
#14583=FACE_OUTER_BOUND ( 'NONE', #14449, .T. ) ;
#14584=DIRECTION ( 'NONE',  ( -0.1566598588826321192, 0.9876526153536342445, 7.798540720466730171E-17 ) ) ;
#14585=FACE_OUTER_BOUND ( 'NONE', #18786, .T. ) ;
#14586=VECTOR ( 'NONE', #2907, 1000.000000000000000 ) ;
#14588=DIRECTION ( 'NONE',  ( -0.1566598588826321192, 0.9876526153536342445, 7.798540720466730171E-17 ) ) ;
#14589=ADVANCED_FACE ( 'NONE', ( #16781 ), #9457, .F. ) ;
#14591=DIRECTION ( 'NONE',  ( -0.1566598588826321192, 0.9876526153536342445, 7.798540720466731404E-17 ) ) ;
#14593=EDGE_CURVE ( 'NONE', #5983, #7813, #14000, .T. ) ;
#14595=AXIS2_PLACEMENT_3D ( 'NONE', #16334, #16438, #10261 ) ;
#14598=ORIENTED_EDGE ( 'NONE', *, *, #9879, .T. ) ;
#14599=VERTEX_POINT ( 'NONE', #1050 ) ;
#14600=CARTESIAN_POINT ( 'NONE',  ( -47.32434745236212592, -22.69378838626621686, -17.32050807568878170 ) ) ;
#14602=EDGE_LOOP ( 'NONE', ( #14771, #13880, #13167, #9695 ) ) ;
#14603=PLANE ( 'NONE',  #17641 ) ;
#14604=ORIENTED_EDGE ( 'NONE', *, *, #14709, .T. ) ;
#14605=DIRECTION ( 'NONE',  ( -0.1566598588826321192, 0.9876526153536342445, 7.798540720466730171E-17 ) ) ;
#14608=EDGE_CURVE ( 'NONE', #6818, #10150, #12272, .T. ) ;
#14609=ADVANCED_FACE ( 'NONE', ( #9832 ), #5384, .F. ) ;
#14610=ADVANCED_FACE ( 'NONE', ( #15598 ), #8232, .F. ) ;
#14611=DIRECTION ( 'NONE',  ( 0.000000000000000000, 0.000000000000000000, 1.000000000000000000 ) ) ;
#14612=VERTEX_POINT ( 'NONE', #11139 ) ;
#14614=ORIENTED_EDGE ( 'NONE', *, *, #3653, .F. ) ;
#14615=AXIS2_PLACEMENT_3D ( 'NONE', #7794, #14802, #6199 ) ;
#14617=DIRECTION ( 'NONE',  ( -0.9876526153536344665, -0.1566598588826304539, 0.000000000000000000 ) ) ;
#14618=DIRECTION ( 'NONE',  ( -0.9876526153536336894, -0.1566598588826349503, 0.000000000000000000 ) ) ;
#14619=CARTESIAN_POINT ( 'NONE',  ( -63.82496892663746735, -30.37359899348040315, -21.65063509461098334 ) ) ;
#14620=VERTEX_POINT ( 'NONE', #2337 ) ;
#14621=ORIENTED_EDGE ( 'NONE', *, *, #4644, .T. ) ;
#14623=ORIENTED_EDGE ( 'NONE', *, *, #17924, .T. ) ;
#14624=DIRECTION ( 'NONE',  ( -0.1566598588826321192, 0.9876526153536342445, 7.798540720466731404E-17 ) ) ;
#14625=EDGE_LOOP ( 'NONE', ( #9019, #18569 ) ) ;
#14627=VERTEX_POINT ( 'NONE', #946 ) ;
#14629=ORIENTED_EDGE ( 'NONE', *, *, #16052, .F. ) ;
#14630=AXIS2_PLACEMENT_3D ( 'NONE', #6741, #8144, #4989 ) ;
#14631=ORIENTED_EDGE ( 'NONE', *, *, #5189, .F. ) ;
#14632=DIRECTION ( 'NONE',  ( -0.1566598588826321747, 0.9876526153536343555, 0.000000000000000000 ) ) ;
#14633=CARTESIAN_POINT ( 'NONE',  ( -40.08167114797252140, -84.31294381664535820, -21.65063509461098690 ) ) ;
#14634=LINE ( 'NONE', #4305, #2418 ) ;
#14635=CARTESIAN_POINT ( 'NONE',  ( 3.231158466157554976, 19.73726462726228092, 24.99999999999999289 ) ) ;
#14638=CARTESIAN_POINT ( 'NONE',  ( -29.75095369693726610, -24.96883386202961574, 8.660254037844417496 ) ) ;
#14639=EDGE_LOOP ( 'NONE', ( #13730, #7242, #16053, #1983 ) ) ;
#14640=EDGE_CURVE ( 'NONE', #886, #4810, #11074, .T. ) ;
#14641=EDGE_LOOP ( 'NONE', ( #8419, #5466 ) ) ;
#14644=EDGE_LOOP ( 'NONE', ( #1999, #1500 ) ) ;
#14645=CARTESIAN_POINT ( 'NONE',  ( 1.360103686702108128, -20.03404830722672259, 1.348786077179111942E-14 ) ) ;
#14646=DIRECTION ( 'NONE',  ( -0.9876526153536341335, -0.1566598588826327021, 0.000000000000000000 ) ) ;
#14647=VERTEX_POINT ( 'NONE', #6913 ) ;
#14648=ORIENTED_EDGE ( 'NONE', *, *, #16453, .T. ) ;
#14650=CARTESIAN_POINT ( 'NONE',  ( -47.48906576312474215, -85.48789275826510448, 1.443110928631665584E-14 ) ) ;
#14651=CARTESIAN_POINT ( 'NONE',  ( -16.87183468716221313, -80.63143713290354242, 21.65063509461101532 ) ) ;
#14652=DIRECTION ( 'NONE',  ( -0.1566598588826321192, 0.9876526153536342445, 7.798540720466730171E-17 ) ) ;
#14653=ADVANCED_FACE ( 'NONE', ( #842 ), #10853, .F. ) ;
#14654=DIRECTION ( 'NONE',  ( -0.1566598588826321747, 0.9876526153536343555, 0.000000000000000000 ) ) ;
#14655=CARTESIAN_POINT ( 'NONE',  ( -65.30644784966793281, -30.60858878180435738, -12.99038105676658006 ) ) ;
#14656=ORIENTED_EDGE ( 'NONE', *, *, #8530, .F. ) ;
#14657=ORIENTED_EDGE ( 'NONE', *, *, #5520, .T. ) ;
#14659=ORIENTED_EDGE ( 'NONE', *, *, #6674, .T. ) ;
#14660=EDGE_CURVE ( 'NONE', #16376, #11672, #11372, .T. ) ;
#14661=DIRECTION ( 'NONE',  ( -0.1566598588826321747, 0.9876526153536343555, 0.000000000000000000 ) ) ;
#14662=VERTEX_POINT ( 'NONE', #16869 ) ;
#14663=ORIENTED_EDGE ( 'NONE', *, *, #5216, .T. ) ;
#14664=CIRCLE ( 'NONE', #4669, 1.500000000000000000 ) ;
#14665=FACE_OUTER_BOUND ( 'NONE', #3319, .T. ) ;
#14666=CARTESIAN_POINT ( 'NONE',  ( -55.42992169613163611, -29.04199019297804085, -4.330127018922181215 ) ) ;
#14667=CARTESIAN_POINT ( 'NONE',  ( -56.37793930130741415, -86.89783148820879433, -21.65063509461098690 ) ) ;
#14669=CYLINDRICAL_SURFACE ( 'NONE', #10335, 1.500000000000001554 ) ;
#14671=CARTESIAN_POINT ( 'NONE',  ( -42.38608437559395270, -21.91048909185307281, 17.32050807568881723 ) ) ;
#14672=DIRECTION ( 'NONE',  ( -0.1566598588826321192, 0.9876526153536342445, 7.798540720466730171E-17 ) ) ;
#14673=DIRECTION ( 'NONE',  ( 0.000000000000000000, 0.000000000000000000, 1.000000000000000000 ) ) ;
#14674=DIRECTION ( 'NONE',  ( -0.9876526153536341335, -0.1566598588826327021, 0.000000000000000000 ) ) ;
#14675=AXIS2_PLACEMENT_3D ( 'NONE', #3165, #14741, #1758 ) ;
#14677=ORIENTED_EDGE ( 'NONE', *, *, #2828, .T. ) ;
#14678=ORIENTED_EDGE ( 'NONE', *, *, #489, .T. ) ;
#14679=EDGE_LOOP ( 'NONE', ( #18369, #5673, #4317, #4357 ) ) ;
#14680=DIRECTION ( 'NONE',  ( -0.1566598588826321192, 0.9876526153536342445, 7.798540720466730171E-17 ) ) ;
#14681=ORIENTED_EDGE ( 'NONE', *, *, #14068, .T. ) ;
#14682=ADVANCED_FACE ( 'NONE', ( #3655 ), #18223, .F. ) ;
#14684=VERTEX_POINT ( 'NONE', #3835 ) ;
#14685=CARTESIAN_POINT ( 'NONE',  ( 1.360103686702108128, -20.03404830722672259, -8.660254037844383745 ) ) ;
#14686=FACE_OUTER_BOUND ( 'NONE', #5827, .T. ) ;
#14687=EDGE_CURVE ( 'NONE', #17456, #697, #3198, .T. ) ;
#14688=CARTESIAN_POINT ( 'NONE',  ( -3.578159390066044665, -20.81734760163988440, 17.32050807568881012 ) ) ;
#14689=FACE_OUTER_BOUND ( 'NONE', #13025, .T. ) ;
#14692=EDGE_LOOP ( 'NONE', ( #13260, #521 ) ) ;
#14696=CARTESIAN_POINT ( 'NONE',  ( -6.047290928450125946, -21.20899724884646531, 4.330127018922214077 ) ) ;
#14698=CARTESIAN_POINT ( 'NONE',  ( -35.63723437888118184, -83.60797445167352748, 8.660254037844412167 ) ) ;
#14699=VECTOR ( 'NONE', #14672, 1000.000000000000000 ) ;
#14701=ORIENTED_EDGE ( 'NONE', *, *, #14705, .T. ) ;
#14702=ORIENTED_EDGE ( 'NONE', *, *, #14813, .T. ) ;
#14703=VERTEX_POINT ( 'NONE', #9754 ) ;
#14704=FACE_OUTER_BOUND ( 'NONE', #3156, .T. ) ;
#14705=EDGE_CURVE ( 'NONE', #10784, #11150, #14115, .T. ) ;
#14706=EDGE_CURVE ( 'NONE', #16580, #15439, #12587, .T. ) ;
#14707=ORIENTED_EDGE ( 'NONE', *, *, #11287, .T. ) ;
#14708=FACE_BOUND ( 'NONE', #7840, .T. ) ;
#14709=EDGE_CURVE ( 'NONE', #14890, #10439, #2906, .T. ) ;
#14710=DIRECTION ( 'NONE',  ( 0.000000000000000000, 0.000000000000000000, 1.000000000000000000 ) ) ;
#14712=DIRECTION ( 'NONE',  ( -0.1566598588826321192, 0.9876526153536342445, 7.798540720466731404E-17 ) ) ;
#14714=ORIENTED_EDGE ( 'NONE', *, *, #10612, .F. ) ;
#14715=CARTESIAN_POINT ( 'NONE',  ( -37.44782129882580080, -21.12718979743991454, 17.32050807568881723 ) ) ;
#14716=DIRECTION ( 'NONE',  ( -0.1566598588826321192, 0.9876526153536342445, 7.798540720466731404E-17 ) ) ;
#14717=CARTESIAN_POINT ( 'NONE',  ( -37.44782129882580080, -21.12718979743988967, 1.232676135170975081E-14 ) ) ;
#14719=VERTEX_POINT ( 'NONE', #5575 ) ;
#14720=VERTEX_POINT ( 'NONE', #5774 ) ;
#14721=LINE ( 'NONE', #620, #12334 ) ;
#14722=VECTOR ( 'NONE', #10894, 1000.000000000000000 ) ;
#14723=CARTESIAN_POINT ( 'NONE',  ( 0.000000000000000000, 0.000000000000000000, 30.00000000000000000 ) ) ;
#14724=ADVANCED_FACE ( 'NONE', ( #7015 ), #7108, .F. ) ;
#14725=CARTESIAN_POINT ( 'NONE',  ( -52.92115514756972061, -86.34952198211958319, -12.99038105676658539 ) ) ;
#14726=EDGE_CURVE ( 'NONE', #16165, #9184, #10287, .T. ) ;
#14727=EDGE_CURVE ( 'NONE', #384, #13798, #13203, .T. ) ;
#14728=AXIS2_PLACEMENT_3D ( 'NONE', #16280, #6247, #16391 ) ;
#14729=ORIENTED_EDGE ( 'NONE', *, *, #8730, .F. ) ;
#14730=DIRECTION ( 'NONE',  ( -0.1566598588826321747, 0.9876526153536343555, 0.000000000000000000 ) ) ;
#14732=EDGE_CURVE ( 'NONE', #11672, #16376, #13489, .T. ) ;
#14734=FACE_OUTER_BOUND ( 'NONE', #1305, .T. ) ;
#14735=CIRCLE ( 'NONE', #17186, 1.500000000000000000 ) ;
#14736=DIRECTION ( 'NONE',  ( -0.9876526153536341335, -0.1566598588826327021, 0.000000000000000000 ) ) ;
#14737=DIRECTION ( 'NONE',  ( -0.1566598588826321192, 0.9876526153536342445, 7.798540720466730171E-17 ) ) ;
#14738=AXIS2_PLACEMENT_3D ( 'NONE', #6325, #6136, #4956 ) ;
#14740=AXIS2_PLACEMENT_3D ( 'NONE', #1699, #17662, #1887 ) ;
#14741=DIRECTION ( 'NONE',  ( -0.1566598588826321192, 0.9876526153536342445, 7.798540720466731404E-17 ) ) ;
#14742=DIRECTION ( 'NONE',  ( -0.1566598588826321192, 0.9876526153536342445, 7.798540720466730171E-17 ) ) ;
#14743=VERTEX_POINT ( 'NONE', #12759 ) ;
#14744=ORIENTED_EDGE ( 'NONE', *, *, #3923, .T. ) ;
#14748=AXIS2_PLACEMENT_3D ( 'NONE', #1055, #17256, #18323 ) ;
#14751=DIRECTION ( 'NONE',  ( -0.9876526153536341335, -0.1566598588826327021, 0.000000000000000000 ) ) ;
#14752=EDGE_CURVE ( 'NONE', #1621, #18515, #16234, .T. ) ;
#14753=AXIS2_PLACEMENT_3D ( 'NONE', #18469, #5432, #8187 ) ;
#14755=EDGE_CURVE ( 'NONE', #16874, #11180, #10100, .T. ) ;
#14756=CARTESIAN_POINT ( 'NONE',  ( -61.15148406731293562, -24.88702641062305787, -12.99038105676658006 ) ) ;
#14758=CARTESIAN_POINT ( 'NONE',  ( -5.513829610595458064, -78.82984875575326100, -4.330127018922185655 ) ) ;
#14759=DIRECTION ( 'NONE',  ( 1.000000000000000000, 0.000000000000000000, 0.000000000000000000 ) ) ;
#14760=VERTEX_POINT ( 'NONE', #17145 ) ;
#14761=EDGE_CURVE ( 'NONE', #2452, #1415, #8056, .T. ) ;
#14762=VECTOR ( 'NONE', #11623, 1000.000000000000000 ) ;
#14763=DIRECTION ( 'NONE',  ( -0.1566598588826321747, 0.9876526153536343555, 0.000000000000000000 ) ) ;
#14764=VERTEX_POINT ( 'NONE', #1230 ) ;
#14765=CARTESIAN_POINT ( 'NONE',  ( -36.46016868347218320, -20.97052993855727721, 12.99038105676661736 ) ) ;
#14766=LINE ( 'NONE', #5, #6317 ) ;
#14767=DIRECTION ( 'NONE',  ( -0.9876526153536344665, -0.1566598588826304539, 0.000000000000000000 ) ) ;
#14770=CIRCLE ( 'NONE', #17516, 1.499999999999997335 ) ;
#14771=ORIENTED_EDGE ( 'NONE', *, *, #15365, .F. ) ;
#14774=ORIENTED_EDGE ( 'NONE', *, *, #16184, .T. ) ;
#14775=DIRECTION ( 'NONE',  ( -0.1566598588826321192, 0.9876526153536342445, 7.798540720466731404E-17 ) ) ;
#14776=AXIS2_PLACEMENT_3D ( 'NONE', #7718, #17787, #2021 ) ;
#14779=CARTESIAN_POINT ( 'NONE',  ( -48.97054468615517919, -85.72288254658904805, 8.660254037844412167 ) ) ;
#14783=CARTESIAN_POINT ( 'NONE',  ( -63.82496892663746735, -30.37359899348040315, -4.330127018922181215 ) ) ;
#14784=DIRECTION ( 'NONE',  ( 3.208277787129350839E-17, 0.000000000000000000, -1.000000000000000000 ) ) ;
#14786=ORIENTED_EDGE ( 'NONE', *, *, #8322, .F. ) ;
#14788=EDGE_LOOP ( 'NONE', ( #5720, #16924, #9548, #1304 ) ) ;
#14790=AXIS2_PLACEMENT_3D ( 'NONE', #1004, #6576, #12230 ) ;
#14791=EDGE_CURVE ( 'NONE', #11499, #10533, #7470, .T. ) ;
#14793=DIRECTION ( 'NONE',  ( -0.1566598588826321192, 0.9876526153536342445, 7.798540720466730171E-17 ) ) ;
#14794=EDGE_LOOP ( 'NONE', ( #15408, #9880 ) ) ;
#14795=ORIENTED_EDGE ( 'NONE', *, *, #13796, .T. ) ;
#14796=VERTEX_POINT ( 'NONE', #2722 ) ;
#14797=EDGE_LOOP ( 'NONE', ( #21, #9839 ) ) ;
#14798=VERTEX_POINT ( 'NONE', #2891 ) ;
#14800=FACE_BOUND ( 'NONE', #18690, .T. ) ;
#14801=EDGE_LOOP ( 'NONE', ( #14192, #12207, #1529, #12598 ) ) ;
#14802=DIRECTION ( 'NONE',  ( -0.1566598588826321192, 0.9876526153536342445, 7.798540720466731404E-17 ) ) ;
#14803=CIRCLE ( 'NONE', #906, 1.500000000000000888 ) ;
#14804=ORIENTED_EDGE ( 'NONE', *, *, #12447, .T. ) ;
#14805=AXIS2_PLACEMENT_3D ( 'NONE', #8126, #8514, #12480 ) ;
#14806=AXIS2_PLACEMENT_3D ( 'NONE', #15882, #11775, #4406 ) ;
#14809=ADVANCED_FACE ( 'NONE', ( #8515 ), #7287, .F. ) ;
#14810=DIRECTION ( 'NONE',  ( -0.1566598588826321192, 0.9876526153536342445, 7.798540720466730171E-17 ) ) ;
#14811=CARTESIAN_POINT ( 'NONE',  ( 7.819480696678551723, -76.71494066083772623, -12.99038105676658894 ) ) ;
#14813=EDGE_CURVE ( 'NONE', #6687, #10467, #12850, .T. ) ;
#14814=VECTOR ( 'NONE', #6662, 1000.000000000000000 ) ;
#14815=CYLINDRICAL_SURFACE ( 'NONE', #2881, 1.500000000000001554 ) ;
#14816=CIRCLE ( 'NONE', #1805, 1.500000000000000444 ) ;
#14817=CARTESIAN_POINT ( 'NONE',  ( -21.81009776393036503, -81.41473642731668292, -4.330127018922185655 ) ) ;
#14820=DIRECTION ( 'NONE',  ( -0.9876526153536336894, -0.1566598588826349503, 0.000000000000000000 ) ) ;
#14823=DIRECTION ( 'NONE',  ( 0.000000000000000000, 0.000000000000000000, 1.000000000000000000 ) ) ;
#14824=ORIENTED_EDGE ( 'NONE', *, *, #8118, .T. ) ;
#14825=CIRCLE ( 'NONE', #13590, 1.500000000000000888 ) ;
#14827=EDGE_LOOP ( 'NONE', ( #14900, #14863, #17573, #15080 ) ) ;
#14829=CARTESIAN_POINT ( 'NONE',  ( -31.72625892764450484, -25.28215357979487266, -17.32050807568878170 ) ) ;
#14830=VECTOR ( 'NONE', #2051, 1000.000000000000000 ) ;
#14831=CARTESIAN_POINT ( 'NONE',  ( -68.76323200340563346, -31.15689828789355786, 21.65063509461101887 ) ) ;
#14837=FACE_OUTER_BOUND ( 'NONE', #2181, .T. ) ;
#14838=AXIS2_PLACEMENT_3D ( 'NONE', #17381, #1710, #16301 ) ;
#14840=CARTESIAN_POINT ( 'NONE',  ( -62.30385499342917655, -87.83779064150456861, -17.32050807568878525 ) ) ;
#14841=VERTEX_POINT ( 'NONE', #17426 ) ;
#14843=ORIENTED_EDGE ( 'NONE', *, *, #8815, .T. ) ;
#14844=CIRCLE ( 'NONE', #11207, 1.499999999999997335 ) ;
#14846=ORIENTED_EDGE ( 'NONE', *, *, #3117, .T. ) ;
#14848=CARTESIAN_POINT ( 'NONE',  ( -56.21322099054477661, -24.10372711620990671, 4.330127018922218518 ) ) ;
#14849=AXIS2_PLACEMENT_3D ( 'NONE', #235, #8868, #13206 ) ;
#14850=CARTESIAN_POINT ( 'NONE',  ( -20.82244514857674389, -81.25807656843406335, 8.660254037844412167 ) ) ;
#14851=CYLINDRICAL_SURFACE ( 'NONE', #12818, 1.500000000000000888 ) ;
#14852=DIRECTION ( 'NONE',  ( -0.1566598588826321192, 0.9876526153536342445, 7.798540720466730171E-17 ) ) ;
#14854=DIRECTION ( 'NONE',  ( 0.000000000000000000, 0.000000000000000000, 1.000000000000000000 ) ) ;
#14855=LINE ( 'NONE', #13612, #16617 ) ;
#14856=VECTOR ( 'NONE', #5175, 1000.000000000000000 ) ;
#14857=DIRECTION ( 'NONE',  ( -0.1566598588826321192, 0.9876526153536342445, 7.798540720466730171E-17 ) ) ;
#14858=CARTESIAN_POINT ( 'NONE',  ( -56.37793930130741415, -86.89783148820879433, -4.330127018922185655 ) ) ;
#14859=CIRCLE ( 'NONE', #3958, 1.500000000000000444 ) ;
#14860=CARTESIAN_POINT ( 'NONE',  ( -47.48906576312472794, -85.48789275826511869, 17.32050807568881368 ) ) ;
#14861=ORIENTED_EDGE ( 'NONE', *, *, #134, .T. ) ;
#14862=EDGE_CURVE ( 'NONE', #6605, #14531, #2985, .T. ) ;
#14863=ORIENTED_EDGE ( 'NONE', *, *, #14894, .F. ) ;
#14864=EDGE_CURVE ( 'NONE', #1820, #2692, #4229, .T. ) ;
#14866=ORIENTED_EDGE ( 'NONE', *, *, #316, .F. ) ;
#14867=CIRCLE ( 'NONE', #1858, 1.500000000000000444 ) ;
#14868=ORIENTED_EDGE ( 'NONE', *, *, #15415, .F. ) ;
#14869=CIRCLE ( 'NONE', #12444, 1.500000000000000444 ) ;
#14870=DIRECTION ( 'NONE',  ( -0.9876526153536341335, -0.1566598588826327576, 0.000000000000000000 ) ) ;
#14871=CARTESIAN_POINT ( 'NONE',  ( 2.881217619910392269, -77.49823995525089515, -12.99038105676658539 ) ) ;
#14873=FACE_OUTER_BOUND ( 'NONE', #18201, .T. ) ;
#14874=DIRECTION ( 'NONE',  ( 0.000000000000000000, 0.000000000000000000, 1.000000000000000000 ) ) ;
#14875=DIRECTION ( 'NONE',  ( -0.1566598588826321192, 0.9876526153536342445, 7.798540720466731404E-17 ) ) ;
#14878=CARTESIAN_POINT ( 'NONE',  ( -26.74836084069850983, -82.19803572172985184, -4.330127018922185655 ) ) ;
#14879=CARTESIAN_POINT ( 'NONE',  ( -63.82496892663746735, -30.37359899348039605, 21.65063509461101887 ) ) ;
#14880=CARTESIAN_POINT ( 'NONE',  ( -77.44775222064782838, -27.47191408218647624, -21.65063509461098334 ) ) ;
#14881=DIRECTION ( 'NONE',  ( 0.000000000000000000, 0.000000000000000000, 1.000000000000000000 ) ) ;
#14882=ORIENTED_EDGE ( 'NONE', *, *, #9856, .F. ) ;
#14883=AXIS2_PLACEMENT_3D ( 'NONE', #10617, #2087, #771 ) ;
#14884=CARTESIAN_POINT ( 'NONE',  ( -61.15148406731293562, -24.88702641062305432, -21.65063509461097979 ) ) ;
#14885=ORIENTED_EDGE ( 'NONE', *, *, #5377, .T. ) ;
#14886=DIRECTION ( 'NONE',  ( -0.1566598588826321192, 0.9876526153536342445, 7.798540720466730171E-17 ) ) ;
#14887=CARTESIAN_POINT ( 'NONE',  ( -40.61513246582718040, -26.69209230973856251, 4.330127018922217630 ) ) ;
#14888=AXIS2_PLACEMENT_3D ( 'NONE', #18314, #5572, #12752 ) ;
#14889=VERTEX_POINT ( 'NONE', #14563 ) ;
#14890=VERTEX_POINT ( 'NONE', #5935 ) ;
#14891=ORIENTED_EDGE ( 'NONE', *, *, #2362, .T. ) ;
#14892=VERTEX_POINT ( 'NONE', #15809 ) ;
#14893=CYLINDRICAL_SURFACE ( 'NONE', #499, 1.500000000000001554 ) ;
#14894=EDGE_CURVE ( 'NONE', #1314, #12681, #6584, .T. ) ;
#14895=EDGE_LOOP ( 'NONE', ( #2609, #11035 ) ) ;
#14896=ORIENTED_EDGE ( 'NONE', *, *, #738, .T. ) ;
#14897=FACE_BOUND ( 'NONE', #10430, .T. ) ;
#14898=VECTOR ( 'NONE', #16420, 1000.000000000000000 ) ;
#14900=ORIENTED_EDGE ( 'NONE', *, *, #3409, .F. ) ;
#14901=EDGE_CURVE ( 'NONE', #13436, #7195, #17188, .T. ) ;
#14902=CIRCLE ( 'NONE', #9166, 1.499999999999999556 ) ;
#14903=ORIENTED_EDGE ( 'NONE', *, *, #15569, .T. ) ;
#14905=CARTESIAN_POINT ( 'NONE',  ( 6.338001773648093362, -76.94993044916168401, -21.65063509461098690 ) ) ;
#14909=DIRECTION ( 'NONE',  ( -0.9876526153536341335, -0.1566598588826327021, 0.000000000000000000 ) ) ;
#14910=EDGE_LOOP ( 'NONE', ( #393, #10833, #16550, #1412 ) ) ;
#14911=ORIENTED_EDGE ( 'NONE', *, *, #17341, .F. ) ;
#14912=DIRECTION ( 'NONE',  ( -0.9876526153536336894, -0.1566598588826349503, 0.000000000000000000 ) ) ;
#14914=FACE_OUTER_BOUND ( 'NONE', #15402, .T. ) ;
#14916=CIRCLE ( 'NONE', #15835, 1.500000000000000888 ) ;
#14917=CARTESIAN_POINT ( 'NONE',  ( -70.20507591625822386, -89.09106951256563889, -8.660254037844385522 ) ) ;
#14918=EDGE_CURVE ( 'NONE', #8286, #7360, #17790, .T. ) ;
#14919=VERTEX_POINT ( 'NONE', #10735 ) ;
#14921=CARTESIAN_POINT ( 'NONE',  ( -72.71384246482016067, -31.78353772342409300, 8.660254037844417496 ) ) ;
#14923=EDGE_CURVE ( 'NONE', #11443, #1825, #1145, .T. ) ;
#14924=DIRECTION ( 'NONE',  ( -0.1566598588826321747, 0.9876526153536343555, 0.000000000000000000 ) ) ;
#14925=DIRECTION ( 'NONE',  ( -0.1566598588826321747, 0.9876526153536343555, 0.000000000000000000 ) ) ;
#14926=CARTESIAN_POINT ( 'NONE',  ( -23.29157668696081629, -81.64972621564064070, -12.99038105676658539 ) ) ;
#14927=AXIS2_PLACEMENT_3D ( 'NONE', #940, #18403, #2241 ) ;
#14928=CARTESIAN_POINT ( 'NONE',  ( -19.17624791478365864, -18.22898240811121440, -8.660254037844380193 ) ) ;
#14930=ORIENTED_EDGE ( 'NONE', *, *, #14306, .F. ) ;
#14931=ORIENTED_EDGE ( 'NONE', *, *, #5698, .F. ) ;
#14932=FACE_OUTER_BOUND ( 'NONE', #7073, .T. ) ;
#14933=ORIENTED_EDGE ( 'NONE', *, *, #9005, .F. ) ;
#14934=VERTEX_POINT ( 'NONE', #16461 ) ;
#14935=DIRECTION ( 'NONE',  ( 0.000000000000000000, 0.000000000000000000, 1.000000000000000000 ) ) ;
#14936=ORIENTED_EDGE ( 'NONE', *, *, #2829, .T. ) ;
#14937=ADVANCED_FACE ( 'NONE', ( #6224 ), #10663, .F. ) ;
#14939=EDGE_CURVE ( 'NONE', #7705, #9461, #3518, .T. ) ;
#14940=DIRECTION ( 'NONE',  ( -0.1566598588826321192, 0.9876526153536342445, 7.798540720466730171E-17 ) ) ;
#14941=ADVANCED_FACE ( 'NONE', ( #17714 ), #9160, .F. ) ;
#14942=CYLINDRICAL_SURFACE ( 'NONE', #13641, 1.500000000000001554 ) ;
#14943=EDGE_CURVE ( 'NONE', #2756, #1785, #8685, .T. ) ;
#14945=DIRECTION ( 'NONE',  ( -0.9876526153536341335, -0.1566598588826327021, 0.000000000000000000 ) ) ;
#14948=CYLINDRICAL_SURFACE ( 'NONE', #9564, 1.500000000000001554 ) ;
#14949=VERTEX_POINT ( 'NONE', #2036 ) ;
#14950=DIRECTION ( 'NONE',  ( -0.1566598588826321192, 0.9876526153536342445, 7.798540720466731404E-17 ) ) ;
#14952=CARTESIAN_POINT ( 'NONE',  ( 11.77009115809307715, -76.08830122530719109, -8.660254037844389075 ) ) ;
#14954=VERTEX_POINT ( 'NONE', #13315 ) ;
#14956=ORIENTED_EDGE ( 'NONE', *, *, #8837, .F. ) ;
#14959=CARTESIAN_POINT ( 'NONE',  ( 2.881217619910392269, -77.49823995525089515, -4.330127018922189208 ) ) ;
#14960=ADVANCED_FACE ( 'NONE', ( #436 ), #4781, .F. ) ;
#14961=EDGE_LOOP ( 'NONE', ( #18657, #11199, #14502, #17432 ) ) ;
#14962=CARTESIAN_POINT ( 'NONE',  ( -35.63723437888118184, -83.60797445167352748, 1.424741226644455312E-14 ) ) ;
#14963=VERTEX_POINT ( 'NONE', #346 ) ;
#14965=DIRECTION ( 'NONE',  ( -0.9876526153536341335, -0.1566598588826327021, 0.000000000000000000 ) ) ;
#14966=DIRECTION ( 'NONE',  ( 0.000000000000000000, 0.000000000000000000, 1.000000000000000000 ) ) ;
#14970=DIRECTION ( 'NONE',  ( -0.1566598588826321192, 0.9876526153536342445, 7.798540720466730171E-17 ) ) ;
#14971=DIRECTION ( 'NONE',  ( 0.000000000000000000, 0.000000000000000000, 1.000000000000000000 ) ) ;
#14973=CARTESIAN_POINT ( 'NONE',  ( -26.58364252993588650, -19.40393134973095002, -21.65063509461097979 ) ) ;
#14974=CYLINDRICAL_SURFACE ( 'NONE', #3545, 1.500000000000001554 ) ;
#14975=ORIENTED_EDGE ( 'NONE', *, *, #18100, .T. ) ;
#14976=DIRECTION ( 'NONE',  ( -0.1566598588826321192, 0.9876526153536342445, 7.798540720466731404E-17 ) ) ;
#14977=ORIENTED_EDGE ( 'NONE', *, *, #16208, .F. ) ;
#14978=CARTESIAN_POINT ( 'NONE',  ( -62.30385499342917655, -87.83779064150456861, -8.660254037844385522 ) ) ;
#14980=CARTESIAN_POINT ( 'NONE',  ( -59.83472345504510770, -87.44614099429800547, 12.99038105676661203 ) ) ;
#14982=ORIENTED_EDGE ( 'NONE', *, *, #16168, .T. ) ;
#14984=ORIENTED_EDGE ( 'NONE', *, *, #2607, .T. ) ;
#14987=ORIENTED_EDGE ( 'NONE', *, *, #2555, .F. ) ;
#14988=AXIS2_PLACEMENT_3D ( 'NONE', #9332, #15118, #2137 ) ;
#14989=FACE_BOUND ( 'NONE', #17776, .T. ) ;
#14990=CARTESIAN_POINT ( 'NONE',  ( -21.81009776393036503, -81.41473642731668292, -4.330127018922185655 ) ) ;
#14992=EDGE_CURVE ( 'NONE', #3473, #13798, #6595, .T. ) ;
#14993=EDGE_CURVE ( 'NONE', #10341, #14647, #3806, .T. ) ;
#14994=ORIENTED_EDGE ( 'NONE', *, *, #4909, .T. ) ;
#14995=DIRECTION ( 'NONE',  ( 0.000000000000000000, 0.000000000000000000, 1.000000000000000000 ) ) ;
#14996=EDGE_CURVE ( 'NONE', #5613, #13071, #15949, .T. ) ;
#14997=CARTESIAN_POINT ( 'NONE',  ( -25.26688191766805858, -81.96304593340589406, 4.330127018922213189 ) ) ;
#14998=VECTOR ( 'NONE', #3605, 1000.000000000000000 ) ;
#14999=CARTESIAN_POINT ( 'NONE',  ( -65.30644784966791860, -30.60858878180435028, 21.65063509461101887 ) ) ;
#15000=DIRECTION ( 'NONE',  ( -0.1566598588826321192, 0.9876526153536342445, 7.798540720466730171E-17 ) ) ;
#15001=CARTESIAN_POINT ( 'NONE',  ( -69.25705831108246002, -31.23522821733487476, 8.660254037844417496 ) ) ;
#15002=CARTESIAN_POINT ( 'NONE',  ( -41.56315007100297265, -84.54793360496931598, -12.99038105676658539 ) ) ;
#15003=EDGE_LOOP ( 'NONE', ( #10383, #3196, #13016, #103 ) ) ;
#15004=VERTEX_POINT ( 'NONE', #5359 ) ;
#15009=ORIENTED_EDGE ( 'NONE', *, *, #15944, .T. ) ;
#15010=DIRECTION ( 'NONE',  ( -0.1566598588826321192, 0.9876526153536342445, 7.798540720466730171E-17 ) ) ;
#15012=FACE_BOUND ( 'NONE', #14291, .T. ) ;
#15013=DIRECTION ( 'NONE',  ( -0.9876526153536341335, -0.1566598588826327021, 0.000000000000000000 ) ) ;
#15014=CARTESIAN_POINT ( 'NONE',  ( -57.20087360589840131, -24.26038697509254405, 8.660254037844417496 ) ) ;
#15016=EDGE_CURVE ( 'NONE', #2581, #1938, #15394, .T. ) ;
#15018=CARTESIAN_POINT ( 'NONE',  ( -25.10216360690543524, -19.16894156140701710, 12.99038105676661736 ) ) ;
#15020=ORIENTED_EDGE ( 'NONE', *, *, #8296, .T. ) ;
#15021=DIRECTION ( 'NONE',  ( -0.9876526153536341335, -0.1566598588826327021, 0.000000000000000000 ) ) ;
#15022=AXIS2_PLACEMENT_3D ( 'NONE', #7850, #6446, #4708 ) ;
#15024=EDGE_CURVE ( 'NONE', #1839, #12162, #2634, .T. ) ;
#15025=VERTEX_POINT ( 'NONE', #6887 ) ;
#15026=FACE_OUTER_BOUND ( 'NONE', #16246, .T. ) ;
#15027=VERTEX_POINT ( 'NONE', #8202 ) ;
#15028=AXIS2_PLACEMENT_3D ( 'NONE', #11993, #8990, #7762 ) ;
#15029=DIRECTION ( 'NONE',  ( -0.9876526153536336894, -0.1566598588826349503, 0.000000000000000000 ) ) ;
#15030=DIRECTION ( 'NONE',  ( -0.1566598588826321192, 0.9876526153536342445, 7.798540720466730171E-17 ) ) ;
#15031=DIRECTION ( 'NONE',  ( -0.9876526153536336894, -0.1566598588826350336, 0.000000000000000000 ) ) ;
#15032=VECTOR ( 'NONE', #5052, 1000.000000000000000 ) ;
#15033=ADVANCED_FACE ( 'NONE', ( #919 ), #16750, .F. ) ;
#15035=DIRECTION ( 'NONE',  ( -0.1566598588826321192, 0.9876526153536342445, 7.798540720466730171E-17 ) ) ;
#15037=CARTESIAN_POINT ( 'NONE',  ( -11.93357161039406300, -79.84813783849035929, -21.65063509461098690 ) ) ;
#15038=FACE_OUTER_BOUND ( 'NONE', #2522, .T. ) ;
#15040=AXIS2_PLACEMENT_3D ( 'NONE', #5578, #11325, #15698 ) ;
#15041=EDGE_CURVE ( 'NONE', #4072, #9210, #16938, .T. ) ;
#15042=DIRECTION ( 'NONE',  ( -0.1566598588826321192, 0.9876526153536342445, 7.798540720466730171E-17 ) ) ;
#15043=ORIENTED_EDGE ( 'NONE', *, *, #8805, .F. ) ;
#15044=DIRECTION ( 'NONE',  ( 1.000000000000000000, 0.000000000000000000, 0.000000000000000000 ) ) ;
#15047=ORIENTED_EDGE ( 'NONE', *, *, #7031, .T. ) ;
#15048=EDGE_CURVE ( 'NONE', #9221, #3679, #5964, .T. ) ;
#15049=DIRECTION ( 'NONE',  ( 0.000000000000000000, 0.000000000000000000, 1.000000000000000000 ) ) ;
#15050=VERTEX_POINT ( 'NONE', #2312 ) ;
#15052=ORIENTED_EDGE ( 'NONE', *, *, #7659, .T. ) ;
#15053=DIRECTION ( 'NONE',  ( -0.9876526153536341335, -0.1566598588826327021, 0.000000000000000000 ) ) ;
#15054=ORIENTED_EDGE ( 'NONE', *, *, #2436, .F. ) ;
#15055=CIRCLE ( 'NONE', #14748, 1.500000000000000444 ) ;
#15056=CARTESIAN_POINT ( 'NONE',  ( -10.28737437660097775, -16.81904367816753165, 21.65063509461101177 ) ) ;
#15057=ORIENTED_EDGE ( 'NONE', *, *, #13362, .T. ) ;
#15058=DIRECTION ( 'NONE',  ( -0.9876526153536341335, -0.1566598588826327021, 0.000000000000000000 ) ) ;
#15063=FACE_OUTER_BOUND ( 'NONE', #1135, .T. ) ;
#15064=EDGE_CURVE ( 'NONE', #10341, #1641, #7781, .T. ) ;
#15065=ORIENTED_EDGE ( 'NONE', *, *, #2335, .T. ) ;
#15067=EDGE_CURVE ( 'NONE', #4379, #14, #8095, .T. ) ;
#15069=CARTESIAN_POINT ( 'NONE',  ( -84.23462711737164454, 33.01666666666666572, 35.00000000000000000 ) ) ;
#15070=CIRCLE ( 'NONE', #7817, 1.500000000000000888 ) ;
#15071=ORIENTED_EDGE ( 'NONE', *, *, #12361, .T. ) ;
#15072=VERTEX_POINT ( 'NONE', #11017 ) ;
#15074=CYLINDRICAL_SURFACE ( 'NONE', #5648, 1.500000000000001554 ) ;
#15075=AXIS2_PLACEMENT_3D ( 'NONE', #13531, #581, #6371 ) ;
#15076=FACE_BOUND ( 'NONE', #13095, .T. ) ;
#15078=DIRECTION ( 'NONE',  ( 0.000000000000000000, 0.000000000000000000, 1.000000000000000000 ) ) ;
#15079=DIRECTION ( 'NONE',  ( -0.1566598588826321192, 0.9876526153536342445, 7.798540720466730171E-17 ) ) ;
#15080=ORIENTED_EDGE ( 'NONE', *, *, #14761, .T. ) ;
#15081=CIRCLE ( 'NONE', #12044, 1.500000000000000888 ) ;
#15082=AXIS2_PLACEMENT_3D ( 'NONE', #15619, #8255, #2553 ) ;
#15083=VERTEX_POINT ( 'NONE', #14061 ) ;
#15084=DIRECTION ( 'NONE',  ( -0.1566598588826321192, 0.9876526153536342445, 7.798540720466730171E-17 ) ) ;
#15085=EDGE_LOOP ( 'NONE', ( #8044, #1573 ) ) ;
#15086=DIRECTION ( 'NONE',  ( -0.1566598588826321192, 0.9876526153536342445, 7.798540720466730171E-17 ) ) ;
#15087=DIRECTION ( 'NONE',  ( -0.1566598588826321192, 0.9876526153536342445, 7.798540720466730171E-17 ) ) ;
#15089=ORIENTED_EDGE ( 'NONE', *, *, #2341, .F. ) ;
#15090=ORIENTED_EDGE ( 'NONE', *, *, #10140, .T. ) ;
#15091=CARTESIAN_POINT ( 'NONE',  ( -16.70711637639958269, -17.83733276090463704, 4.330127018922218518 ) ) ;
#15093=LINE ( 'NONE', #7905, #15357 ) ;
#15094=EDGE_CURVE ( 'NONE', #10171, #7400, #12599, .T. ) ;
#15095=CARTESIAN_POINT ( 'NONE',  ( -19.38060123572413218, -23.32390534376198232, 4.330127018922217630 ) ) ;
#15096=CIRCLE ( 'NONE', #14201, 1.499999999999999556 ) ;
#15098=EDGE_CURVE ( 'NONE', #8327, #5727, #6893, .T. ) ;
#15099=AXIS2_PLACEMENT_3D ( 'NONE', #5027, #707, #9597 ) ;
#15100=ORIENTED_EDGE ( 'NONE', *, *, #2582, .T. ) ;
#15101=CARTESIAN_POINT ( 'NONE',  ( -32.50955822205765600, -20.34389050302674207, -17.32050807568878170 ) ) ;
#15102=CARTESIAN_POINT ( 'NONE',  ( -52.96079015774756726, -28.65034054577146705, -17.32050807568878170 ) ) ;
#15103=CIRCLE ( 'NONE', #3290, 1.500000000000000888 ) ;
#15105=EDGE_CURVE ( 'NONE', #12855, #3591, #12248, .T. ) ;
#15106=AXIS2_PLACEMENT_3D ( 'NONE', #2885, #18775, #4501 ) ;
#15107=CIRCLE ( 'NONE', #6657, 1.500000000000001332 ) ;
#15108=DIRECTION ( 'NONE',  ( -0.1566598588826321192, 0.9876526153536342445, 7.798540720466730171E-17 ) ) ;
#15109=FACE_OUTER_BOUND ( 'NONE', #3415, .T. ) ;
#15110=DIRECTION ( 'NONE',  ( -0.1566598588826321192, 0.9876526153536342445, 7.798540720466730171E-17 ) ) ;
#15112=CIRCLE ( 'NONE', #15710, 1.500000000000000888 ) ;
#15113=CARTESIAN_POINT ( 'NONE',  ( -79.13358446461874962, -32.80182680616118773, 1.869203119972154228E-14 ) ) ;
#15114=CIRCLE ( 'NONE', #18506, 1.500000000000000888 ) ;
#15116=ORIENTED_EDGE ( 'NONE', *, *, #1826, .T. ) ;
#15118=DIRECTION ( 'NONE',  ( -0.1566598588826321747, 0.9876526153536343555, 0.000000000000000000 ) ) ;
#15119=AXIS2_PLACEMENT_3D ( 'NONE', #16059, #1568, #7260 ) ;
#15120=ORIENTED_EDGE ( 'NONE', *, *, #9378, .T. ) ;
#15121=ORIENTED_EDGE ( 'NONE', *, *, #15384, .F. ) ;
#15122=DIRECTION ( 'NONE',  ( -0.1566598588826321192, 0.9876526153536342445, 7.798540720466731404E-17 ) ) ;
#15123=VECTOR ( 'NONE', #9063, 1000.000000000000000 ) ;
#15124=AXIS2_PLACEMENT_3D ( 'NONE', #16037, #8736, #11374 ) ;
#15125=ORIENTED_EDGE ( 'NONE', *, *, #13666, .F. ) ;
#15129=AXIS2_PLACEMENT_3D ( 'NONE', #7594, #10415, #17382 ) ;
#15130=ADVANCED_FACE ( 'NONE', ( #11486, #14358 ), #3629, .F. ) ;
#15131=AXIS2_PLACEMENT_3D ( 'NONE', #14811, #4663, #17695 ) ;
#15132=CARTESIAN_POINT ( 'NONE',  ( -20.86208015875457988, -23.55889513208593655, -12.99038105676658006 ) ) ;
#15133=AXIS2_PLACEMENT_3D ( 'NONE', #5239, #16914, #15473 ) ;
#15135=DIRECTION ( 'NONE',  ( -0.9876526153536341335, -0.1566598588826327576, 0.000000000000000000 ) ) ;
#15136=AXIS2_PLACEMENT_3D ( 'NONE', #7956, #18034, #760 ) ;
#15137=CARTESIAN_POINT ( 'NONE',  ( -12.75650591498505371, -17.21069332537411256, 17.32050807568881012 ) ) ;
#15138=EDGE_CURVE ( 'NONE', #16734, #1864, #17323, .T. ) ;
#15139=CARTESIAN_POINT ( 'NONE',  ( -18.35331361019266794, -80.86642692122748599, 12.99038105676661203 ) ) ;
#15141=AXIS2_PLACEMENT_3D ( 'NONE', #1239, #12567, #9557 ) ;
#15142=CARTESIAN_POINT ( 'NONE',  ( 3.231158466157551423, 19.73726462726227737, -30.00000000000000000 ) ) ;
#15145=AXIS2_PLACEMENT_3D ( 'NONE', #11373, #15559, #12892 ) ;
#15146=CARTESIAN_POINT ( 'NONE',  ( -76.95392591297100182, -27.39358415274516645, -17.32050807568878170 ) ) ;
#15147=ORIENTED_EDGE ( 'NONE', *, *, #1045, .F. ) ;
#15149=CIRCLE ( 'NONE', #3626, 1.500000000000000888 ) ;
#15150=CARTESIAN_POINT ( 'NONE',  ( -0.1213752363283457369, -20.26903809555066616, -8.660254037844383745 ) ) ;
#15151=CIRCLE ( 'NONE', #14838, 1.500000000000001332 ) ;
#15152=EDGE_CURVE ( 'NONE', #14323, #10331, #8699, .T. ) ;
#15154=CIRCLE ( 'NONE', #17612, 1.500000000000000000 ) ;
#15155=EDGE_CURVE ( 'NONE', #11172, #495, #10497, .T. ) ;
#15156=CARTESIAN_POINT ( 'NONE',  ( -60.32854976272193426, -87.52447092373931525, -17.32050807568878525 ) ) ;
#15157=VECTOR ( 'NONE', #67, 1000.000000000000000 ) ;
#15158=DIRECTION ( 'NONE',  ( -0.9876526153536336894, -0.1566598588826350336, 0.000000000000000000 ) ) ;
#15159=AXIS2_PLACEMENT_3D ( 'NONE', #10667, #4883, #11879 ) ;
#15160=ORIENTED_EDGE ( 'NONE', *, *, #6145, .F. ) ;
#15161=DIRECTION ( 'NONE',  ( -0.1566598588826321192, 0.9876526153536342445, 7.798540720466730171E-17 ) ) ;
#15162=EDGE_CURVE ( 'NONE', #16506, #5655, #16260, .T. ) ;
#15163=CARTESIAN_POINT ( 'NONE',  ( -79.91688375903190433, -27.86356372939306780, 8.660254037844417496 ) ) ;
#15164=CARTESIAN_POINT ( 'NONE',  ( -58.84707083969148300, -87.28948113541537168, 8.660254037844412167 ) ) ;
#15166=VERTEX_POINT ( 'NONE', #8668 ) ;
#15167=CIRCLE ( 'NONE', #5815, 1.500000000000000888 ) ;
#15168=CYLINDRICAL_SURFACE ( 'NONE', #17038, 1.500000000000001554 ) ;
#15169=CARTESIAN_POINT ( 'NONE',  ( -72.01566283620284992, -26.61028485833201529, 1.926565525561697761E-14 ) ) ;
#15170=VECTOR ( 'NONE', #4792, 1000.000000000000000 ) ;
#15171=FACE_OUTER_BOUND ( 'NONE', #6448, .T. ) ;
#15173=EDGE_LOOP ( 'NONE', ( #11944, #1766 ) ) ;
#15174=ORIENTED_EDGE ( 'NONE', *, *, #5337, .T. ) ;
#15175=ORIENTED_EDGE ( 'NONE', *, *, #15094, .T. ) ;
#15176=DIRECTION ( 'NONE',  ( -0.000000000000000000, -0.000000000000000000, -1.000000000000000000 ) ) ;
#15177=EDGE_CURVE ( 'NONE', #2115, #15396, #2331, .T. ) ;
#15179=ORIENTED_EDGE ( 'NONE', *, *, #1297, .T. ) ;
#15180=FACE_BOUND ( 'NONE', #9399, .T. ) ;
#15181=EDGE_CURVE ( 'NONE', #1617, #6871, #11988, .T. ) ;
#15182=EDGE_CURVE ( 'NONE', #11831, #9589, #15351, .T. ) ;
#15183=VERTEX_POINT ( 'NONE', #11396 ) ;
#15184=EDGE_CURVE ( 'NONE', #17699, #9820, #11101, .T. ) ;
#15185=DIRECTION ( 'NONE',  ( -0.1566598588826321747, 0.9876526153536343555, 0.000000000000000000 ) ) ;
#15186=ORIENTED_EDGE ( 'NONE', *, *, #17341, .T. ) ;
#15187=AXIS2_PLACEMENT_3D ( 'NONE', #7710, #13462, #504 ) ;
#15188=CIRCLE ( 'NONE', #17649, 1.500000000000000888 ) ;
#15190=DIRECTION ( 'NONE',  ( -0.1566598588826321192, 0.9876526153536342445, 7.798540720466731404E-17 ) ) ;
#15192=AXIS2_PLACEMENT_3D ( 'NONE', #3474, #7407, #10409 ) ;
#15193=CARTESIAN_POINT ( 'NONE',  ( -16.87183468716221313, -80.63143713290352821, -12.99038105676658539 ) ) ;
#15194=ORIENTED_EDGE ( 'NONE', *, *, #14996, .T. ) ;
#15196=DIRECTION ( 'NONE',  ( -0.1566598588826321192, 0.9876526153536342445, 7.798540720466730171E-17 ) ) ;
#15197=CYLINDRICAL_SURFACE ( 'NONE', #6596, 1.500000000000001554 ) ;
#15199=EDGE_LOOP ( 'NONE', ( #15270, #13545 ) ) ;
#15202=DIRECTION ( 'NONE',  ( -0.1566598588826321747, 0.9876526153536343555, 0.000000000000000000 ) ) ;
#15203=VECTOR ( 'NONE', #6103, 1000.000000000000114 ) ;
#15206=DIRECTION ( 'NONE',  ( -0.9876526153536344665, -0.1566598588826304539, 0.000000000000000000 ) ) ;
#15208=ADVANCED_FACE ( 'NONE', ( #15576 ), #5740, .F. ) ;
#15209=ADVANCED_FACE ( 'NONE', ( #14446 ), #15958, .F. ) ;
#15210=DIRECTION ( 'NONE',  ( -0.9876526153536341335, -0.1566598588826327021, 0.000000000000000000 ) ) ;
#15212=DIRECTION ( 'NONE',  ( -0.1566598588826321192, 0.9876526153536342445, 7.798540720466730171E-17 ) ) ;
#15213=EDGE_LOOP ( 'NONE', ( #10741, #18234, #2825, #1077 ) ) ;
#15214=ORIENTED_EDGE ( 'NONE', *, *, #9618, .F. ) ;
#15215=CIRCLE ( 'NONE', #11866, 1.500000000000000888 ) ;
#15216=DIRECTION ( 'NONE',  ( -0.1566598588826321747, 0.9876526153536343555, 0.000000000000000000 ) ) ;
#15217=VERTEX_POINT ( 'NONE', #14269 ) ;
#15218=ORIENTED_EDGE ( 'NONE', *, *, #9952, .T. ) ;
#15219=FACE_OUTER_BOUND ( 'NONE', #16401, .T. ) ;
#15220=LINE ( 'NONE', #2239, #3639 ) ;
#15221=AXIS2_PLACEMENT_3D ( 'NONE', #13252, #6460, #4913 ) ;
#15222=ORIENTED_EDGE ( 'NONE', *, *, #11966, .T. ) ;
#15223=CARTESIAN_POINT ( 'NONE',  ( -47.98289207080154739, -85.56622268770644268, 21.65063509461101532 ) ) ;
#15226=EDGE_CURVE ( 'NONE', #1436, #11647, #5680, .T. ) ;
#15227=ADVANCED_FACE ( 'NONE', ( #6990 ), #12730, .F. ) ;
#15228=CYLINDRICAL_SURFACE ( 'NONE', #7846, 1.500000000000001554 ) ;
#15229=DIRECTION ( 'NONE',  ( -0.9876526153536336894, -0.1566598588826349503, 0.000000000000000000 ) ) ;
#15230=CARTESIAN_POINT ( 'NONE',  ( -25.76070822534488869, -82.04137586284720385, 1.424741226644455312E-14 ) ) ;
#15231=DIRECTION ( 'NONE',  ( -0.1566598588826321192, 0.9876526153536342445, 7.798540720466730171E-17 ) ) ;
#15232=EDGE_CURVE ( 'NONE', #10493, #592, #10575, .T. ) ;
#15233=DIRECTION ( 'NONE',  ( -0.1566598588826321747, 0.9876526153536343555, 0.000000000000000000 ) ) ;
#15234=ORIENTED_EDGE ( 'NONE', *, *, #16407, .F. ) ;
#15235=CARTESIAN_POINT ( 'NONE',  ( -30.04042668367358360, -19.95224085582016116, -21.65063509461098334 ) ) ;
#15237=ORIENTED_EDGE ( 'NONE', *, *, #16230, .F. ) ;
#15238=ORIENTED_EDGE ( 'NONE', *, *, #11658, .T. ) ;
#15239=CARTESIAN_POINT ( 'NONE',  ( -56.21322099054477661, -24.10372711620990671, 4.330127018922218518 ) ) ;
#15241=CARTESIAN_POINT ( 'NONE',  ( -30.69897130211303349, -82.82467515726038698, 8.660254037844412167 ) ) ;
#15242=VERTEX_POINT ( 'NONE', #1655 ) ;
#15243=FACE_OUTER_BOUND ( 'NONE', #8175, .T. ) ;
#15244=CARTESIAN_POINT ( 'NONE',  ( -76.66445292623467367, -32.41017715895461038, -4.330127018922181215 ) ) ;
#15247=CARTESIAN_POINT ( 'NONE',  ( -47.32434745236209750, -22.69378838626622752, 8.660254037844417496 ) ) ;
#15248=CARTESIAN_POINT ( 'NONE',  ( -84.16561914167408531, 33.59999999999999432, 30.00000000000000000 ) ) ;
#15249=DIRECTION ( 'NONE',  ( -0.9876526153536336894, -0.1566598588826349503, 0.000000000000000000 ) ) ;
#15250=DIRECTION ( 'NONE',  ( -0.9876526153536341335, -0.1566598588826327021, 0.000000000000000000 ) ) ;
#15251=FILL_AREA_STYLE_COLOUR ( '', #18587 ) ;
#15254=ORIENTED_EDGE ( 'NONE', *, *, #2059, .F. ) ;
#15255=DIRECTION ( 'NONE',  ( -0.9876526153536336894, -0.1566598588826350336, 0.000000000000000000 ) ) ;
#15256=ORIENTED_EDGE ( 'NONE', *, *, #5714, .F. ) ;
#15257=EDGE_CURVE ( 'NONE', #3679, #9221, #12694, .T. ) ;
#15258=ORIENTED_EDGE ( 'NONE', *, *, #8811, .T. ) ;
#15259=VERTEX_POINT ( 'NONE', #9029 ) ;
#15260=CARTESIAN_POINT ( 'NONE',  ( -4.526176995241833367, -78.67318889687062722, -17.32050807568878525 ) ) ;
#15261=FACE_BOUND ( 'NONE', #9090, .T. ) ;
#15264=CIRCLE ( 'NONE', #17422, 1.499999999999999556 ) ;
#15265=ORIENTED_EDGE ( 'NONE', *, *, #11715, .F. ) ;
#15266=DIRECTION ( 'NONE',  ( -0.1566598588826321192, 0.9876526153536342445, 7.798540720466730171E-17 ) ) ;
#15267=CARTESIAN_POINT ( 'NONE',  ( -71.02801022084922522, -26.45362499944938506, 12.99038105676661736 ) ) ;
#15268=FACE_BOUND ( 'NONE', #6133, .T. ) ;
#15269=DIRECTION ( 'NONE',  ( -0.1566598588826321192, 0.9876526153536342445, 7.798540720466731404E-17 ) ) ;
#15270=ORIENTED_EDGE ( 'NONE', *, *, #960, .T. ) ;
#15271=CYLINDRICAL_SURFACE ( 'NONE', #621, 1.500000000000001554 ) ;
#15272=DIRECTION ( 'NONE',  ( 0.000000000000000000, 0.000000000000000000, 1.000000000000000000 ) ) ;
#15273=DIRECTION ( 'NONE',  ( -0.1566598588826321747, 0.9876526153536343555, 0.000000000000000000 ) ) ;
#15274=EDGE_CURVE ( 'NONE', #14342, #2732, #11773, .T. ) ;
#15275=EDGE_LOOP ( 'NONE', ( #3090, #10129, #13202, #15460 ) ) ;
#15277=CARTESIAN_POINT ( 'NONE',  ( -50.49165861936347710, -28.25869089856488614, 4.330127018922217630 ) ) ;
#15279=CIRCLE ( 'NONE', #18366, 1.499999999999999556 ) ;
#15280=ADVANCED_FACE ( 'NONE', ( #16440 ), #16336, .F. ) ;
#15282=ORIENTED_EDGE ( 'NONE', *, *, #12086, .T. ) ;
#15283=ORIENTED_EDGE ( 'NONE', *, *, #280, .T. ) ;
#15284=DIRECTION ( 'NONE',  ( -0.9876526153536341335, -0.1566598588826327021, 0.000000000000000000 ) ) ;
#15285=ORIENTED_EDGE ( 'NONE', *, *, #17465, .F. ) ;
#15286=DIRECTION ( 'NONE',  ( -0.9876526153536336894, -0.1566598588826349503, 0.000000000000000000 ) ) ;
#15288=CARTESIAN_POINT ( 'NONE',  ( -39.09401853261887538, -84.15628395776273862, 8.660254037844412167 ) ) ;
#15289=CIRCLE ( 'NONE', #7739, 1.500000000000000888 ) ;
#15290=CARTESIAN_POINT ( 'NONE',  ( -71.72618984946653597, -31.62687786454144856, -12.99038105676658006 ) ) ;
#15293=DIRECTION ( 'NONE',  ( -0.1566598588826321192, 0.9876526153536342445, 7.798540720466730171E-17 ) ) ;
#15294=DIRECTION ( 'NONE',  ( -0.9876526153536336894, -0.1566598588826349503, 0.000000000000000000 ) ) ;
#15295=CARTESIAN_POINT ( 'NONE',  ( 0.3724510713484854851, -20.19070816610934926, 12.99038105676661026 ) ) ;
#15297=EDGE_CURVE ( 'NONE', #4549, #15692, #4824, .T. ) ;
#15298=DIRECTION ( 'NONE',  ( -0.1566598588826321192, 0.9876526153536342445, 7.798540720466730171E-17 ) ) ;
#15299=ORIENTED_EDGE ( 'NONE', *, *, #4469, .F. ) ;
#15300=ORIENTED_EDGE ( 'NONE', *, *, #6249, .T. ) ;
#15301=FACE_BOUND ( 'NONE', #15199, .T. ) ;
#15302=DIRECTION ( 'NONE',  ( 0.000000000000000000, 0.000000000000000000, 1.000000000000000000 ) ) ;
#15304=AXIS2_PLACEMENT_3D ( 'NONE', #12470, #5278, #12360 ) ;
#15305=ORIENTED_EDGE ( 'NONE', *, *, #15486, .F. ) ;
#15306=ORIENTED_EDGE ( 'NONE', *, *, #9297, .F. ) ;
#15307=EDGE_LOOP ( 'NONE', ( #3725, #828 ) ) ;
#15308=EDGE_CURVE ( 'NONE', #3849, #859, #15436, .T. ) ;
#15309=VERTEX_POINT ( 'NONE', #3145 ) ;
#15310=AXIS2_PLACEMENT_3D ( 'NONE', #12870, #6061, #11977 ) ;
#15311=ORIENTED_EDGE ( 'NONE', *, *, #3822, .T. ) ;
#15312=DIRECTION ( 'NONE',  ( 0.000000000000000000, 0.000000000000000000, 1.000000000000000000 ) ) ;
#15313=CARTESIAN_POINT ( 'NONE',  ( -8.476787456656362352, -79.29982833240116236, -4.330127018922185655 ) ) ;
#15314=ORIENTED_EDGE ( 'NONE', *, *, #14335, .T. ) ;
#15316=AXIS2_PLACEMENT_3D ( 'NONE', #18005, #16552, #13491 ) ;
#15317=CARTESIAN_POINT ( 'NONE',  ( -57.69469991357522076, -24.33871690453386094, 21.65063509461101887 ) ) ;
#15318=FACE_OUTER_BOUND ( 'NONE', #2044, .T. ) ;
#15319=( NAMED_UNIT ( * ) SI_UNIT ( $, .STERADIAN. ) SOLID_ANGLE_UNIT ( ) );
#15320=DIRECTION ( 'NONE',  ( -0.1566598588826321192, 0.9876526153536342445, 7.798540720466730171E-17 ) ) ;
#15321=VECTOR ( 'NONE', #9179, 1000.000000000000000 ) ;
#15322=DIRECTION ( 'NONE',  ( -0.1566598588826321192, 0.9876526153536342445, 7.798540720466730171E-17 ) ) ;
#15323=CARTESIAN_POINT ( 'NONE',  ( 8.807133312032172867, -76.55828080195509244, -17.32050807568878525 ) ) ;
#15324=CARTESIAN_POINT ( 'NONE',  ( -4.526176995241833367, -78.67318889687062722, 17.32050807568880657 ) ) ;
#15327=CIRCLE ( 'NONE', #11081, 1.500000000000000888 ) ;
#15328=LINE ( 'NONE', #16878, #16325 ) ;
#15329=ORIENTED_EDGE ( 'NONE', *, *, #9435, .F. ) ;
#15330=EDGE_CURVE ( 'NONE', #11583, #18320, #14219, .T. ) ;
#15331=DIRECTION ( 'NONE',  ( -0.1566598588826321192, 0.9876526153536342445, 7.798540720466731404E-17 ) ) ;
#15333=AXIS2_PLACEMENT_3D ( 'NONE', #5169, #18384, #1024 ) ;
#15334=DIRECTION ( 'NONE',  ( -0.1566598588826321192, 0.9876526153536342445, 7.798540720466730171E-17 ) ) ;
#15337=EDGE_CURVE ( 'NONE', #6519, #13656, #11661, .T. ) ;
#15338=DIRECTION ( 'NONE',  ( 2.887450008416415878E-16, 0.000000000000000000, 1.000000000000000000 ) ) ;
#15339=DIRECTION ( 'NONE',  ( -0.1566598588826321192, 0.9876526153536342445, 7.798540720466730171E-17 ) ) ;
#15340=EDGE_LOOP ( 'NONE', ( #439, #11986 ) ) ;
#15341=AXIS2_PLACEMENT_3D ( 'NONE', #6611, #6719, #15029 ) ;
#15342=CARTESIAN_POINT ( 'NONE',  ( -29.05277406831996245, -19.79558099693753093, -17.32050807568878170 ) ) ;
#15346=DIRECTION ( 'NONE',  ( -0.1566598588826321192, 0.9876526153536342445, 7.798540720466730171E-17 ) ) ;
#15348=DIRECTION ( 'NONE',  ( -0.1566598588826321192, 0.9876526153536342445, 7.798540720466730171E-17 ) ) ;
#15349=ORIENTED_EDGE ( 'NONE', *, *, #16724, .F. ) ;
#15351=CIRCLE ( 'NONE', #14453, 1.500000000000000444 ) ;
#15352=DIRECTION ( 'NONE',  ( -0.1566598588826321192, 0.9876526153536342445, 7.798540720466730171E-17 ) ) ;
#15353=ORIENTED_EDGE ( 'NONE', *, *, #7664, .F. ) ;
#15354=ORIENTED_EDGE ( 'NONE', *, *, #3556, .T. ) ;
#15356=LINE ( 'NONE', #9294, #14722 ) ;
#15357=VECTOR ( 'NONE', #16349, 1000.000000000000000 ) ;
#15358=FACE_BOUND ( 'NONE', #4643, .T. ) ;
#15359=EDGE_CURVE ( 'NONE', #5533, #9341, #7278, .T. ) ;
#15361=EDGE_LOOP ( 'NONE', ( #14145, #9157, #13772, #2900 ) ) ;
#15362=VECTOR ( 'NONE', #17230, 1000.000000000000000 ) ;
#15363=DIRECTION ( 'NONE',  ( 0.000000000000000000, 0.000000000000000000, 1.000000000000000000 ) ) ;
#15364=DIRECTION ( 'NONE',  ( 0.000000000000000000, 0.000000000000000000, 1.000000000000000000 ) ) ;
#15365=EDGE_CURVE ( 'NONE', #3093, #18006, #6046, .T. ) ;
#15366=CYLINDRICAL_SURFACE ( 'NONE', #18215, 1.500000000000001554 ) ;
#15367=ORIENTED_EDGE ( 'NONE', *, *, #14027, .F. ) ;
#15368=DIRECTION ( 'NONE',  ( -0.1566598588826321192, 0.9876526153536342445, 7.798540720466731404E-17 ) ) ;
#15369=CYLINDRICAL_SURFACE ( 'NONE', #18152, 1.500000000000001554 ) ;
#15370=DIRECTION ( 'NONE',  ( -0.9876526153536341335, -0.1566598588826327021, 0.000000000000000000 ) ) ;
#15372=ORIENTED_EDGE ( 'NONE', *, *, #8382, .F. ) ;
#15373=FACE_OUTER_BOUND ( 'NONE', #12066, .T. ) ;
#15374=ORIENTED_EDGE ( 'NONE', *, *, #15105, .T. ) ;
#15375=DIRECTION ( 'NONE',  ( 0.000000000000000000, 0.000000000000000000, 1.000000000000000000 ) ) ;
#15376=VECTOR ( 'NONE', #1249, 1000.000000000000000 ) ;
#15378=VERTEX_POINT ( 'NONE', #14635 ) ;
#15379=ORIENTED_EDGE ( 'NONE', *, *, #16123, .F. ) ;
#15380=LINE ( 'NONE', #8288, #9743 ) ;
#15381=EDGE_LOOP ( 'NONE', ( #15174, #3606 ) ) ;
#15382=CARTESIAN_POINT ( 'NONE',  ( -52.96079015774756016, -28.65034054577145994, 8.660254037844417496 ) ) ;
#15383=CYLINDRICAL_SURFACE ( 'NONE', #3000, 1.500000000000001554 ) ;
#15384=EDGE_CURVE ( 'NONE', #11742, #1595, #6989, .T. ) ;
#15385=FACE_BOUND ( 'NONE', #18324, .T. ) ;
#15386=AXIS2_PLACEMENT_3D ( 'NONE', #1575, #8862, #7171 ) ;
#15387=FACE_OUTER_BOUND ( 'NONE', #5187, .T. ) ;
#15389=EDGE_CURVE ( 'NONE', #13798, #384, #3018, .T. ) ;
#15390=CIRCLE ( 'NONE', #8451, 1.499999999999999556 ) ;
#15391=DIRECTION ( 'NONE',  ( -0.1566598588826321192, 0.9876526153536342445, 7.798540720466730171E-17 ) ) ;
#15392=EDGE_CURVE ( 'NONE', #1506, #12855, #3906, .T. ) ;
#15393=CARTESIAN_POINT ( 'NONE',  ( -29.75095369693726610, -24.96883386202961574, 1.869203119972154228E-14 ) ) ;
#15394=LINE ( 'NONE', #10828, #16565 ) ;
#15395=FACE_OUTER_BOUND ( 'NONE', #9923, .T. ) ;
#15396=VERTEX_POINT ( 'NONE', #507 ) ;
#15397=EDGE_LOOP ( 'NONE', ( #924, #6112 ) ) ;
#15399=DIRECTION ( 'NONE',  ( -0.1566598588826321192, 0.9876526153536342445, 7.798540720466730171E-17 ) ) ;
#15400=AXIS2_PLACEMENT_3D ( 'NONE', #15561, #11644, #1367 ) ;
#15401=ORIENTED_EDGE ( 'NONE', *, *, #12486, .T. ) ;
#15402=EDGE_LOOP ( 'NONE', ( #13006, #16400, #14346, #252 ) ) ;
#15405=DIRECTION ( 'NONE',  ( -0.9876526153536344665, -0.1566598588826304539, 0.000000000000000000 ) ) ;
#15406=CIRCLE ( 'NONE', #6349, 1.500000000000000888 ) ;
#15407=ORIENTED_EDGE ( 'NONE', *, *, #1330, .F. ) ;
#15408=ORIENTED_EDGE ( 'NONE', *, *, #8662, .F. ) ;
#15409=DIRECTION ( 'NONE',  ( -0.1566598588826321192, 0.9876526153536342445, 7.798540720466730171E-17 ) ) ;
#15410=CYLINDRICAL_SURFACE ( 'NONE', #15304, 1.500000000000001554 ) ;
#15411=FACE_OUTER_BOUND ( 'NONE', #18541, .T. ) ;
#15412=EDGE_CURVE ( 'NONE', #4575, #14954, #11858, .T. ) ;
#15414=AXIS2_PLACEMENT_3D ( 'NONE', #8577, #12719, #14348 ) ;
#15415=EDGE_CURVE ( 'NONE', #2, #12073, #8477, .T. ) ;
#15416=CARTESIAN_POINT ( 'NONE',  ( 9.300959619709004755, -76.47995087251376845, 12.99038105676660493 ) ) ;
#15418=LINE ( 'NONE', #18011, #3720 ) ;
#15422=CARTESIAN_POINT ( 'NONE',  ( -25.10216360690543524, -19.16894156140701710, 21.65063509461101887 ) ) ;
#15423=AXIS2_PLACEMENT_3D ( 'NONE', #2558, #976, #18141 ) ;
#15424=AXIS2_PLACEMENT_3D ( 'NONE', #5164, #8089, #10926 ) ;
#15425=VERTEX_POINT ( 'NONE', #12429 ) ;
#15427=DIRECTION ( 'NONE',  ( -0.1566598588826321192, 0.9876526153536342445, 7.798540720466731404E-17 ) ) ;
#15430=CARTESIAN_POINT ( 'NONE',  ( -67.07739975943471222, -25.82698556391885703, 1.926565525561698076E-14 ) ) ;
#15432=ORIENTED_EDGE ( 'NONE', *, *, #5264, .T. ) ;
#15433=AXIS2_PLACEMENT_3D ( 'NONE', #2733, #8525, #1332 ) ;
#15436=CIRCLE ( 'NONE', #4534, 1.500000000000000888 ) ;
#15439=VERTEX_POINT ( 'NONE', #17974 ) ;
#15440=AXIS2_PLACEMENT_3D ( 'NONE', #11954, #17800, #10561 ) ;
#15441=CIRCLE ( 'NONE', #5772, 2.500000000000002220 ) ;
#15442=CYLINDRICAL_SURFACE ( 'NONE', #1577, 1.500000000000001554 ) ;
#15443=VERTEX_POINT ( 'NONE', #2109 ) ;
#15444=DIRECTION ( 'NONE',  ( -0.1566598588826321192, 0.9876526153536342445, 7.798540720466731404E-17 ) ) ;
#15446=CARTESIAN_POINT ( 'NONE',  ( -66.25446545484369665, -88.46443007703511796, 21.65063509461101532 ) ) ;
#15447=CIRCLE ( 'NONE', #16056, 1.500000000000000888 ) ;
#15448=CARTESIAN_POINT ( 'NONE',  ( 7.819480696678551723, -76.71494066083772623, 21.65063509461100821 ) ) ;
#15449=CARTESIAN_POINT ( 'NONE',  ( 2.881217619910392269, -77.49823995525089515, 12.99038105676660493 ) ) ;
#15450=DIRECTION ( 'NONE',  ( -0.9876526153536336894, -0.1566598588826349503, 0.000000000000000000 ) ) ;
#15451=ORIENTED_EDGE ( 'NONE', *, *, #4019, .F. ) ;
#15452=FACE_OUTER_BOUND ( 'NONE', #16504, .T. ) ;
#15453=FACE_BOUND ( 'NONE', #4602, .T. ) ;
#15454=ADVANCED_FACE ( 'NONE', ( #11087 ), #15271, .F. ) ;
#15455=CIRCLE ( 'NONE', #6068, 1.499999999999999556 ) ;
#15457=AXIS2_PLACEMENT_3D ( 'NONE', #5178, #3918, #15405 ) ;
#15458=ORIENTED_EDGE ( 'NONE', *, *, #13722, .F. ) ;
#15459=DIRECTION ( 'NONE',  ( -0.9876526153536341335, -0.1566598588826327021, 0.000000000000000000 ) ) ;
#15460=ORIENTED_EDGE ( 'NONE', *, *, #2556, .T. ) ;
#15461=VERTEX_POINT ( 'NONE', #3785 ) ;
#15462=CIRCLE ( 'NONE', #7307, 1.499999999999999556 ) ;
#15463=DIRECTION ( 'NONE',  ( -0.1566598588826321192, 0.9876526153536342445, 7.798540720466730171E-17 ) ) ;
#15464=VECTOR ( 'NONE', #16465, 1000.000000000000000 ) ;
#15465=FACE_BOUND ( 'NONE', #12947, .T. ) ;
#15466=CARTESIAN_POINT ( 'NONE',  ( -28.26947477390680774, -24.73384407370567217, 8.660254037844417496 ) ) ;
#15467=EDGE_LOOP ( 'NONE', ( #12188, #9714, #8942, #541 ) ) ;
#15469=DIRECTION ( 'NONE',  ( -0.000000000000000000, -0.000000000000000000, -1.000000000000000000 ) ) ;
#15470=ORIENTED_EDGE ( 'NONE', *, *, #13023, .T. ) ;
#15471=CARTESIAN_POINT ( 'NONE',  ( 2.841582609732560272, -19.79905851890276836, -8.660254037844383745 ) ) ;
#15472=EDGE_CURVE ( 'NONE', #537, #10340, #13842, .T. ) ;
#15473=DIRECTION ( 'NONE',  ( 0.000000000000000000, 0.000000000000000000, 1.000000000000000000 ) ) ;
#15475=CARTESIAN_POINT ( 'NONE',  ( -44.07191661956487394, -27.24040181582776299, 12.99038105676661736 ) ) ;
#15476=ORIENTED_EDGE ( 'NONE', *, *, #18751, .F. ) ;
#15478=EDGE_CURVE ( 'NONE', #1662, #1326, #7563, .T. ) ;
#15479=CARTESIAN_POINT ( 'NONE',  ( -56.37793930130739994, -86.89783148820880854, 21.65063509461101532 ) ) ;
#15480=CARTESIAN_POINT ( 'NONE',  ( -49.95819730150881099, -85.87954240547166762, -12.99038105676658539 ) ) ;
#15481=CIRCLE ( 'NONE', #13048, 1.499999999999999556 ) ;
#15482=ORIENTED_EDGE ( 'NONE', *, *, #18102, .T. ) ;
#15484=DIRECTION ( 'NONE',  ( -0.9876526153536341335, -0.1566598588826327021, 0.000000000000000000 ) ) ;
#15485=CARTESIAN_POINT ( 'NONE',  ( -70.24471092643608472, -31.39188807621751209, -4.330127018922181215 ) ) ;
#15486=EDGE_CURVE ( 'NONE', #4436, #18590, #2118, .T. ) ;
#15487=AXIS2_PLACEMENT_3D ( 'NONE', #11967, #1605, #7742 ) ;
#15488=CIRCLE ( 'NONE', #15187, 1.500000000000000888 ) ;
#15489=LINE ( 'NONE', #14056, #9427 ) ;
#15490=AXIS2_PLACEMENT_3D ( 'NONE', #7034, #12781, #18626 ) ;
#15491=DIRECTION ( 'NONE',  ( -0.1566598588826321192, 0.9876526153536342445, 7.798540720466731404E-17 ) ) ;
#15492=DIRECTION ( 'NONE',  ( -0.1566598588826321192, 0.9876526153536342445, 7.798540720466730171E-17 ) ) ;
#15493=DIRECTION ( 'NONE',  ( -0.1566598588826321192, 0.9876526153536342445, 7.798540720466730171E-17 ) ) ;
#15496=DIRECTION ( 'NONE',  ( -0.1566598588826321192, 0.9876526153536342445, 7.798540720466730171E-17 ) ) ;
#15497=DIRECTION ( 'NONE',  ( -0.9876526153536341335, -0.1566598588826327021, 0.000000000000000000 ) ) ;
#15498=DIRECTION ( 'NONE',  ( -0.9876526153536341335, -0.1566598588826327021, 0.000000000000000000 ) ) ;
#15499=MECHANICAL_DESIGN_GEOMETRIC_PRESENTATION_REPRESENTATION('',(#13069),#16118);
#15502=ORIENTED_EDGE ( 'NONE', *, *, #10161, .F. ) ;
#15503=CARTESIAN_POINT ( 'NONE',  ( -46.50141314777110324, -85.33123289938248490, 4.330127018922213189 ) ) ;
#15505=EDGE_LOOP ( 'NONE', ( #12568, #5703 ) ) ;
#15506=AXIS2_PLACEMENT_3D ( 'NONE', #8403, #3738, #12371 ) ;
#15508=EDGE_LOOP ( 'NONE', ( #10691, #11221 ) ) ;
#15509=CARTESIAN_POINT ( 'NONE',  ( -8.516422466834198346, -21.60064689605303911, 8.660254037844413944 ) ) ;
#15510=EDGE_CURVE ( 'NONE', #15004, #13436, #7983, .T. ) ;
#15511=VERTEX_POINT ( 'NONE', #16727 ) ;
#15512=DIRECTION ( 'NONE',  ( 0.000000000000000000, 0.000000000000000000, 1.000000000000000000 ) ) ;
#15515=CYLINDRICAL_SURFACE ( 'NONE', #5836, 1.500000000000001554 ) ;
#15516=SURFACE_STYLE_FILL_AREA ( #943 ) ;
#15518=CARTESIAN_POINT ( 'NONE',  ( -24.27922930231443743, -81.80638607452326028, -17.32050807568878525 ) ) ;
#15519=CARTESIAN_POINT ( 'NONE',  ( -9.299721761247353058, -16.66238381928489787, 17.32050807568881368 ) ) ;
#15520=LINE ( 'NONE', #3837, #16889 ) ;
#15521=ORIENTED_EDGE ( 'NONE', *, *, #2967, .F. ) ;
#15522=CARTESIAN_POINT ( 'NONE',  ( -26.58364252993588650, -19.40393134973095357, -4.330127018922180326 ) ) ;
#15524=ORIENTED_EDGE ( 'NONE', *, *, #8539, .F. ) ;
#15525=EDGE_CURVE ( 'NONE', #10629, #18301, #1240, .T. ) ;
#15526=EDGE_CURVE ( 'NONE', #12710, #14627, #18361, .T. ) ;
#15528=EDGE_LOOP ( 'NONE', ( #17589, #3446 ) ) ;
#15529=EDGE_CURVE ( 'NONE', #15709, #5881, #13296, .T. ) ;
#15530=CIRCLE ( 'NONE', #5856, 1.500000000000001332 ) ;
#15531=EDGE_CURVE ( 'NONE', #13656, #12208, #15731, .T. ) ;
#15532=CARTESIAN_POINT ( 'NONE',  ( -19.38060123572413218, -23.32390534376198232, -4.330127018922181215 ) ) ;
#15533=EDGE_LOOP ( 'NONE', ( #756, #4859, #471, #16298 ) ) ;
#15534=DIRECTION ( 'NONE',  ( 0.000000000000000000, 0.000000000000000000, 1.000000000000000000 ) ) ;
#15538=CARTESIAN_POINT ( 'NONE',  ( -56.37793930130741415, -86.89783148820879433, 4.330127018922213189 ) ) ;
#15540=CYLINDRICAL_SURFACE ( 'NONE', #17354, 1.500000000000001554 ) ;
#15541=CARTESIAN_POINT ( 'NONE',  ( -21.84973277410820458, -23.71555499096855613, 17.32050807568881723 ) ) ;
#15543=ORIENTED_EDGE ( 'NONE', *, *, #13553, .T. ) ;
#15544=EDGE_CURVE ( 'NONE', #14684, #1532, #9975, .T. ) ;
#15545=FACE_OUTER_BOUND ( 'NONE', #17394, .T. ) ;
#15546=ORIENTED_EDGE ( 'NONE', *, *, #3716, .F. ) ;
#15548=CARTESIAN_POINT ( 'NONE',  ( -20.82244514857674389, -81.25807656843406335, -8.660254037844385522 ) ) ;
#15549=FACE_BOUND ( 'NONE', #377, .T. ) ;
#15550=EDGE_CURVE ( 'NONE', #7797, #3315, #2288, .T. ) ;
#15552=DIRECTION ( 'NONE',  ( 0.000000000000000000, 0.000000000000000000, 1.000000000000000000 ) ) ;
#15553=CARTESIAN_POINT ( 'NONE',  ( 0.4120860815263194254, -77.88988960245745830, -17.32050807568878525 ) ) ;
#15555=CARTESIAN_POINT ( 'NONE',  ( -50.45202360918564466, -85.95787233491300583, -8.660254037844385522 ) ) ;
#15556=VERTEX_POINT ( 'NONE', #701 ) ;
#15557=DIRECTION ( 'NONE',  ( -0.1566598588826321192, 0.9876526153536342445, 7.798540720466730171E-17 ) ) ;
#15559=DIRECTION ( 'NONE',  ( -0.1566598588826321192, 0.9876526153536342445, 7.798540720466730171E-17 ) ) ;
#15560=DIRECTION ( 'NONE',  ( -0.1566598588826321192, 0.9876526153536342445, 7.798540720466731404E-17 ) ) ;
#15561=CARTESIAN_POINT ( 'NONE',  ( -3.578159390066044665, -20.81734760163988440, 17.32050807568881012 ) ) ;
#15562=EDGE_LOOP ( 'NONE', ( #9531, #15818, #735, #5069 ) ) ;
#15563=ORIENTED_EDGE ( 'NONE', *, *, #5189, .T. ) ;
#15564=EDGE_LOOP ( 'NONE', ( #3245, #8112, #2437, #13162 ) ) ;
#15565=DIRECTION ( 'NONE',  ( -0.1566598588826321192, 0.9876526153536342445, 7.798540720466730171E-17 ) ) ;
#15566=ORIENTED_EDGE ( 'NONE', *, *, #9783, .F. ) ;
#15567=ORIENTED_EDGE ( 'NONE', *, *, #2432, .T. ) ;
#15569=EDGE_CURVE ( 'NONE', #1993, #8675, #18061, .T. ) ;
#15570=DIRECTION ( 'NONE',  ( -0.1566598588826321192, 0.9876526153536342445, 7.798540720466730171E-17 ) ) ;
#15571=EDGE_LOOP ( 'NONE', ( #15607, #17555 ) ) ;
#15572=EDGE_CURVE ( 'NONE', #11621, #5655, #3603, .T. ) ;
#15576=FACE_OUTER_BOUND ( 'NONE', #10739, .T. ) ;
#15577=ORIENTED_EDGE ( 'NONE', *, *, #6391, .T. ) ;
#15580=ORIENTED_EDGE ( 'NONE', *, *, #7358, .T. ) ;
#15581=ORIENTED_EDGE ( 'NONE', *, *, #6335, .F. ) ;
#15582=DIRECTION ( 'NONE',  ( -0.1566598588826321470, 0.9876526153536342445, 0.000000000000000000 ) ) ;
#15583=LINE ( 'NONE', #10937, #1849 ) ;
#15585=CYLINDRICAL_SURFACE ( 'NONE', #301, 1.500000000000001554 ) ;
#15586=ORIENTED_EDGE ( 'NONE', *, *, #15486, .T. ) ;
#15587=DIRECTION ( 'NONE',  ( -0.1566598588826321192, 0.9876526153536342445, 7.798540720466730171E-17 ) ) ;
#15588=VECTOR ( 'NONE', #15212, 1000.000000000000000 ) ;
#15589=CARTESIAN_POINT ( 'NONE',  ( -62.13913668266656032, -25.04368626950569876, 1.926565525561698076E-14 ) ) ;
#15590=ORIENTED_EDGE ( 'NONE', *, *, #7249, .T. ) ;
#15591=CYLINDRICAL_SURFACE ( 'NONE', #3047, 1.500000000000000666 ) ;
#15592=ADVANCED_FACE ( 'NONE', ( #5137 ), #10144, .F. ) ;
#15593=CARTESIAN_POINT ( 'NONE',  ( 55.85952145814821534, 6.938893903907228378E-15, 92.77853496600735639 ) ) ;
#15594=FACE_OUTER_BOUND ( 'NONE', #7486, .T. ) ;
#15595=( NAMED_UNIT ( * ) SI_UNIT ( $, .STERADIAN. ) SOLID_ANGLE_UNIT ( ) );
#15597=FACE_OUTER_BOUND ( 'NONE', #18281, .T. ) ;
#15598=FACE_OUTER_BOUND ( 'NONE', #1504, .T. ) ;
#15599=ADVANCED_FACE ( 'NONE', ( #4372 ), #6964, .F. ) ;
#15600=DIRECTION ( 'NONE',  ( -0.1566598588826321192, 0.9876526153536342445, 7.798540720466731404E-17 ) ) ;
#15602=ORIENTED_EDGE ( 'NONE', *, *, #14660, .F. ) ;
#15604=DIRECTION ( 'NONE',  ( -0.1566598588826321192, 0.9876526153536342445, 7.798540720466730171E-17 ) ) ;
#15605=ORIENTED_EDGE ( 'NONE', *, *, #11422, .F. ) ;
#15606=LINE ( 'NONE', #8417, #7882 ) ;
#15607=ORIENTED_EDGE ( 'NONE', *, *, #11571, .T. ) ;
#15608=VERTEX_POINT ( 'NONE', #9790 ) ;
#15609=ORIENTED_EDGE ( 'NONE', *, *, #11792, .T. ) ;
#15613=CARTESIAN_POINT ( 'NONE',  ( -33.99103714508810725, -20.57888029135068919, -8.660254037844380193 ) ) ;
#15614=AXIS2_PLACEMENT_3D ( 'NONE', #10034, #94, #12960 ) ;
#15616=DIRECTION ( 'NONE',  ( -0.1566598588826321192, 0.9876526153536342445, 7.798540720466730171E-17 ) ) ;
#15617=ADVANCED_FACE ( 'NONE', ( #12604 ), #4284, .F. ) ;
#15618=ADVANCED_FACE ( 'NONE', ( #11188 ), #15933, .F. ) ;
#15619=CARTESIAN_POINT ( 'NONE',  ( -48.02252708097940825, -27.86704125135830523, 1.869203119972154228E-14 ) ) ;
#15624=AXIS2_PLACEMENT_3D ( 'NONE', #10794, #12721, #8085 ) ;
#15625=ORIENTED_EDGE ( 'NONE', *, *, #9575, .T. ) ;
#15627=ORIENTED_EDGE ( 'NONE', *, *, #9439, .F. ) ;
#15629=AXIS2_PLACEMENT_3D ( 'NONE', #11323, #18611, #14188 ) ;
#15630=EDGE_LOOP ( 'NONE', ( #6511, #9691, #1603, #2190 ) ) ;
#15631=ORIENTED_EDGE ( 'NONE', *, *, #18277, .T. ) ;
#15632=DIRECTION ( 'NONE',  ( -0.1566598588826321747, 0.9876526153536343555, 0.000000000000000000 ) ) ;
#15633=DIRECTION ( 'NONE',  ( -0.1566598588826321192, 0.9876526153536342445, 7.798540720466731404E-17 ) ) ;
#15634=VECTOR ( 'NONE', #1324, 1000.000000000000000 ) ;
#15636=CARTESIAN_POINT ( 'NONE',  ( -42.55080268635659735, -84.70459346385193555, -17.32050807568878525 ) ) ;
#15637=EDGE_LOOP ( 'NONE', ( #4267, #907, #18196, #4840 ) ) ;
#15638=EDGE_CURVE ( 'NONE', #17453, #4620, #629, .T. ) ;
#15639=ADVANCED_FACE ( 'NONE', ( #4075 ), #14039, .F. ) ;
#15640=AXIS2_PLACEMENT_3D ( 'NONE', #16844, #7922, #13680 ) ;
#15641=ORIENTED_EDGE ( 'NONE', *, *, #16806, .T. ) ;
#15642=ORIENTED_EDGE ( 'NONE', *, *, #1444, .F. ) ;
#15643=FACE_OUTER_BOUND ( 'NONE', #7129, .T. ) ;
#15644=DIRECTION ( 'NONE',  ( -0.1566598588826321192, 0.9876526153536342445, 7.798540720466730171E-17 ) ) ;
#15645=CARTESIAN_POINT ( 'NONE',  ( 6.831828081324923474, -76.87160051972034580, -8.660254037844389075 ) ) ;
#15646=AXIS2_PLACEMENT_3D ( 'NONE', #5201, #3747, #12088 ) ;
#15647=CARTESIAN_POINT ( 'NONE',  ( -39.09401853261887538, -84.15628395776273862, 8.660254037844412167 ) ) ;
#15648=VERTEX_POINT ( 'NONE', #9871 ) ;
#15649=ORIENTED_EDGE ( 'NONE', *, *, #10295, .T. ) ;
#15650=ORIENTED_EDGE ( 'NONE', *, *, #5158, .T. ) ;
#15652=CYLINDRICAL_SURFACE ( 'NONE', #12435, 1.500000000000001554 ) ;
#15653=VERTEX_POINT ( 'NONE', #18460 ) ;
#15654=EDGE_LOOP ( 'NONE', ( #6947, #6959, #1333, #18138 ) ) ;
#15655=DIRECTION ( 'NONE',  ( -0.1566598588826321192, 0.9876526153536342445, 7.798540720466731404E-17 ) ) ;
#15656=AXIS2_PLACEMENT_3D ( 'NONE', #622, #12145, #16163 ) ;
#15658=DIRECTION ( 'NONE',  ( -0.1566598588826321192, 0.9876526153536342445, 7.798540720466730171E-17 ) ) ;
#15659=DIRECTION ( 'NONE',  ( 0.000000000000000000, 0.000000000000000000, 1.000000000000000000 ) ) ;
#15660=DIRECTION ( 'NONE',  ( 0.000000000000000000, 0.000000000000000000, 1.000000000000000000 ) ) ;
#15663=VERTEX_POINT ( 'NONE', #17012 ) ;
#15664=DIRECTION ( 'NONE',  ( -0.1566598588826321747, 0.9876526153536343555, 0.000000000000000000 ) ) ;
#15665=CARTESIAN_POINT ( 'NONE',  ( -1.892327146095121204, -15.48743487766515337, 21.65063509461101532 ) ) ;
#15666=ORIENTED_EDGE ( 'NONE', *, *, #2102, .T. ) ;
#15667=EDGE_CURVE ( 'NONE', #7992, #3794, #12709, .T. ) ;
#15668=CIRCLE ( 'NONE', #1461, 1.499999999999999556 ) ;
#15669=DIRECTION ( 'NONE',  ( -0.9876526153536336894, -0.1566598588826350336, 0.000000000000000000 ) ) ;
#15671=ORIENTED_EDGE ( 'NONE', *, *, #3770, .F. ) ;
#15672=EDGE_CURVE ( 'NONE', #12329, #9759, #3924, .T. ) ;
#15675=CARTESIAN_POINT ( 'NONE',  ( -66.25446545484369665, -88.46443007703511796, 4.330127018922213189 ) ) ;
#15676=VERTEX_POINT ( 'NONE', #14241 ) ;
#15678=EDGE_CURVE ( 'NONE', #8415, #8214, #17389, .T. ) ;
#15679=DIRECTION ( 'NONE',  ( -0.9876526153536341335, -0.1566598588826327021, 0.000000000000000000 ) ) ;
#15680=EDGE_LOOP ( 'NONE', ( #10221, #14116, #8079, #16295 ) ) ;
#15683=VERTEX_POINT ( 'NONE', #1088 ) ;
#15684=CYLINDRICAL_SURFACE ( 'NONE', #2757, 1.500000000000001554 ) ;
#15685=VECTOR ( 'NONE', #2796, 1000.000000000000000 ) ;
#15686=VECTOR ( 'NONE', #9872, 1000.000000000000000 ) ;
#15687=LINE ( 'NONE', #12747, #12387 ) ;
#15688=AXIS2_PLACEMENT_3D ( 'NONE', #9176, #3273, #8970 ) ;
#15689=DIRECTION ( 'NONE',  ( 0.000000000000000000, 0.000000000000000000, 1.000000000000000000 ) ) ;
#15691=DIRECTION ( 'NONE',  ( -0.1566598588826321192, 0.9876526153536342445, 7.798540720466730171E-17 ) ) ;
#15692=VERTEX_POINT ( 'NONE', #17198 ) ;
#15694=CIRCLE ( 'NONE', #7534, 1.500000000000000888 ) ;
#15695=DIRECTION ( 'NONE',  ( 0.000000000000000000, 0.000000000000000000, 1.000000000000000000 ) ) ;
#15697=VECTOR ( 'NONE', #5690, 1000.000000000000000 ) ;
#15698=DIRECTION ( 'NONE',  ( 0.000000000000000000, 0.000000000000000000, 1.000000000000000000 ) ) ;
#15700=CARTESIAN_POINT ( 'NONE',  ( -41.60278508118080509, -26.84875216862118918, -8.660254037844380193 ) ) ;
#15702=CARTESIAN_POINT ( 'NONE',  ( -41.56315007100295844, -84.54793360496931598, -4.330127018922185655 ) ) ;
#15703=VERTEX_POINT ( 'NONE', #1279 ) ;
#15704=ORIENTED_EDGE ( 'NONE', *, *, #444, .F. ) ;
#15706=CARTESIAN_POINT ( 'NONE',  ( -15.39035576413176187, -80.39644734457957043, 4.330127018922213189 ) ) ;
#15707=DIRECTION ( 'NONE',  ( -0.1566598588826321747, 0.9876526153536343555, 0.000000000000000000 ) ) ;
#15708=EDGE_LOOP ( 'NONE', ( #10429, #12798 ) ) ;
#15709=VERTEX_POINT ( 'NONE', #5821 ) ;
#15710=AXIS2_PLACEMENT_3D ( 'NONE', #4261, #17554, #6163 ) ;
#15711=AXIS2_PLACEMENT_3D ( 'NONE', #3970, #16994, #8444 ) ;
#15712=CARTESIAN_POINT ( 'NONE',  ( -79.24244631363546887, 32.81909429640987952, -24.99999999999999289 ) ) ;
#15713=ADVANCED_FACE ( 'NONE', ( #6861 ), #8362, .F. ) ;
#15715=DIRECTION ( 'NONE',  ( 0.000000000000000000, 0.000000000000000000, 1.000000000000000000 ) ) ;
#15716=AXIS2_PLACEMENT_3D ( 'NONE', #6502, #9233, #4680 ) ;
#15718=AXIS2_PLACEMENT_3D ( 'NONE', #4902, #10596, #3467 ) ;
#15719=CIRCLE ( 'NONE', #8463, 1.500000000000000888 ) ;
#15721=CARTESIAN_POINT ( 'NONE',  ( -1.109027851681966492, -20.42569795443330349, -4.330127018922184767 ) ) ;
#15722=CARTESIAN_POINT ( 'NONE',  ( -19.17624791478365864, -18.22898240811121795, 1.908195823574487804E-14 ) ) ;
#15723=DIRECTION ( 'NONE',  ( -0.9876526153536336894, -0.1566598588826349503, 0.000000000000000000 ) ) ;
#15724=CARTESIAN_POINT ( 'NONE',  ( -18.18859529943003750, -18.07232254922858061, -12.99038105676658006 ) ) ;
#15725=EDGE_LOOP ( 'NONE', ( #3091, #11459 ) ) ;
#15726=CARTESIAN_POINT ( 'NONE',  ( -34.68921677370541090, -25.75213315644277046, 8.660254037844417496 ) ) ;
#15727=AXIS2_PLACEMENT_3D ( 'NONE', #1030, #15582, #1114 ) ;
#15729=DIRECTION ( 'NONE',  ( -0.9876526153536336894, -0.1566598588826349503, 0.000000000000000000 ) ) ;
#15730=ORIENTED_EDGE ( 'NONE', *, *, #1297, .F. ) ;
#15731=CIRCLE ( 'NONE', #18194, 1.499999999999999556 ) ;
#15733=ORIENTED_EDGE ( 'NONE', *, *, #5834, .T. ) ;
#15734=ORIENTED_EDGE ( 'NONE', *, *, #1444, .T. ) ;
#15735=AXIS2_PLACEMENT_3D ( 'NONE', #11301, #15496, #2511 ) ;
#15737=CYLINDRICAL_SURFACE ( 'NONE', #9366, 1.500000000000001554 ) ;
#15738=ADVANCED_FACE ( 'NONE', ( #11284 ), #17103, .F. ) ;
#15739=CIRCLE ( 'NONE', #16671, 1.500000000000000888 ) ;
#15740=ORIENTED_EDGE ( 'NONE', *, *, #17349, .F. ) ;
#15741=ORIENTED_EDGE ( 'NONE', *, *, #10008, .T. ) ;
#15743=EDGE_LOOP ( 'NONE', ( #13256, #11851, #7177, #1596 ) ) ;
#15744=ORIENTED_EDGE ( 'NONE', *, *, #516, .T. ) ;
#15745=CARTESIAN_POINT ( 'NONE',  ( -81.73462711737164454, 33.01666666666666572, 35.00000000000000000 ) ) ;
#15746=EDGE_CURVE ( 'NONE', #12681, #12642, #7296, .T. ) ;
#15747=AXIS2_PLACEMENT_3D ( 'NONE', #8243, #14010, #1059 ) ;
#15748=ORIENTED_EDGE ( 'NONE', *, *, #5128, .F. ) ;
#15750=CIRCLE ( 'NONE', #12087, 1.500000000000001332 ) ;
#15751=EDGE_LOOP ( 'NONE', ( #4885, #16042, #2322, #4061 ) ) ;
#15752=VECTOR ( 'NONE', #15084, 1000.000000000000000 ) ;
#15753=AXIS2_PLACEMENT_3D ( 'NONE', #15479, #16825, #11095 ) ;
#15754=ORIENTED_EDGE ( 'NONE', *, *, #15922, .T. ) ;
#15755=DIRECTION ( 'NONE',  ( -0.1566598588826321747, 0.9876526153536343555, 0.000000000000000000 ) ) ;
#15756=DIRECTION ( 'NONE',  ( -0.1566598588826321192, 0.9876526153536342445, 7.798540720466730171E-17 ) ) ;
#15757=DIRECTION ( 'NONE',  ( -0.9876526153536336894, -0.1566598588826349503, 0.000000000000000000 ) ) ;
#15758=CARTESIAN_POINT ( 'NONE',  ( -61.31620237807555895, -87.68113078262194904, -12.99038105676658539 ) ) ;
#15759=CIRCLE ( 'NONE', #17595, 1.500000000000000888 ) ;
#15760=CARTESIAN_POINT ( 'NONE',  ( 0.000000000000000000, 0.000000000000000000, 30.00000000000000000 ) ) ;
#15761=VECTOR ( 'NONE', #641, 1000.000000000000000 ) ;
#15763=ORIENTED_EDGE ( 'NONE', *, *, #8569, .T. ) ;
#15764=EDGE_LOOP ( 'NONE', ( #12773, #5247 ) ) ;
#15765=EDGE_LOOP ( 'NONE', ( #14540, #15125 ) ) ;
#15766=DIRECTION ( 'NONE',  ( -0.9876526153536344665, -0.1566598588826304539, 0.000000000000000000 ) ) ;
#15767=ADVANCED_FACE ( 'NONE', ( #3464 ), #18021, .F. ) ;
#15768=EDGE_CURVE ( 'NONE', #15396, #2115, #3621, .T. ) ;
#15769=ORIENTED_EDGE ( 'NONE', *, *, #8250, .T. ) ;
#15771=FACE_BOUND ( 'NONE', #7114, .T. ) ;
#15772=EDGE_CURVE ( 'NONE', #11102, #7929, #14247, .T. ) ;
#15773=AXIS2_PLACEMENT_3D ( 'NONE', #6900, #12469, #13988 ) ;
#15774=LINE ( 'NONE', #14537, #7855 ) ;
#15775=LINE ( 'NONE', #8580, #13037 ) ;
#15776=VECTOR ( 'NONE', #6892, 1000.000000000000000 ) ;
#15777=CARTESIAN_POINT ( 'NONE',  ( -25.59598991458226536, -19.24727149084832689, 17.32050807568881723 ) ) ;
#15778=DIRECTION ( 'NONE',  ( 0.000000000000000000, 0.000000000000000000, 1.000000000000000000 ) ) ;
#15780=AXIS2_PLACEMENT_3D ( 'NONE', #8080, #6496, #2213 ) ;
#15781=CYLINDRICAL_SURFACE ( 'NONE', #13604, 1.500000000000001554 ) ;
#15782=DIRECTION ( 'NONE',  ( -0.9876526153536336894, -0.1566598588826349503, 0.000000000000000000 ) ) ;
#15783=DIRECTION ( 'NONE',  ( -0.1566598588826321192, 0.9876526153536342445, 7.798540720466730171E-17 ) ) ;
#15786=VERTEX_POINT ( 'NONE', #6449 ) ;
#15787=FACE_BOUND ( 'NONE', #2614, .T. ) ;
#15788=DIRECTION ( 'NONE',  ( 0.000000000000000000, 0.000000000000000000, 1.000000000000000000 ) ) ;
#15791=VECTOR ( 'NONE', #547, 1000.000000000000000 ) ;
#15792=ADVANCED_FACE ( 'NONE', ( #12275 ), #5897, .F. ) ;
#15793=ORIENTED_EDGE ( 'NONE', *, *, #2364, .F. ) ;
#15794=DIRECTION ( 'NONE',  ( -0.1566598588826321747, 0.9876526153536343555, 0.000000000000000000 ) ) ;
#15795=AXIS2_PLACEMENT_3D ( 'NONE', #18530, #17162, #6832 ) ;
#15796=CARTESIAN_POINT ( 'NONE',  ( -73.49714175923330117, -26.84527464665596597, 17.32050807568882078 ) ) ;
#15797=DIRECTION ( 'NONE',  ( -0.1566598588826321192, 0.9876526153536342445, 7.798540720466730171E-17 ) ) ;
#15799=AXIS2_PLACEMENT_3D ( 'NONE', #6175, #13249, #16128 ) ;
#15800=DIRECTION ( 'NONE',  ( -0.9876526153536341335, -0.1566598588826327021, 0.000000000000000000 ) ) ;
#15801=CARTESIAN_POINT ( 'NONE',  ( -44.56574292724172182, -27.31873174526908699, -8.660254037844380193 ) ) ;
#15802=FACE_OUTER_BOUND ( 'NONE', #1779, .T. ) ;
#15803=CARTESIAN_POINT ( 'NONE',  ( -27.57129514528951120, -19.56059120861359091, 1.926565525561698076E-14 ) ) ;
#15805=ORIENTED_EDGE ( 'NONE', *, *, #526, .F. ) ;
#15806=AXIS2_PLACEMENT_3D ( 'NONE', #5527, #11280, #15364 ) ;
#15807=DIRECTION ( 'NONE',  ( -0.1566598588826321192, 0.9876526153536342445, 7.798540720466730171E-17 ) ) ;
#15809=CARTESIAN_POINT ( 'NONE',  ( -2.590506774712424853, -20.66068774275724707, -21.65063509461098334 ) ) ;
#15811=CARTESIAN_POINT ( 'NONE',  ( -8.476787456656362352, -79.29982833240114815, -12.99038105676658539 ) ) ;
#15813=VECTOR ( 'NONE', #13995, 1000.000000000000000 ) ;
#15817=FACE_OUTER_BOUND ( 'NONE', #15275, .T. ) ;
#15818=ORIENTED_EDGE ( 'NONE', *, *, #2782, .T. ) ;
#15819=ORIENTED_EDGE ( 'NONE', *, *, #51, .T. ) ;
#15820=DIRECTION ( 'NONE',  ( -0.1566598588826321192, 0.9876526153536342445, 7.798540720466731404E-17 ) ) ;
#15821=EDGE_CURVE ( 'NONE', #3794, #7992, #9712, .T. ) ;
#15822=ORIENTED_EDGE ( 'NONE', *, *, #6884, .F. ) ;
#15823=CARTESIAN_POINT ( 'NONE',  ( -67.77557938805200877, -31.00023842901093118, -17.32050807568878170 ) ) ;
#15824=CIRCLE ( 'NONE', #1607, 1.500000000000000888 ) ;
#15825=DIRECTION ( 'NONE',  ( 0.000000000000000000, 0.000000000000000000, 1.000000000000000000 ) ) ;
#15827=DIRECTION ( 'NONE',  ( -0.9876526153536341335, -0.1566598588826327021, 0.000000000000000000 ) ) ;
#15828=CARTESIAN_POINT ( 'NONE',  ( -6.007655918272284623, -78.90817868519457079, -17.32050807568878525 ) ) ;
#15829=EDGE_CURVE ( 'NONE', #10552, #8596, #4459, .T. ) ;
#15831=CARTESIAN_POINT ( 'NONE',  ( -3.373806069125576901, -15.72242466598909871, 21.65063509461101177 ) ) ;
#15832=VERTEX_POINT ( 'NONE', #10857 ) ;
#15833=EDGE_LOOP ( 'NONE', ( #2392, #7128 ) ) ;
#15834=CARTESIAN_POINT ( 'NONE',  ( -56.37793930130741415, -86.89783148820879433, 4.330127018922213189 ) ) ;
#15835=AXIS2_PLACEMENT_3D ( 'NONE', #14688, #11823, #9275 ) ;
#15836=VERTEX_POINT ( 'NONE', #18115 ) ;
#15837=EDGE_LOOP ( 'NONE', ( #9976, #17839, #6278, #14478 ) ) ;
#15838=ORIENTED_EDGE ( 'NONE', *, *, #12610, .T. ) ;
#15839=DIRECTION ( 'NONE',  ( -0.1566598588826321747, 0.9876526153536343555, 0.000000000000000000 ) ) ;
#15840=FACE_BOUND ( 'NONE', #4369, .T. ) ;
#15843=EDGE_CURVE ( 'NONE', #6040, #227, #4979, .T. ) ;
#15844=DIRECTION ( 'NONE',  ( -0.1566598588826321192, 0.9876526153536342445, 7.798540720466730171E-17 ) ) ;
#15845=DIRECTION ( 'NONE',  ( -0.9876526153536336894, -0.1566598588826349503, 0.000000000000000000 ) ) ;
#15846=CARTESIAN_POINT ( 'NONE',  ( -20.65772683781411345, -18.46397219643516507, 1.908195823574487804E-14 ) ) ;
#15847=EDGE_CURVE ( 'NONE', #8275, #4130, #3033, .T. ) ;
#15851=ORIENTED_EDGE ( 'NONE', *, *, #6942, .F. ) ;
#15852=ORIENTED_EDGE ( 'NONE', *, *, #17465, .T. ) ;
#15853=CARTESIAN_POINT ( 'NONE',  ( -26.58364252993588650, -19.40393134973095357, -12.99038105676658006 ) ) ;
#15854=VECTOR ( 'NONE', #7941, 1000.000000000000000 ) ;
#15855=VERTEX_POINT ( 'NONE', #10683 ) ;
#15856=FACE_BOUND ( 'NONE', #7033, .T. ) ;
#15857=CARTESIAN_POINT ( 'NONE',  ( -64.77298653181324539, -88.22944028871114597, -21.65063509461098690 ) ) ;
#15858=ORIENTED_EDGE ( 'NONE', *, *, #18283, .F. ) ;
#15859=CARTESIAN_POINT ( 'NONE',  ( -7.528769851480577202, -21.44398703717040888, -21.65063509461098334 ) ) ;
#15861=DIRECTION ( 'NONE',  ( 0.000000000000000000, 0.000000000000000000, 1.000000000000000000 ) ) ;
#15862=DIRECTION ( 'NONE',  ( -0.9876526153536336894, -0.1566598588826349503, 0.000000000000000000 ) ) ;
#15863=ORIENTED_EDGE ( 'NONE', *, *, #4673, .T. ) ;
#15864=EDGE_CURVE ( 'NONE', #9857, #5108, #10240, .T. ) ;
#15865=EDGE_CURVE ( 'NONE', #17419, #9271, #6065, .T. ) ;
#15866=CARTESIAN_POINT ( 'NONE',  ( -51.27495791377661760, -23.32042782179675200, 12.99038105676661736 ) ) ;
#15869=EDGE_CURVE ( 'NONE', #7505, #9397, #17597, .T. ) ;
#15870=CARTESIAN_POINT ( 'NONE',  ( -50.45202360918563045, -85.95787233491302004, 17.32050807568881368 ) ) ;
#15871=ORIENTED_EDGE ( 'NONE', *, *, #9984, .F. ) ;
#15872=EDGE_LOOP ( 'NONE', ( #12967, #6332, #1370, #5924 ) ) ;
#15873=FACE_OUTER_BOUND ( 'NONE', #14602, .T. ) ;
#15874=ORIENTED_EDGE ( 'NONE', *, *, #14068, .F. ) ;
#15875=LINE ( 'NONE', #10362, #3524 ) ;
#15876=FACE_OUTER_BOUND ( 'NONE', #12609, .T. ) ;
#15877=ORIENTED_EDGE ( 'NONE', *, *, #2193, .F. ) ;
#15878=DIRECTION ( 'NONE',  ( -0.9876526153536336894, -0.1566598588826349503, 0.000000000000000000 ) ) ;
#15880=CIRCLE ( 'NONE', #1373, 1.500000000000000444 ) ;
#15882=CARTESIAN_POINT ( 'NONE',  ( -9.464440072009985272, -79.45648819128378193, 8.660254037844412167 ) ) ;
#15884=ORIENTED_EDGE ( 'NONE', *, *, #10112, .F. ) ;
#15886=CARTESIAN_POINT ( 'NONE',  ( -6.995308533625909320, -79.06483854407720457, -21.65063509461098690 ) ) ;
#15887=ORIENTED_EDGE ( 'NONE', *, *, #13198, .F. ) ;
#15889=DIRECTION ( 'NONE',  ( -0.9876526153536336894, -0.1566598588826349503, 0.000000000000000000 ) ) ;
#15892=CARTESIAN_POINT ( 'NONE',  ( -44.85521591397803576, -22.30213873905963951, -12.99038105676658006 ) ) ;
#15893=CARTESIAN_POINT ( 'NONE',  ( 8.807133312032172867, -76.55828080195509244, -8.660254037844389075 ) ) ;
#15894=ORIENTED_EDGE ( 'NONE', *, *, #9089, .F. ) ;
#15895=CIRCLE ( 'NONE', #8016, 1.500000000000000888 ) ;
#15896=DIRECTION ( 'NONE',  ( -0.1566598588826321192, 0.9876526153536342445, 7.798540720466731404E-17 ) ) ;
#15897=VERTEX_POINT ( 'NONE', #8735 ) ;
#15898=ORIENTED_EDGE ( 'NONE', *, *, #5061, .F. ) ;
#15899=DIRECTION ( 'NONE',  ( -0.1566598588826321192, 0.9876526153536342445, 7.798540720466730171E-17 ) ) ;
#15901=DIRECTION ( 'NONE',  ( -0.9876526153536336894, -0.1566598588826349503, 0.000000000000000000 ) ) ;
#15903=CARTESIAN_POINT ( 'NONE',  ( -7.982961148979534016, -79.22149840295983836, 8.660254037844412167 ) ) ;
#15905=FACE_OUTER_BOUND ( 'NONE', #5123, .T. ) ;
#15906=VECTOR ( 'NONE', #18063, 1000.000000000000114 ) ;
#15907=VERTEX_POINT ( 'NONE', #13091 ) ;
#15909=DIRECTION ( 'NONE',  ( -0.1566598588826321192, 0.9876526153536342445, 7.798540720466730171E-17 ) ) ;
#15912=VERTEX_POINT ( 'NONE', #10593 ) ;
#15913=EDGE_CURVE ( 'NONE', #16881, #2, #117, .T. ) ;
#15914=ORIENTED_EDGE ( 'NONE', *, *, #15155, .T. ) ;
#15916=ADVANCED_FACE ( 'NONE', ( #661 ), #12185, .F. ) ;
#15917=CARTESIAN_POINT ( 'NONE',  ( -31.68662391746665463, -82.98133501614300656, 21.65063509461101532 ) ) ;
#15918=AXIS2_PLACEMENT_3D ( 'NONE', #7133, #17377, #4360 ) ;
#15919=ORIENTED_EDGE ( 'NONE', *, *, #990, .F. ) ;
#15920=VERTEX_POINT ( 'NONE', #2539 ) ;
#15921=DIRECTION ( 'NONE',  ( -0.1566598588826321747, 0.9876526153536343555, 0.000000000000000000 ) ) ;
#15922=EDGE_CURVE ( 'NONE', #2300, #7880, #13012, .T. ) ;
#15924=CARTESIAN_POINT ( 'NONE',  ( -80.30645961545690170, -27.92535762103354458, 25.00000000000001776 ) ) ;
#15925=DIRECTION ( 'NONE',  ( -0.1566598588826321192, 0.9876526153536342445, 7.798540720466731404E-17 ) ) ;
#15927=DIRECTION ( 'NONE',  ( -0.9876526153536336894, -0.1566598588826349503, 0.000000000000000000 ) ) ;
#15928=VERTEX_POINT ( 'NONE', #5200 ) ;
#15929=VERTEX_POINT ( 'NONE', #18322 ) ;
#15930=CARTESIAN_POINT ( 'NONE',  ( -59.67000514428247016, -24.65203662229912851, 21.65063509461101887 ) ) ;
#15931=DIRECTION ( 'NONE',  ( 0.000000000000000000, 0.000000000000000000, 1.000000000000000000 ) ) ;
#15933=CYLINDRICAL_SURFACE ( 'NONE', #15145, 1.500000000000001554 ) ;
#15934=DIRECTION ( 'NONE',  ( -0.1566598588826321192, 0.9876526153536342445, 7.798540720466730171E-17 ) ) ;
#15935=FACE_BOUND ( 'NONE', #18235, .T. ) ;
#15937=DIRECTION ( 'NONE',  ( -0.1566598588826321192, 0.9876526153536342445, 7.798540720466731404E-17 ) ) ;
#15939=ORIENTED_EDGE ( 'NONE', *, *, #2406, .F. ) ;
#15941=CARTESIAN_POINT ( 'NONE',  ( -9.504075082187826595, -21.75730675493566579, -12.99038105676658006 ) ) ;
#15942=AXIS2_PLACEMENT_3D ( 'NONE', #5798, #4532, #14406 ) ;
#15943=CIRCLE ( 'NONE', #12596, 1.500000000000000444 ) ;
#15944=EDGE_CURVE ( 'NONE', #1139, #9239, #3660, .T. ) ;
#15945=ORIENTED_EDGE ( 'NONE', *, *, #12361, .F. ) ;
#15946=CARTESIAN_POINT ( 'NONE',  ( -76.66445292623467367, -32.41017715895461038, -21.65063509461098334 ) ) ;
#15947=CARTESIAN_POINT ( 'NONE',  ( -40.61513246582718040, -26.69209230973856251, 21.65063509461101887 ) ) ;
#15948=ORIENTED_EDGE ( 'NONE', *, *, #9203, .T. ) ;
#15949=CIRCLE ( 'NONE', #15333, 1.500000000000000000 ) ;
#15950=EDGE_CURVE ( 'NONE', #18110, #15929, #2735, .T. ) ;
#15952=EDGE_CURVE ( 'NONE', #2545, #10257, #15750, .T. ) ;
#15953=VECTOR ( 'NONE', #4696, 1000.000000000000000 ) ;
#15955=EDGE_LOOP ( 'NONE', ( #7631, #5238 ) ) ;
#15956=VECTOR ( 'NONE', #13901, 1000.000000000000000 ) ;
#15957=DIRECTION ( 'NONE',  ( -0.1566598588826321192, 0.9876526153536342445, 7.798540720466730171E-17 ) ) ;
#15958=CYLINDRICAL_SURFACE ( 'NONE', #6294, 1.500000000000000888 ) ;
#15960=DIRECTION ( 'NONE',  ( -0.1566598588826321192, 0.9876526153536342445, 7.798540720466730171E-17 ) ) ;
#15961=CARTESIAN_POINT ( 'NONE',  ( -29.25712738926042888, -24.89050393258829175, -4.330127018922181215 ) ) ;
#15962=EDGE_LOOP ( 'NONE', ( #8268, #8923, #5136, #2369 ) ) ;
#15963=EDGE_LOOP ( 'NONE', ( #14786, #7852 ) ) ;
#15964=CARTESIAN_POINT ( 'NONE',  ( -47.98289207080156871, -85.56622268770641426, -21.65063509461098690 ) ) ;
#15966=AXIS2_PLACEMENT_3D ( 'NONE', #1989, #4826, #18137 ) ;
#15967=CARTESIAN_POINT ( 'NONE',  ( -53.74408945216070776, -23.71207746900332936, 8.660254037844417496 ) ) ;
#15969=EDGE_CURVE ( 'NONE', #17353, #7282, #8412, .T. ) ;
#15970=VERTEX_POINT ( 'NONE', #9550 ) ;
#15972=AXIS2_PLACEMENT_3D ( 'NONE', #14645, #6116, #4312 ) ;
#15973=EDGE_CURVE ( 'NONE', #17742, #14531, #4841, .T. ) ;
#15976=DIRECTION ( 'NONE',  ( -0.000000000000000000, -0.000000000000000000, -1.000000000000000000 ) ) ;
#15977=CIRCLE ( 'NONE', #6312, 1.500000000000001332 ) ;
#15978=DIRECTION ( 'NONE',  ( -0.1566598588826321747, 0.9876526153536343555, 0.000000000000000000 ) ) ;
#15979=DIRECTION ( 'NONE',  ( 1.000000000000000000, 0.000000000000000000, 0.000000000000000000 ) ) ;
#15980=CARTESIAN_POINT ( 'NONE',  ( -25.76070822534488869, -82.04137586284721806, 17.32050807568881368 ) ) ;
#15983=CARTESIAN_POINT ( 'NONE',  ( -45.55339554259534651, -27.47539160415172432, -21.65063509461098334 ) ) ;
#15984=AXIS2_PLACEMENT_3D ( 'NONE', #11806, #95, #8898 ) ;
#15985=DIRECTION ( 'NONE',  ( 0.000000000000000000, 0.000000000000000000, 1.000000000000000000 ) ) ;
#15986=ORIENTED_EDGE ( 'NONE', *, *, #11578, .F. ) ;
#15987=CIRCLE ( 'NONE', #12336, 1.499999999999999556 ) ;
#15988=CIRCLE ( 'NONE', #4816, 1.500000000000000888 ) ;
#15990=ORIENTED_EDGE ( 'NONE', *, *, #11786, .F. ) ;
#15991=EDGE_CURVE ( 'NONE', #6871, #1617, #11485, .T. ) ;
#15993=ADVANCED_FACE ( 'NONE', ( #12380 ), #18225, .F. ) ;
#15994=ADVANCED_FACE ( 'NONE', ( #16784 ), #3745, .F. ) ;
#15995=DIRECTION ( 'NONE',  ( -0.1566598588826321747, 0.9876526153536343555, 0.000000000000000000 ) ) ;
#15996=CARTESIAN_POINT ( 'NONE',  ( -51.43967622453926936, -86.11453219379562540, -21.65063509461098690 ) ) ;
#15999=DIRECTION ( 'NONE',  ( -0.9876526153536336894, -0.1566598588826349503, 0.000000000000000000 ) ) ;
#16001=AXIS2_PLACEMENT_3D ( 'NONE', #12783, #8343, #8435 ) ;
#16003=AXIS2_PLACEMENT_3D ( 'NONE', #5531, #11089, #11285 ) ;
#16005=FACE_BOUND ( 'NONE', #14551, .T. ) ;
#16006=DIRECTION ( 'NONE',  ( -0.9876526153536341335, -0.1566598588826327021, 0.000000000000000000 ) ) ;
#16007=FACE_OUTER_BOUND ( 'NONE', #14961, .T. ) ;
#16008=DIRECTION ( 'NONE',  ( -0.1566598588826321747, 0.9876526153536343555, 0.000000000000000000 ) ) ;
#16009=ORIENTED_EDGE ( 'NONE', *, *, #4726, .F. ) ;
#16010=CLOSED_SHELL ( 'NONE', ( #10661, #8680, #16284, #11153, #3352, #15792, #18649, #9415, #2800, #10343, #6407, #6330, #8353, #873, #10065, #761, #12644, #7661, #2888, #3790, #12919, #13057, #3219, #9788, #9134, #15738, #2313, #12241, #5065, #13390, #12946, #2214, #18677, #17320, #6613, #14682, #16756, #1302, #3475, #2309, #2867, #17376, #13588, #16574, #18702, #12419, #17510, #11662, #9694, #5408, #13885, #10202, #5895, #10318, #7579, #16751, #5565, #9631, #6750, #16995, #12096, #2887, #16528, #18406, #17413, #1630, #2308, #1803, #1910, #809, #18072, #4066, #9357, #18349, #8894, #11994, #12566, #5564, #3951, #6610, #8681, #201, #18159, #5155, #18354, #6671, #18026, #9724, #12496, #10315, #333, #12732, #4085, #2685, #11720, #16225, #6503, #14194, #10048, #7918, #3333, #16813, #10135, #13530, #17895, #16139, #10369, #8315, #5360, #16341, #4704, #7374, #6880, #5029, #1418, #12381, #10911, #1973, #10916, #14124, #18380, #11973, #15617, #3084, #10550, #2334, #4348, #4835, #18550, #15227, #10388, #1273, #16643, #9829, #11828, #17407, #16578, #17519, #1379, #14396, #15618, #5583, #7252, #5162, #12860, #17551, #12021, #4779, #4056, #8998, #1281, #16939, #9744, #18774, #17070, #11942, #8445, #7430, #8698, #4388, #10687, #6444, #6834, #7466, #17920, #18230, #8987, #7380, #13457, #12386, #6167, #754, #7740, #7810, #2665, #9171, #14452, #2103, #14589, #3164, #8093, #6730, #10726, #16976, #414, #9645, #15993, #11235, #6564, #17296, #933, #11091, #4552, #9981, #5000, #15130, #16477, #9092, #1669, #7386, #7618, #7203, #14536, #9718, #9980, #14610, #459, #10765, #15592, #4147, #17264, #600, #12265, #7096, #1604, #6471, #9624, #4499, #3932, #11550, #14311, #10620, #11455, #9326, #10182, #13911, #12995, #6086, #1854, #12932, #8632, #1584, #3403, #7812, #17751, #4204, #18419, #900, #2936, #3740, #106, #3312, #12996, #15767, #3964, #6062, #6147, #12024, #4599, #5900, #3472, #10763, #10527, #579, #14243, #8416, #4146, #15599, #1327, #2642, #7753, #10111, #15713, #12023, #14724, #12192, #13429, #14023, #6853, #17889, #3248, #14479, #11416, #15209, #15454, #6968, #1954, #4831, #14809, #17167, #4999, #14022, #15033, #3810, #13370, #418, #78, #4, #1051, #12800, #14474, #14653, #11177, #1086, #12376, #16164, #12113, #729, #6387, #8392, #5854, #6410, #5966, #9039, #17315, #15280, #1142, #10587, #6991, #14937, #2939, #3455, #16162, #14960, #1653, #6115, #1112, #17395, #1251, #568, #18097, #11881, #4248, #7126, #16908, #15208, #6050, #8776, #13692, #17691, #16705, #4315, #10504, #3746, #5649, #16379, #2661, #13529, #834, #655, #6264, #11436, #15639, #10236, #15994, #3299, #6590, #10269, #15916, #16502, #11938, #1555, #12679, #9407, #2983, #2913, #17975, #14419, #4121, #12739, #2394, #14609, #2543, #14941, #16609, #17392, #5197, #4953, #6504, #6535, #14476, #1557, #8558, #2945, #17759, #4645, #16858, #8657, #8613, #5674, #16121, #9932, #6608, #4408, #2719 ) ) ;
#16011=ORIENTED_EDGE ( 'NONE', *, *, #7312, .T. ) ;
#16012=DIRECTION ( 'NONE',  ( -0.9876526153536341335, -0.1566598588826327021, 0.000000000000000000 ) ) ;
#16014=VECTOR ( 'NONE', #16423, 1000.000000000000000 ) ;
#16015=EDGE_LOOP ( 'NONE', ( #3132, #1866, #17560, #7695 ) ) ;
#16017=ORIENTED_EDGE ( 'NONE', *, *, #1826, .F. ) ;
#16018=LINE ( 'NONE', #472, #2629 ) ;
#16019=AXIS2_PLACEMENT_3D ( 'NONE', #3461, #18109, #5075 ) ;
#16020=AXIS2_PLACEMENT_3D ( 'NONE', #5085, #7950, #749 ) ;
#16021=FACE_BOUND ( 'NONE', #12983, .T. ) ;
#16022=ORIENTED_EDGE ( 'NONE', *, *, #2289, .F. ) ;
#16023=DIRECTION ( 'NONE',  ( 0.000000000000000000, 0.000000000000000000, 1.000000000000000000 ) ) ;
#16025=AXIS2_PLACEMENT_3D ( 'NONE', #12901, #4193, #8747 ) ;
#16026=EDGE_CURVE ( 'NONE', #9148, #1188, #18548, .T. ) ;
#16027=AXIS2_PLACEMENT_3D ( 'NONE', #5317, #11072, #16900 ) ;
#16028=CARTESIAN_POINT ( 'NONE',  ( -81.73462711737164454, 33.01666666666666572, -35.00000000000000000 ) ) ;
#16029=ORIENTED_EDGE ( 'NONE', *, *, #2102, .F. ) ;
#16030=FACE_BOUND ( 'NONE', #4519, .T. ) ;
#16031=CIRCLE ( 'NONE', #12394, 1.500000000000000888 ) ;
#16032=VERTEX_POINT ( 'NONE', #15892 ) ;
#16033=CARTESIAN_POINT ( 'NONE',  ( -39.09401853261888959, -84.15628395776272441, -8.660254037844385522 ) ) ;
#16036=DIRECTION ( 'NONE',  ( -0.1566598588826321192, 0.9876526153536342445, 7.798540720466731404E-17 ) ) ;
#16037=CARTESIAN_POINT ( 'NONE',  ( -77.65210554158829837, -32.56683701783724416, 17.32050807568881723 ) ) ;
#16038=DIRECTION ( 'NONE',  ( -0.1566598588826321192, 0.9876526153536342445, 7.798540720466731404E-17 ) ) ;
#16039=ORIENTED_EDGE ( 'NONE', *, *, #16522, .F. ) ;
#16041=AXIS2_PLACEMENT_3D ( 'NONE', #12743, #4211, #5753 ) ;
#16042=ORIENTED_EDGE ( 'NONE', *, *, #12362, .F. ) ;
#16043=CARTESIAN_POINT ( 'NONE',  ( -76.17062661855784711, -32.33184722951329348, -17.32050807568878170 ) ) ;
#16044=VERTEX_POINT ( 'NONE', #11688 ) ;
#16045=VECTOR ( 'NONE', #13659, 1000.000000000000000 ) ;
#16048=AXIS2_PLACEMENT_3D ( 'NONE', #18669, #2693, #8856 ) ;
#16049=ORIENTED_EDGE ( 'NONE', *, *, #16965, .F. ) ;
#16052=EDGE_CURVE ( 'NONE', #12090, #12954, #17525, .T. ) ;
#16053=ORIENTED_EDGE ( 'NONE', *, *, #239, .T. ) ;
#16054=DIRECTION ( 'NONE',  ( -0.1566598588826321192, 0.9876526153536342445, 7.798540720466730171E-17 ) ) ;
#16055=FACE_BOUND ( 'NONE', #11335, .T. ) ;
#16056=AXIS2_PLACEMENT_3D ( 'NONE', #9660, #2630, #2454 ) ;
#16057=DIRECTION ( 'NONE',  ( -0.000000000000000000, -0.000000000000000000, -1.000000000000000000 ) ) ;
#16059=CARTESIAN_POINT ( 'NONE',  ( -70.24471092643608472, -31.39188807621751209, 21.65063509461101887 ) ) ;
#16060=AXIS2_PLACEMENT_3D ( 'NONE', #12810, #18736, #5716 ) ;
#16061=CARTESIAN_POINT ( 'NONE',  ( 11.77009115809307715, -76.08830122530719109, 8.660254037844406838 ) ) ;
#16063=AXIS2_PLACEMENT_3D ( 'NONE', #5529, #14240, #11640 ) ;
#16064=VERTEX_POINT ( 'NONE', #16089 ) ;
#16065=VERTEX_POINT ( 'NONE', #15700 ) ;
#16066=DIRECTION ( 'NONE',  ( -0.1566598588826321192, 0.9876526153536342445, 7.798540720466730171E-17 ) ) ;
#16067=AXIS2_PLACEMENT_3D ( 'NONE', #3541, #6516, #10940 ) ;
#16068=VERTEX_POINT ( 'NONE', #3089 ) ;
#16069=EDGE_CURVE ( 'NONE', #11171, #7553, #8784, .T. ) ;
#16070=CARTESIAN_POINT ( 'NONE',  ( -8.312069145893737243, -16.50572396040226053, -12.99038105676658006 ) ) ;
#16071=CARTESIAN_POINT ( 'NONE',  ( -45.51376053241747144, -85.17457304049985112, 17.32050807568881368 ) ) ;
#16072=EDGE_LOOP ( 'NONE', ( #18175, #1698 ) ) ;
#16073=FACE_OUTER_BOUND ( 'NONE', #1368, .T. ) ;
#16074=AXIS2_PLACEMENT_3D ( 'NONE', #1851, #431, #10279 ) ;
#16075=AXIS2_PLACEMENT_3D ( 'NONE', #14003, #2625, #1234 ) ;
#16076=CARTESIAN_POINT ( 'NONE',  ( -53.74408945216070776, -23.71207746900332936, 8.660254037844417496 ) ) ;
#16077=DIRECTION ( 'NONE',  ( 1.000000000000000000, 0.000000000000000000, -0.000000000000000000 ) ) ;
#16078=CARTESIAN_POINT ( 'NONE',  ( -66.08974714408108753, -25.67032570503621614, -12.99038105676658006 ) ) ;
#16080=AXIS2_PLACEMENT_3D ( 'NONE', #16855, #15409, #12359 ) ;
#16081=EDGE_CURVE ( 'NONE', #5805, #9632, #2989, .T. ) ;
#16082=CARTESIAN_POINT ( 'NONE',  ( -58.84707083969148300, -87.28948113541537168, 1.424741226644455312E-14 ) ) ;
#16083=CARTESIAN_POINT ( 'NONE',  ( 55.85952145814821534, 6.938893903907228378E-15, -30.00000000000000000 ) ) ;
#16086=CARTESIAN_POINT ( 'NONE',  ( 3.868870235264020963, -77.34158009636824715, 17.32050807568880657 ) ) ;
#16087=VERTEX_POINT ( 'NONE', #14469 ) ;
#16088=ORIENTED_EDGE ( 'NONE', *, *, #6709, .T. ) ;
#16089=CARTESIAN_POINT ( 'NONE',  ( -61.84966369593023927, -30.06027927571514624, -12.99038105676658006 ) ) ;
#16090=VERTEX_POINT ( 'NONE', #7196 ) ;
#16091=EDGE_CURVE ( 'NONE', #8605, #17569, #3642, .T. ) ;
#16092=CIRCLE ( 'NONE', #1893, 1.500000000000001332 ) ;
#16093=DIRECTION ( 'NONE',  ( -0.1566598588826321192, 0.9876526153536342445, 7.798540720466730171E-17 ) ) ;
#16095=EDGE_LOOP ( 'NONE', ( #6541, #12688 ) ) ;
#16096=CIRCLE ( 'NONE', #18567, 1.500000000000000888 ) ;
#16097=ORIENTED_EDGE ( 'NONE', *, *, #1083, .T. ) ;
#16098=CARTESIAN_POINT ( 'NONE',  ( -23.12685837619818940, -18.85562184364173532, -21.65063509461098334 ) ) ;
#16099=CIRCLE ( 'NONE', #4878, 1.499999999999999556 ) ;
#16100=DIRECTION ( 'NONE',  ( 1.000000000000000000, 0.000000000000000000, 0.000000000000000000 ) ) ;
#16103=CARTESIAN_POINT ( 'NONE',  ( -0.4108482230646692823, -15.25244508934120802, 21.65063509461101177 ) ) ;
#16104=DIRECTION ( 'NONE',  ( -0.1566598588826321192, 0.9876526153536342445, 7.798540720466730171E-17 ) ) ;
#16105=CARTESIAN_POINT ( 'NONE',  ( -38.14600092744311155, -26.30044266253198160, -17.32050807568878170 ) ) ;
#16106=CIRCLE ( 'NONE', #11245, 1.500000000000001332 ) ;
#16109=CARTESIAN_POINT ( 'NONE',  ( -70.24471092643608472, -31.39188807621751209, 12.99038105676661736 ) ) ;
#16111=EDGE_CURVE ( 'NONE', #356, #14582, #8803, .T. ) ;
#16112=DIRECTION ( 'NONE',  ( -0.9876526153536336894, -0.1566598588826350336, 0.000000000000000000 ) ) ;
#16114=EDGE_CURVE ( 'NONE', #3127, #2423, #11502, .T. ) ;
#16115=DIRECTION ( 'NONE',  ( -0.1566598588826321192, 0.9876526153536342445, 7.798540720466730171E-17 ) ) ;
#16116=ORIENTED_EDGE ( 'NONE', *, *, #7027, .T. ) ;
#16117=EDGE_CURVE ( 'NONE', #4398, #3127, #14297, .T. ) ;
#16118=( GEOMETRIC_REPRESENTATION_CONTEXT ( 3 ) GLOBAL_UNCERTAINTY_ASSIGNED_CONTEXT ( ( #9278 ) ) GLOBAL_UNIT_ASSIGNED_CONTEXT ( ( #681, #8628, #975 ) ) REPRESENTATION_CONTEXT ( 'NONE', 'WORKASPACE' ) );
#16119=ORIENTED_EDGE ( 'NONE', *, *, #6436, .T. ) ;
#16120=CYLINDRICAL_SURFACE ( 'NONE', #5041, 1.500000000000001554 ) ;
#16121=ADVANCED_FACE ( 'NONE', ( #7111 ), #18697, .F. ) ;
#16122=ORIENTED_EDGE ( 'NONE', *, *, #5511, .F. ) ;
#16123=EDGE_CURVE ( 'NONE', #2946, #17353, #16681, .T. ) ;
#16124=ORIENTED_EDGE ( 'NONE', *, *, #1411, .T. ) ;
#16125=ORIENTED_EDGE ( 'NONE', *, *, #4137, .F. ) ;
#16126=CARTESIAN_POINT ( 'NONE',  ( -25.80034323552273179, -24.34219442649909126, 4.330127018922217630 ) ) ;
#16128=DIRECTION ( 'NONE',  ( -0.9876526153536341335, -0.1566598588826327021, 0.000000000000000000 ) ) ;
#16129=CARTESIAN_POINT ( 'NONE',  ( -52.26261052913025651, -23.47708768067938223, 1.926565525561698076E-14 ) ) ;
#16135=CARTESIAN_POINT ( 'NONE',  ( -40.41077914488671041, -21.59716937408778037, 1.214306433183764966E-14 ) ) ;
#16136=CARTESIAN_POINT ( 'NONE',  ( 6.338001773648100468, -76.94993044916168401, 12.99038105676660493 ) ) ;
#16137=EDGE_CURVE ( 'NONE', #6687, #17343, #34, .T. ) ;
#16138=VERTEX_POINT ( 'NONE', #77 ) ;
#16139=ADVANCED_FACE ( 'NONE', ( #5861 ), #4961, .F. ) ;
#16141=ORIENTED_EDGE ( 'NONE', *, *, #10496, .F. ) ;
#16142=ORIENTED_EDGE ( 'NONE', *, *, #4063, .F. ) ;
#16143=FACE_BOUND ( 'NONE', #14644, .T. ) ;
#16144=CARTESIAN_POINT ( 'NONE',  ( -66.08974714408108753, -25.67032570503621969, -4.330127018922180326 ) ) ;
#16145=ORIENTED_EDGE ( 'NONE', *, *, #2192, .F. ) ;
#16146=AXIS2_PLACEMENT_3D ( 'NONE', #5611, #10136, #17187 ) ;
#16147=CYLINDRICAL_SURFACE ( 'NONE', #2712, 1.500000000000001554 ) ;
#16148=ORIENTED_EDGE ( 'NONE', *, *, #12671, .F. ) ;
#16149=ORIENTED_EDGE ( 'NONE', *, *, #9491, .F. ) ;
#16150=CARTESIAN_POINT ( 'NONE',  ( -25.80034323552273179, -24.34219442649909126, -12.99038105676658006 ) ) ;
#16152=DIRECTION ( 'NONE',  ( 0.000000000000000000, 0.000000000000000000, 1.000000000000000000 ) ) ;
#16155=ORIENTED_EDGE ( 'NONE', *, *, #15973, .T. ) ;
#16156=EDGE_LOOP ( 'NONE', ( #17073, #6072 ) ) ;
#16157=AXIS2_PLACEMENT_3D ( 'NONE', #17646, #16383, #16188 ) ;
#16158=FACE_BOUND ( 'NONE', #2266, .T. ) ;
#16159=DIRECTION ( 'NONE',  ( -6.505213034913026604E-17, -0.000000000000000000, 1.000000000000000000 ) ) ;
#16160=EDGE_LOOP ( 'NONE', ( #984, #7908, #7528, #14367 ) ) ;
#16161=CARTESIAN_POINT ( 'NONE',  ( -25.26688191766805858, -81.96304593340589406, 21.65063509461101532 ) ) ;
#16162=ADVANCED_FACE ( 'NONE', ( #14932 ), #10568, .F. ) ;
#16163=DIRECTION ( 'NONE',  ( 1.000000000000000000, 0.000000000000000000, 0.000000000000000000 ) ) ;
#16164=ADVANCED_FACE ( 'NONE', ( #11785 ), #17719, .F. ) ;
#16165=VERTEX_POINT ( 'NONE', #17632 ) ;
#16166=DIRECTION ( 'NONE',  ( -0.1566598588826321192, 0.9876526153536342445, 7.798540720466731404E-17 ) ) ;
#16167=LINE ( 'NONE', #4945, #1788 ) ;
#16168=EDGE_CURVE ( 'NONE', #10248, #1545, #12062, .T. ) ;
#16169=FACE_BOUND ( 'NONE', #2631, .T. ) ;
#16170=LINE ( 'NONE', #14650, #16998 ) ;
#16171=DIRECTION ( 'NONE',  ( -0.9876526153536336894, -0.1566598588826349503, 0.000000000000000000 ) ) ;
#16172=DIRECTION ( 'NONE',  ( -0.9876526153536336894, -0.1566598588826349503, 0.000000000000000000 ) ) ;
#16174=ORIENTED_EDGE ( 'NONE', *, *, #15772, .T. ) ;
#16176=DIRECTION ( 'NONE',  ( -0.1566598588826321192, 0.9876526153536342445, 7.798540720466730171E-17 ) ) ;
#16178=CARTESIAN_POINT ( 'NONE',  ( 2.881217619910392269, -77.49823995525089515, -4.330127018922189208 ) ) ;
#16179=ORIENTED_EDGE ( 'NONE', *, *, #519, .F. ) ;
#16180=ORIENTED_EDGE ( 'NONE', *, *, #17229, .F. ) ;
#16181=CARTESIAN_POINT ( 'NONE',  ( -43.08426400421126345, -27.08374195694514341, -17.32050807568878170 ) ) ;
#16182=ORIENTED_EDGE ( 'NONE', *, *, #13745, .T. ) ;
#16183=ORIENTED_EDGE ( 'NONE', *, *, #4867, .T. ) ;
#16184=EDGE_CURVE ( 'NONE', #18301, #10629, #16693, .T. ) ;
#16185=AXIS2_PLACEMENT_3D ( 'NONE', #13169, #8918, #6380 ) ;
#16186=DIRECTION ( 'NONE',  ( -0.1566598588826321192, 0.9876526153536342445, 7.798540720466730171E-17 ) ) ;
#16187=CYLINDRICAL_SURFACE ( 'NONE', #3953, 1.500000000000001554 ) ;
#16188=DIRECTION ( 'NONE',  ( -0.9876526153536336894, -0.1566598588826349503, 0.000000000000000000 ) ) ;
#16189=ORIENTED_EDGE ( 'NONE', *, *, #4019, .T. ) ;
#16191=CARTESIAN_POINT ( 'NONE',  ( -25.26688191766805858, -81.96304593340589406, 12.99038105676661203 ) ) ;
#16193=CARTESIAN_POINT ( 'NONE',  ( -20.82244514857674389, -81.25807656843406335, 1.424741226644455312E-14 ) ) ;
#16194=EDGE_LOOP ( 'NONE', ( #14166, #2148, #11651, #11729 ) ) ;
#16195=CARTESIAN_POINT ( 'NONE',  ( -5.059638313096497697, -21.05233738996382797, 8.660254037844412167 ) ) ;
#16197=DIRECTION ( 'NONE',  ( -0.9876526153536341335, -0.1566598588826327576, 0.000000000000000000 ) ) ;
#16198=AXIS2_PLACEMENT_3D ( 'NONE', #12935, #7549, #15889 ) ;
#16199=ORIENTED_EDGE ( 'NONE', *, *, #3692, .T. ) ;
#16201=CARTESIAN_POINT ( 'NONE',  ( -61.15148406731293562, -24.88702641062306142, -4.330127018922180326 ) ) ;
#16202=ORIENTED_EDGE ( 'NONE', *, *, #990, .T. ) ;
#16203=ORIENTED_EDGE ( 'NONE', *, *, #11571, .F. ) ;
#16204=DIRECTION ( 'NONE',  ( -0.1566598588826321747, 0.9876526153536343555, 0.000000000000000000 ) ) ;
#16207=EDGE_CURVE ( 'NONE', #592, #1113, #7735, .T. ) ;
#16208=EDGE_CURVE ( 'NONE', #1459, #8907, #951, .T. ) ;
#16209=DIRECTION ( 'NONE',  ( -0.1566598588826321747, 0.9876526153536343555, 0.000000000000000000 ) ) ;
#16210=CIRCLE ( 'NONE', #8937, 1.500000000000000444 ) ;
#16211=CARTESIAN_POINT ( 'NONE',  ( -48.80582637539256297, -22.92877817459016754, 1.908195823574487804E-14 ) ) ;
#16212=EDGE_CURVE ( 'NONE', #14096, #15836, #13633, .T. ) ;
#16213=CARTESIAN_POINT ( 'NONE',  ( -54.73174206751432536, -23.86873732788596669, 12.99038105676661736 ) ) ;
#16214=CARTESIAN_POINT ( 'NONE',  ( -12.46703292824872733, -22.22728633158356359, 12.99038105676661381 ) ) ;
#16215=VERTEX_POINT ( 'NONE', #11960 ) ;
#16216=VERTEX_POINT ( 'NONE', #3444 ) ;
#16217=CIRCLE ( 'NONE', #9254, 1.500000000000000000 ) ;
#16218=DIRECTION ( 'NONE',  ( -0.9876526153536341335, -0.1566598588826327021, 0.000000000000000000 ) ) ;
#16219=LINE ( 'NONE', #11837, #10836 ) ;
#16221=EDGE_LOOP ( 'NONE', ( #13133, #3133 ) ) ;
#16223=EDGE_LOOP ( 'NONE', ( #1208, #18015, #1136, #17480 ) ) ;
#16224=CARTESIAN_POINT ( 'NONE',  ( -24.81269062016911064, -24.18553456761645393, 8.660254037844417496 ) ) ;
#16225=ADVANCED_FACE ( 'NONE', ( #3361 ), #6329, .F. ) ;
#16226=ORIENTED_EDGE ( 'NONE', *, *, #15472, .F. ) ;
#16227=FACE_BOUND ( 'NONE', #247, .T. ) ;
#16228=EDGE_CURVE ( 'NONE', #5860, #14458, #5796, .T. ) ;
#16230=EDGE_CURVE ( 'NONE', #12256, #14223, #1269, .T. ) ;
#16231=EDGE_LOOP ( 'NONE', ( #466, #11611, #9385, #2366 ) ) ;
#16234=CIRCLE ( 'NONE', #15629, 1.500000000000000888 ) ;
#16235=ORIENTED_EDGE ( 'NONE', *, *, #13917, .F. ) ;
#16236=LINE ( 'NONE', #14905, #12696 ) ;
#16237=DIRECTION ( 'NONE',  ( -0.9876526153536341335, -0.1566598588826327021, 0.000000000000000000 ) ) ;
#16238=FACE_OUTER_BOUND ( 'NONE', #1027, .T. ) ;
#16239=LINE ( 'NONE', #9138, #9246 ) ;
#16241=ORIENTED_EDGE ( 'NONE', *, *, #5639, .T. ) ;
#16242=VERTEX_POINT ( 'NONE', #7831 ) ;
#16243=LINE ( 'NONE', #12141, #17527 ) ;
#16244=DIRECTION ( 'NONE',  ( -0.1566598588826321192, 0.9876526153536342445, 7.798540720466731404E-17 ) ) ;
#16246=EDGE_LOOP ( 'NONE', ( #12564, #9470, #10338, #10910 ) ) ;
#16247=CARTESIAN_POINT ( 'NONE',  ( 2.881217619910392269, -77.49823995525089515, 4.330127018922209636 ) ) ;
#16248=ORIENTED_EDGE ( 'NONE', *, *, #5784, .T. ) ;
#16249=AXIS2_PLACEMENT_3D ( 'NONE', #13691, #5185, #10946 ) ;
#16250=AXIS2_PLACEMENT_3D ( 'NONE', #16178, #13317, #18086 ) ;
#16251=CARTESIAN_POINT ( 'NONE',  ( -77.44775222064782838, -27.47191408218649400, 21.65063509461101887 ) ) ;
#16254=CARTESIAN_POINT ( 'NONE',  ( -53.94844277310117064, -28.80700040465408662, 12.99038105676661736 ) ) ;
#16257=ORIENTED_EDGE ( 'NONE', *, *, #14864, .T. ) ;
#16258=EDGE_CURVE ( 'NONE', #3229, #13151, #10740, .T. ) ;
#16259=CARTESIAN_POINT ( 'NONE',  ( -14.23798483801550674, -17.44568311369805969, -8.660254037844380193 ) ) ;
#16260=CIRCLE ( 'NONE', #1447, 1.500000000000000444 ) ;
#16261=CARTESIAN_POINT ( 'NONE',  ( -28.26947477390680774, -24.73384407370567217, -8.660254037844380193 ) ) ;
#16263=AXIS2_PLACEMENT_3D ( 'NONE', #10271, #7270, #4402 ) ;
#16264=CARTESIAN_POINT ( 'NONE',  ( -36.62488699423479943, -83.76463431055617548, 4.330127018922213189 ) ) ;
#16265=ORIENTED_EDGE ( 'NONE', *, *, #1465, .T. ) ;
#16266=DIRECTION ( 'NONE',  ( -0.9876526153536336894, -0.1566598588826349503, 0.000000000000000000 ) ) ;
#16267=ORIENTED_EDGE ( 'NONE', *, *, #7350, .T. ) ;
#16268=AXIS2_PLACEMENT_3D ( 'NONE', #6820, #7112, #5672 ) ;
#16269=DIRECTION ( 'NONE',  ( -0.9876526153536341335, -0.1566598588826327021, 0.000000000000000000 ) ) ;
#16270=ORIENTED_EDGE ( 'NONE', *, *, #18305, .F. ) ;
#16271=DIRECTION ( 'NONE',  ( -0.1566598588826321192, 0.9876526153536342445, 7.798540720466730171E-17 ) ) ;
#16272=AXIS2_PLACEMENT_3D ( 'NONE', #16827, #9510, #9600 ) ;
#16273=EDGE_LOOP ( 'NONE', ( #14994, #7405 ) ) ;
#16275=FACE_OUTER_BOUND ( 'NONE', #12306, .T. ) ;
#16276=DIRECTION ( 'NONE',  ( -0.1566598588826321192, 0.9876526153536342445, 7.798540720466731404E-17 ) ) ;
#16279=VERTEX_POINT ( 'NONE', #16547 ) ;
#16280=CARTESIAN_POINT ( 'NONE',  ( 1.360103686702108128, -20.03404830722672259, -8.660254037844383745 ) ) ;
#16281=CIRCLE ( 'NONE', #18756, 1.499999999999997335 ) ;
#16282=DIRECTION ( 'NONE',  ( -0.1566598588826321192, 0.9876526153536342445, 7.798540720466730171E-17 ) ) ;
#16283=ORIENTED_EDGE ( 'NONE', *, *, #14126, .T. ) ;
#16284=ADVANCED_FACE ( 'NONE', ( #3538 ), #9335, .F. ) ;
#16285=CYLINDRICAL_SURFACE ( 'NONE', #9669, 2.000000000000000000 ) ;
#16286=EDGE_LOOP ( 'NONE', ( #2725, #6867, #2785, #10379 ) ) ;
#16287=CIRCLE ( 'NONE', #9018, 1.500000000000000444 ) ;
#16288=ORIENTED_EDGE ( 'NONE', *, *, #2555, .T. ) ;
#16289=DIRECTION ( 'NONE',  ( -0.1566598588826321192, 0.9876526153536342445, 7.798540720466731404E-17 ) ) ;
#16290=EDGE_LOOP ( 'NONE', ( #17848, #18412, #15020, #11297 ) ) ;
#16293=ORIENTED_EDGE ( 'NONE', *, *, #10855, .T. ) ;
#16295=ORIENTED_EDGE ( 'NONE', *, *, #3055, .F. ) ;
#16297=DIRECTION ( 'NONE',  ( -0.1566598588826321192, 0.9876526153536342445, 7.798540720466730171E-17 ) ) ;
#16298=ORIENTED_EDGE ( 'NONE', *, *, #10643, .T. ) ;
#16299=CIRCLE ( 'NONE', #7231, 2.500000000000002220 ) ;
#16300=DIRECTION ( 'NONE',  ( -0.1566598588826321192, 0.9876526153536342445, 7.798540720466730171E-17 ) ) ;
#16301=DIRECTION ( 'NONE',  ( 0.000000000000000000, 0.000000000000000000, 1.000000000000000000 ) ) ;
#16302=DIRECTION ( 'NONE',  ( -0.1566598588826321192, 0.9876526153536342445, 7.798540720466730171E-17 ) ) ;
#16305=CARTESIAN_POINT ( 'NONE',  ( -9.504075082187823043, -21.75730675493566579, 21.65063509461101177 ) ) ;
#16306=DIRECTION ( 'NONE',  ( -0.1566598588826321192, 0.9876526153536342445, 7.798540720466731404E-17 ) ) ;
#16308=ORIENTED_EDGE ( 'NONE', *, *, #14134, .T. ) ;
#16309=VECTOR ( 'NONE', #14035, 1000.000000000000000 ) ;
#16310=CARTESIAN_POINT ( 'NONE',  ( -2.000000000000000000, 0.000000000000000000, 30.00000000000000000 ) ) ;
#16312=EDGE_CURVE ( 'NONE', #4310, #1682, #18300, .T. ) ;
#16313=CARTESIAN_POINT ( 'NONE',  ( -28.06512145296634486, -19.63892113805490780, 21.65063509461101887 ) ) ;
#16314=CIRCLE ( 'NONE', #17540, 1.500000000000000888 ) ;
#16315=CIRCLE ( 'NONE', #10554, 1.500000000000000000 ) ;
#16316=CARTESIAN_POINT ( 'NONE',  ( -7.982961148979534016, -79.22149840295983836, -17.32050807568878525 ) ) ;
#16319=EDGE_CURVE ( 'NONE', #10598, #1633, #9727, .T. ) ;
#16322=ORIENTED_EDGE ( 'NONE', *, *, #2552, .F. ) ;
#16323=CARTESIAN_POINT ( 'NONE',  ( -68.55887868246516348, -26.06197535224280415, 8.660254037844417496 ) ) ;
#16324=FACE_BOUND ( 'NONE', #6799, .T. ) ;
#16325=VECTOR ( 'NONE', #9268, 1000.000000000000000 ) ;
#16326=CYLINDRICAL_SURFACE ( 'NONE', #7061, 1.500000000000001554 ) ;
#16327=AXIS2_PLACEMENT_3D ( 'NONE', #9007, #6382, #12011 ) ;
#16329=AXIS2_PLACEMENT_3D ( 'NONE', #8684, #7372, #11603 ) ;
#16330=AXIS2_PLACEMENT_3D ( 'NONE', #16362, #1753, #7541 ) ;
#16331=CIRCLE ( 'NONE', #1516, 1.500000000000000888 ) ;
#16332=AXIS2_PLACEMENT_3D ( 'NONE', #11010, #9614, #2407 ) ;
#16334=CARTESIAN_POINT ( 'NONE',  ( -45.55339554259533230, -27.47539160415171722, -4.330127018922181215 ) ) ;
#16335=LINE ( 'NONE', #9133, #2438 ) ;
#16336=CYLINDRICAL_SURFACE ( 'NONE', #15131, 1.500000000000000666 ) ;
#16337=DIRECTION ( 'NONE',  ( 0.000000000000000000, 0.000000000000000000, 1.000000000000000000 ) ) ;
#16338=CIRCLE ( 'NONE', #13304, 1.500000000000000444 ) ;
#16339=DIRECTION ( 'NONE',  ( -0.1566598588826321192, 0.9876526153536342445, 7.798540720466730171E-17 ) ) ;
#16341=ADVANCED_FACE ( 'NONE', ( #13874 ), #16944, .F. ) ;
#16342=FACE_OUTER_BOUND ( 'NONE', #2843, .T. ) ;
#16343=ORIENTED_EDGE ( 'NONE', *, *, #12985, .T. ) ;
#16344=EDGE_LOOP ( 'NONE', ( #13548, #12467 ) ) ;
#16345=CARTESIAN_POINT ( 'NONE',  ( -23.12685837619818940, -18.85562184364174243, -4.330127018922180326 ) ) ;
#16346=EDGE_CURVE ( 'NONE', #6192, #8055, #16390, .T. ) ;
#16347=AXIS2_PLACEMENT_3D ( 'NONE', #5622, #3984, #7145 ) ;
#16349=DIRECTION ( 'NONE',  ( -0.1566598588826321192, 0.9876526153536342445, 7.798540720466730171E-17 ) ) ;
#16350=EDGE_CURVE ( 'NONE', #10352, #14662, #6714, .T. ) ;
#16351=DIRECTION ( 'NONE',  ( -0.1566598588826321192, 0.9876526153536342445, 7.798540720466731404E-17 ) ) ;
#16353=EDGE_CURVE ( 'NONE', #11687, #9583, #6708, .T. ) ;
#16355=AXIS2_PLACEMENT_3D ( 'NONE', #711, #7809, #13571 ) ;
#16356=ORIENTED_EDGE ( 'NONE', *, *, #3117, .F. ) ;
#16357=DIRECTION ( 'NONE',  ( 0.000000000000000000, 0.000000000000000000, 1.000000000000000000 ) ) ;
#16358=FACE_BOUND ( 'NONE', #8915, .T. ) ;
#16359=VECTOR ( 'NONE', #16093, 1000.000000000000000 ) ;
#16360=DIRECTION ( 'NONE',  ( -0.9876526153536341335, -0.1566598588826327021, 0.000000000000000000 ) ) ;
#16362=CARTESIAN_POINT ( 'NONE',  ( -14.23798483801550674, -17.44568311369805613, -17.32050807568878170 ) ) ;
#16363=CIRCLE ( 'NONE', #8190, 1.500000000000000888 ) ;
#16364=CARTESIAN_POINT ( 'NONE',  ( -57.89905323451570496, -29.43363984018461466, 17.32050807568881723 ) ) ;
#16365=AXIS2_PLACEMENT_3D ( 'NONE', #6641, #16414, #10610 ) ;
#16366=DIRECTION ( 'NONE',  ( 0.000000000000000000, 0.000000000000000000, 1.000000000000000000 ) ) ;
#16367=DIRECTION ( 'NONE',  ( -0.1566598588826321192, 0.9876526153536342445, 7.798540720466730171E-17 ) ) ;
#16368=EDGE_CURVE ( 'NONE', #10552, #12139, #13340, .T. ) ;
#16369=ORIENTED_EDGE ( 'NONE', *, *, #16026, .T. ) ;
#16370=EDGE_LOOP ( 'NONE', ( #3612, #8111, #2932, #12353 ) ) ;
#16372=VERTEX_POINT ( 'NONE', #8010 ) ;
#16373=EDGE_LOOP ( 'NONE', ( #4784, #11964, #9891, #3969 ) ) ;
#16374=AXIS2_PLACEMENT_3D ( 'NONE', #5047, #6415, #15013 ) ;
#16375=EDGE_LOOP ( 'NONE', ( #18700, #11047, #2501, #13380 ) ) ;
#16376=VERTEX_POINT ( 'NONE', #5460 ) ;
#16378=EDGE_LOOP ( 'NONE', ( #9252, #232, #6784, #12490 ) ) ;
#16379=ADVANCED_FACE ( 'NONE', ( #821 ), #18491, .F. ) ;
#16380=DIRECTION ( 'NONE',  ( -0.1566598588826321747, 0.9876526153536343555, 0.000000000000000000 ) ) ;
#16382=CARTESIAN_POINT ( 'NONE',  ( -79.23462711737164454, 33.01666666666666572, -35.00000000000000000 ) ) ;
#16383=DIRECTION ( 'NONE',  ( -0.1566598588826321192, 0.9876526153536342445, 7.798540720466730171E-17 ) ) ;
#16384=ORIENTED_EDGE ( 'NONE', *, *, #712, .T. ) ;
#16385=CARTESIAN_POINT ( 'NONE',  ( -14.44233815895597672, -22.54060604934882051, 12.99038105676661381 ) ) ;
#16387=VERTEX_POINT ( 'NONE', #3915 ) ;
#16388=AXIS2_PLACEMENT_3D ( 'NONE', #7818, #15108, #13580 ) ;
#16389=DIRECTION ( 'NONE',  ( -0.9876526153536336894, -0.1566598588826349503, 0.000000000000000000 ) ) ;
#16390=CIRCLE ( 'NONE', #8213, 1.500000000000000444 ) ;
#16391=DIRECTION ( 'NONE',  ( -0.9876526153536341335, -0.1566598588826327576, 0.000000000000000000 ) ) ;
#16392=FACE_BOUND ( 'NONE', #6297, .T. ) ;
#16394=AXIS2_PLACEMENT_3D ( 'NONE', #1009, #11100, #6781 ) ;
#16395=DIRECTION ( 'NONE',  ( -0.1566598588826321747, 0.9876526153536343555, 0.000000000000000000 ) ) ;
#16396=DIRECTION ( 'NONE',  ( -1.000000000000000000, 0.000000000000000000, 0.000000000000000000 ) ) ;
#16397=ORIENTED_EDGE ( 'NONE', *, *, #15392, .T. ) ;
#16398=AXIS2_PLACEMENT_3D ( 'NONE', #16247, #9228, #11868 ) ;
#16399=DIRECTION ( 'NONE',  ( -0.9876526153536336894, -0.1566598588826349503, 0.000000000000000000 ) ) ;
#16400=ORIENTED_EDGE ( 'NONE', *, *, #12246, .F. ) ;
#16401=EDGE_LOOP ( 'NONE', ( #18108, #18160, #6328, #5535 ) ) ;
#16402=EDGE_CURVE ( 'NONE', #4043, #7608, #1031, .T. ) ;
#16403=VECTOR ( 'NONE', #12396, 1000.000000000000000 ) ;
#16404=ORIENTED_EDGE ( 'NONE', *, *, #10746, .F. ) ;
#16405=AXIS2_PLACEMENT_3D ( 'NONE', #4932, #16512, #17777 ) ;
#16406=DIRECTION ( 'NONE',  ( 0.000000000000000000, 0.000000000000000000, 1.000000000000000000 ) ) ;
#16407=EDGE_CURVE ( 'NONE', #8789, #10862, #9114, .T. ) ;
#16408=EDGE_CURVE ( 'NONE', #3308, #15217, #2604, .T. ) ;
#16410=VERTEX_POINT ( 'NONE', #8389 ) ;
#16411=AXIS2_PLACEMENT_3D ( 'NONE', #3179, #10206, #13141 ) ;
#16412=EDGE_CURVE ( 'NONE', #8596, #17674, #12428, .T. ) ;
#16413=CARTESIAN_POINT ( 'NONE',  ( -3.578159390066044665, -20.81734760163988440, 8.660254037844412167 ) ) ;
#16414=DIRECTION ( 'NONE',  ( -0.1566598588826321747, 0.9876526153536343555, 0.000000000000000000 ) ) ;
#16415=FACE_OUTER_BOUND ( 'NONE', #16803, .T. ) ;
#16416=DIRECTION ( 'NONE',  ( -0.1566598588826321192, 0.9876526153536342445, 7.798540720466730171E-17 ) ) ;
#16417=CYLINDRICAL_SURFACE ( 'NONE', #10810, 1.500000000000001554 ) ;
#16418=ORIENTED_EDGE ( 'NONE', *, *, #3610, .F. ) ;
#16420=DIRECTION ( 'NONE',  ( -0.1566598588826321192, 0.9876526153536342445, 7.798540720466730171E-17 ) ) ;
#16421=ORIENTED_EDGE ( 'NONE', *, *, #15048, .T. ) ;
#16422=CARTESIAN_POINT ( 'NONE',  ( -19.87442754340095519, -23.40223527320329922, 1.869203119972154228E-14 ) ) ;
#16423=DIRECTION ( 'NONE',  ( -0.1566598588826321192, 0.9876526153536342445, 7.798540720466730171E-17 ) ) ;
#16424=CIRCLE ( 'NONE', #1597, 2.500000000000002220 ) ;
#16425=ORIENTED_EDGE ( 'NONE', *, *, #13328, .T. ) ;
#16426=ORIENTED_EDGE ( 'NONE', *, *, #9153, .F. ) ;
#16427=ORIENTED_EDGE ( 'NONE', *, *, #11389, .F. ) ;
#16428=CARTESIAN_POINT ( 'NONE',  ( -31.72625892764450484, -25.28215357979487266, 1.887572821959364500E-14 ) ) ;
#16429=ORIENTED_EDGE ( 'NONE', *, *, #8697, .T. ) ;
#16430=FACE_BOUND ( 'NONE', #13727, .T. ) ;
#16433=DIRECTION ( 'NONE',  ( -0.1566598588826321192, 0.9876526153536342445, 7.798540720466730171E-17 ) ) ;
#16434=ORIENTED_EDGE ( 'NONE', *, *, #14732, .F. ) ;
#16436=ORIENTED_EDGE ( 'NONE', *, *, #9066, .F. ) ;
#16437=EDGE_CURVE ( 'NONE', #14246, #3468, #10903, .T. ) ;
#16438=DIRECTION ( 'NONE',  ( -0.1566598588826321747, 0.9876526153536343555, 0.000000000000000000 ) ) ;
#16440=FACE_OUTER_BOUND ( 'NONE', #3189, .T. ) ;
#16444=VERTEX_POINT ( 'NONE', #9813 ) ;
#16445=ORIENTED_EDGE ( 'NONE', *, *, #16916, .T. ) ;
#16446=FACE_OUTER_BOUND ( 'NONE', #14910, .T. ) ;
#16447=CARTESIAN_POINT ( 'NONE',  ( -30.04042668367358360, -19.95224085582017892, 21.65063509461101887 ) ) ;
#16448=AXIS2_PLACEMENT_3D ( 'NONE', #11552, #18645, #7055 ) ;
#16449=EDGE_LOOP ( 'NONE', ( #1033, #7993 ) ) ;
#16450=LINE ( 'NONE', #17792, #18252 ) ;
#16452=CARTESIAN_POINT ( 'NONE',  ( -14.23798483801550674, -17.44568311369805969, -8.660254037844380193 ) ) ;
#16453=EDGE_CURVE ( 'NONE', #5727, #6686, #15583, .T. ) ;
#16454=CARTESIAN_POINT ( 'NONE',  ( -46.33669483700847280, -22.53712852738359018, 4.330127018922218518 ) ) ;
#16457=EDGE_CURVE ( 'NONE', #3665, #13180, #4271, .T. ) ;
#16458=ORIENTED_EDGE ( 'NONE', *, *, #4968, .T. ) ;
#16459=VECTOR ( 'NONE', #11528, 1000.000000000000000 ) ;
#16460=DIRECTION ( 'NONE',  ( 0.000000000000000000, 0.000000000000000000, 1.000000000000000000 ) ) ;
#16461=CARTESIAN_POINT ( 'NONE',  ( -70.04035760549561473, -26.29696514056674417, -8.660254037844380193 ) ) ;
#16463=ORIENTED_EDGE ( 'NONE', *, *, #12771, .F. ) ;
#16464=ORIENTED_EDGE ( 'NONE', *, *, #14687, .F. ) ;
#16465=DIRECTION ( 'NONE',  ( -0.1566598588826321192, 0.9876526153536342445, 7.798540720466730171E-17 ) ) ;
#16466=ORIENTED_EDGE ( 'NONE', *, *, #15162, .T. ) ;
#16467=ORIENTED_EDGE ( 'NONE', *, *, #7027, .F. ) ;
#16468=ORIENTED_EDGE ( 'NONE', *, *, #8355, .T. ) ;
#16469=DIRECTION ( 'NONE',  ( -0.1566598588826321747, 0.9876526153536343555, 0.000000000000000000 ) ) ;
#16470=EDGE_LOOP ( 'NONE', ( #6499, #3783 ) ) ;
#16471=DIRECTION ( 'NONE',  ( -0.1566598588826321192, 0.9876526153536342445, 7.798540720466730171E-17 ) ) ;
#16472=EDGE_CURVE ( 'NONE', #8310, #626, #13556, .T. ) ;
#16473=FACE_OUTER_BOUND ( 'NONE', #4291, .T. ) ;
#16475=ORIENTED_EDGE ( 'NONE', *, *, #11572, .T. ) ;
#16477=ADVANCED_FACE ( 'NONE', ( #11493 ), #1211, .T. ) ;
#16478=FACE_OUTER_BOUND ( 'NONE', #823, .T. ) ;
#16479=CARTESIAN_POINT ( 'NONE',  ( -21.64537945316773460, -18.62063205531779531, -12.99038105676658006 ) ) ;
#16480=CARTESIAN_POINT ( 'NONE',  ( -34.15575545585073058, -83.37298466334958391, 1.424741226644455312E-14 ) ) ;
#16481=DIRECTION ( 'NONE',  ( -0.1566598588826321192, 0.9876526153536342445, 7.798540720466730171E-17 ) ) ;
#16482=FACE_OUTER_BOUND ( 'NONE', #17499, .T. ) ;
#16484=DIRECTION ( 'NONE',  ( -0.1566598588826321192, 0.9876526153536342445, 7.798540720466730171E-17 ) ) ;
#16486=EDGE_LOOP ( 'NONE', ( #2676, #17294, #14570, #15769 ) ) ;
#16487=EDGE_LOOP ( 'NONE', ( #9025, #7132 ) ) ;
#16490=ORIENTED_EDGE ( 'NONE', *, *, #15672, .T. ) ;
#16491=DIRECTION ( 'NONE',  ( -0.1566598588826321192, 0.9876526153536342445, 7.798540720466731404E-17 ) ) ;
#16493=CARTESIAN_POINT ( 'NONE',  ( -57.69469991357524208, -24.33871690453384318, -21.65063509461098334 ) ) ;
#16494=VECTOR ( 'NONE', #14189, 1000.000000000000000 ) ;
#16495=DIRECTION ( 'NONE',  ( -0.1566598588826321747, 0.9876526153536343555, 0.000000000000000000 ) ) ;
#16497=EDGE_CURVE ( 'NONE', #2286, #11293, #11590, .T. ) ;
#16499=SURFACE_SIDE_STYLE ('',( #16595 ) ) ;
#16501=PLANE ( 'NONE',  #1213 ) ;
#16502=ADVANCED_FACE ( 'NONE', ( #57 ), #13018, .F. ) ;
#16503=ORIENTED_EDGE ( 'NONE', *, *, #13562, .T. ) ;
#16504=EDGE_LOOP ( 'NONE', ( #1353, #13515, #8631, #881 ) ) ;
#16505=ORIENTED_EDGE ( 'NONE', *, *, #2850, .F. ) ;
#16506=VERTEX_POINT ( 'NONE', #14552 ) ;
#16507=CARTESIAN_POINT ( 'NONE',  ( -53.74408945216072198, -23.71207746900331870, -17.32050807568878170 ) ) ;
#16508=VERTEX_POINT ( 'NONE', #11308 ) ;
#16509=CIRCLE ( 'NONE', #1665, 1.500000000000001332 ) ;
#16510=FACE_BOUND ( 'NONE', #5540, .T. ) ;
#16511=CYLINDRICAL_SURFACE ( 'NONE', #5227, 1.500000000000000888 ) ;
#16512=DIRECTION ( 'NONE',  ( -0.1566598588826321747, 0.9876526153536343555, 0.000000000000000000 ) ) ;
#16513=DIRECTION ( 'NONE',  ( -0.1566598588826321192, 0.9876526153536342445, 7.798540720466730171E-17 ) ) ;
#16515=DIRECTION ( 'NONE',  ( 0.000000000000000000, 0.000000000000000000, 1.000000000000000000 ) ) ;
#16516=DIRECTION ( 'NONE',  ( -0.1566598588826321192, 0.9876526153536342445, 7.798540720466731404E-17 ) ) ;
#16518=DIRECTION ( 'NONE',  ( -0.1566598588826321192, 0.9876526153536342445, 7.798540720466730171E-17 ) ) ;
#16519=ORIENTED_EDGE ( 'NONE', *, *, #12594, .T. ) ;
#16520=EDGE_LOOP ( 'NONE', ( #18094, #17007, #14861, #7698 ) ) ;
#16521=FACE_OUTER_BOUND ( 'NONE', #11915, .T. ) ;
#16522=EDGE_CURVE ( 'NONE', #9759, #12329, #12953, .T. ) ;
#16523=DIRECTION ( 'NONE',  ( -0.9876526153536336894, -0.1566598588826349503, 0.000000000000000000 ) ) ;
#16525=AXIS2_PLACEMENT_3D ( 'NONE', #6006, #4394, #8754 ) ;
#16526=ORIENTED_EDGE ( 'NONE', *, *, #4314, .F. ) ;
#16527=CARTESIAN_POINT ( 'NONE',  ( 2.447859171744382056, -14.79900155049411659, 30.00000000000000000 ) ) ;
#16528=ADVANCED_FACE ( 'NONE', ( #5746 ), #3071, .F. ) ;
#16529=CARTESIAN_POINT ( 'NONE',  ( -0.4108482230646692823, -15.25244508934120802, 12.99038105676661026 ) ) ;
#16531=ORIENTED_EDGE ( 'NONE', *, *, #2244, .F. ) ;
#16532=CIRCLE ( 'NONE', #1997, 1.500000000000000888 ) ;
#16533=EDGE_CURVE ( 'NONE', #15443, #4155, #2806, .T. ) ;
#16534=DIRECTION ( 'NONE',  ( -0.9876526153536336894, -0.1566598588826349503, 0.000000000000000000 ) ) ;
#16535=DIRECTION ( 'NONE',  ( 0.000000000000000000, 0.000000000000000000, 1.000000000000000000 ) ) ;
#16536=CARTESIAN_POINT ( 'NONE',  ( -74.19532138785061193, -32.01852751174804013, -17.32050807568878170 ) ) ;
#16538=ORIENTED_EDGE ( 'NONE', *, *, #14752, .F. ) ;
#16539=AXIS2_PLACEMENT_3D ( 'NONE', #2370, #18261, #13933 ) ;
#16540=FACE_OUTER_BOUND ( 'NONE', #8264, .T. ) ;
#16542=LINE ( 'NONE', #817, #3292 ) ;
#16543=EDGE_CURVE ( 'NONE', #11671, #794, #10167, .T. ) ;
#16544=DIRECTION ( 'NONE',  ( -0.1566598588826321192, 0.9876526153536342445, 7.798540720466731404E-17 ) ) ;
#16545=ORIENTED_EDGE ( 'NONE', *, *, #11619, .T. ) ;
#16547=CARTESIAN_POINT ( 'NONE',  ( -18.18859529943003750, -18.07232254922858417, 4.330127018922218518 ) ) ;
#16549=AXIS2_PLACEMENT_3D ( 'NONE', #12557, #2246, #12377 ) ;
#16550=ORIENTED_EDGE ( 'NONE', *, *, #9408, .T. ) ;
#16551=ORIENTED_EDGE ( 'NONE', *, *, #3098, .F. ) ;
#16552=DIRECTION ( 'NONE',  ( -0.1566598588826321747, 0.9876526153536343555, 0.000000000000000000 ) ) ;
#16554=ORIENTED_EDGE ( 'NONE', *, *, #7642, .F. ) ;
#16555=VERTEX_POINT ( 'NONE', #12834 ) ;
#16556=ORIENTED_EDGE ( 'NONE', *, *, #16453, .F. ) ;
#16559=CIRCLE ( 'NONE', #17171, 1.500000000000000888 ) ;
#16560=EDGE_CURVE ( 'NONE', #9583, #13845, #10818, .T. ) ;
#16561=LINE ( 'NONE', #2151, #10863 ) ;
#16562=DIRECTION ( 'NONE',  ( -0.1566598588826321192, 0.9876526153536342445, 7.798540720466730171E-17 ) ) ;
#16563=CARTESIAN_POINT ( 'NONE',  ( -59.83472345504510770, -87.44614099429799126, -4.330127018922185655 ) ) ;
#16564=CARTESIAN_POINT ( 'NONE',  ( -27.28182215855319015, -24.57718421482303484, -21.65063509461098334 ) ) ;
#16565=VECTOR ( 'NONE', #12536, 1000.000000000000000 ) ;
#16566=CARTESIAN_POINT ( 'NONE',  ( -28.26947477390680774, -24.73384407370567217, 1.869203119972154228E-14 ) ) ;
#16567=CIRCLE ( 'NONE', #8391, 1.499999999999999556 ) ;
#16568=CARTESIAN_POINT ( 'NONE',  ( -8.516422466834198346, -21.60064689605303911, -17.32050807568878170 ) ) ;
#16569=DIRECTION ( 'NONE',  ( -0.1566598588826321192, 0.9876526153536342445, 7.798540720466731404E-17 ) ) ;
#16570=VECTOR ( 'NONE', #17885, 1000.000000000000000 ) ;
#16571=DIRECTION ( 'NONE',  ( 0.000000000000000000, 0.000000000000000000, 1.000000000000000000 ) ) ;
#16572=VERTEX_POINT ( 'NONE', #10086 ) ;
#16573=CARTESIAN_POINT ( 'NONE',  ( -36.46016868347218320, -20.97052993855727010, -4.330127018922180326 ) ) ;
#16574=ADVANCED_FACE ( 'NONE', ( #15873 ), #2875, .F. ) ;
#16575=EDGE_LOOP ( 'NONE', ( #11425, #15120 ) ) ;
#16578=ADVANCED_FACE ( 'NONE', ( #18676 ), #9993, .F. ) ;
#16580=VERTEX_POINT ( 'NONE', #7632 ) ;
#16581=VECTOR ( 'NONE', #9315, 1000.000000000000000 ) ;
#16582=EDGE_LOOP ( 'NONE', ( #389, #10935 ) ) ;
#16583=ORIENTED_EDGE ( 'NONE', *, *, #14923, .F. ) ;
#16584=DIRECTION ( 'NONE',  ( -0.1566598588826321192, 0.9876526153536342445, 7.798540720466730171E-17 ) ) ;
#16585=DIRECTION ( 'NONE',  ( -0.1566598588826321192, 0.9876526153536342445, 7.798540720466731404E-17 ) ) ;
#16586=VERTEX_POINT ( 'NONE', #3239 ) ;
#16587=LINE ( 'NONE', #1984, #17298 ) ;
#16591=ORIENTED_EDGE ( 'NONE', *, *, #4673, .F. ) ;
#16593=EDGE_LOOP ( 'NONE', ( #18783, #3110 ) ) ;
#16594=CIRCLE ( 'NONE', #18760, 1.500000000000000888 ) ;
#16595=SURFACE_STYLE_FILL_AREA ( #13538 ) ;
#16598=EDGE_CURVE ( 'NONE', #16165, #18092, #13248, .T. ) ;
#16600=AXIS2_PLACEMENT_3D ( 'NONE', #16480, #7751, #18224 ) ;
#16601=VECTOR ( 'NONE', #17412, 1000.000000000000000 ) ;
#16603=ORIENTED_EDGE ( 'NONE', *, *, #1505, .T. ) ;
#16604=ORIENTED_EDGE ( 'NONE', *, *, #5088, .F. ) ;
#16607=CIRCLE ( 'NONE', #6935, 1.500000000000000888 ) ;
#16608=FACE_BOUND ( 'NONE', #14797, .T. ) ;
#16609=ADVANCED_FACE ( 'NONE', ( #16521 ), #13389, .F. ) ;
#16612=DIRECTION ( 'NONE',  ( -0.1566598588826321192, 0.9876526153536342445, 7.798540720466730171E-17 ) ) ;
#16613=EDGE_LOOP ( 'NONE', ( #2367, #18474, #15580, #3143 ) ) ;
#16615=DIRECTION ( 'NONE',  ( -0.1566598588826321192, 0.9876526153536342445, 7.798540720466730171E-17 ) ) ;
#16616=FACE_BOUND ( 'NONE', #10908, .T. ) ;
#16617=VECTOR ( 'NONE', #6244, 1000.000000000000000 ) ;
#16618=DIRECTION ( 'NONE',  ( 0.000000000000000000, 0.000000000000000000, 1.000000000000000000 ) ) ;
#16619=AXIS2_PLACEMENT_3D ( 'NONE', #11214, #2599, #12538 ) ;
#16620=ORIENTED_EDGE ( 'NONE', *, *, #17484, .F. ) ;
#16622=CARTESIAN_POINT ( 'NONE',  ( -33.20773785067495254, -25.51714336811882688, -8.660254037844380193 ) ) ;
#16623=CARTESIAN_POINT ( 'NONE',  ( -51.27495791377663181, -23.32042782179674845, 4.330127018922218518 ) ) ;
#16625=ORIENTED_EDGE ( 'NONE', *, *, #15550, .F. ) ;
#16626=FACE_OUTER_BOUND ( 'NONE', #16290, .T. ) ;
#16627=CARTESIAN_POINT ( 'NONE',  ( 2.000000000000000000, 2.449293598294706414E-16, 30.00000000000000000 ) ) ;
#16628=AXIS2_PLACEMENT_3D ( 'NONE', #210, #7512, #309 ) ;
#16629=ORIENTED_EDGE ( 'NONE', *, *, #2761, .F. ) ;
#16631=AXIS2_PLACEMENT_3D ( 'NONE', #12795, #18722, #10041 ) ;
#16632=EDGE_LOOP ( 'NONE', ( #17887, #14283 ) ) ;
#16633=CARTESIAN_POINT ( 'NONE',  ( -30.73860631229088369, -25.12549372091224598, -12.99038105676658006 ) ) ;
#16634=EDGE_CURVE ( 'NONE', #1595, #11742, #6331, .T. ) ;
#16636=CIRCLE ( 'NONE', #11749, 1.500000000000000888 ) ;
#16637=VERTEX_POINT ( 'NONE', #427 ) ;
#16638=EDGE_CURVE ( 'NONE', #15242, #5250, #1659, .T. ) ;
#16639=VECTOR ( 'NONE', #4597, 1000.000000000000000 ) ;
#16640=CIRCLE ( 'NONE', #13879, 1.499999999999999556 ) ;
#16641=CIRCLE ( 'NONE', #6054, 1.500000000000000888 ) ;
#16642=DIRECTION ( 'NONE',  ( -0.9876526153536336894, -0.1566598588826349503, 0.000000000000000000 ) ) ;
#16643=ADVANCED_FACE ( 'NONE', ( #16446 ), #11936, .F. ) ;
#16644=CARTESIAN_POINT ( 'NONE',  ( 0.5768043922889515285, -15.09578523045857601, -8.660254037844383745 ) ) ;
#16645=CARTESIAN_POINT ( 'NONE',  ( -28.22983976372896109, -82.43302551005379541, 21.65063509461101532 ) ) ;
#16647=ORIENTED_EDGE ( 'NONE', *, *, #10640, .F. ) ;
#16648=VECTOR ( 'NONE', #14321, 1000.000000000000000 ) ;
#16650=DIRECTION ( 'NONE',  ( -0.1566598588826321747, 0.9876526153536343555, 0.000000000000000000 ) ) ;
#16651=DIRECTION ( 'NONE',  ( -0.1566598588826321747, 0.9876526153536343555, 0.000000000000000000 ) ) ;
#16654=VECTOR ( 'NONE', #11015, 1000.000000000000000 ) ;
#16655=VERTEX_POINT ( 'NONE', #16345 ) ;
#16657=DIRECTION ( 'NONE',  ( -0.9876526153536336894, -0.1566598588826349503, 0.000000000000000000 ) ) ;
#16658=ORIENTED_EDGE ( 'NONE', *, *, #12216, .F. ) ;
#16659=AXIS2_PLACEMENT_3D ( 'NONE', #1019, #6982, #1201 ) ;
#16660=DIRECTION ( 'NONE',  ( -0.1566598588826321192, 0.9876526153536342445, 7.798540720466730171E-17 ) ) ;
#16663=ORIENTED_EDGE ( 'NONE', *, *, #9152, .T. ) ;
#16664=VECTOR ( 'NONE', #14066, 1000.000000000000000 ) ;
#16665=AXIS2_PLACEMENT_3D ( 'NONE', #1637, #16036, #7675 ) ;
#16666=DIRECTION ( 'NONE',  ( -0.1566598588826321747, 0.9876526153536343555, 0.000000000000000000 ) ) ;
#16667=ORIENTED_EDGE ( 'NONE', *, *, #3482, .T. ) ;
#16668=CARTESIAN_POINT ( 'NONE',  ( -39.09401853261888959, -84.15628395776273862, 1.424741226644455312E-14 ) ) ;
#16669=EDGE_CURVE ( 'NONE', #15242, #11338, #7438, .T. ) ;
#16670=CARTESIAN_POINT ( 'NONE',  ( -0.1213752363283457369, -20.26903809555066616, 8.660254037844412167 ) ) ;
#16671=AXIS2_PLACEMENT_3D ( 'NONE', #16960, #13992, #1044 ) ;
#16672=VERTEX_POINT ( 'NONE', #9142 ) ;
#16673=CARTESIAN_POINT ( 'NONE',  ( -33.00338452973448966, -20.42222043246805541, -12.99038105676658006 ) ) ;
#16675=DIRECTION ( 'NONE',  ( -0.1566598588826321192, 0.9876526153536342445, 7.798540720466731404E-17 ) ) ;
#16676=CARTESIAN_POINT ( 'NONE',  ( -46.50141314777111745, -85.33123289938247069, -21.65063509461098690 ) ) ;
#16678=CIRCLE ( 'NONE', #8501, 1.499999999999999556 ) ;
#16681=CIRCLE ( 'NONE', #12417, 1.499999999999997335 ) ;
#16682=DIRECTION ( 'NONE',  ( -0.1566598588826321192, 0.9876526153536342445, 7.798540720466731404E-17 ) ) ;
#16683=ORIENTED_EDGE ( 'NONE', *, *, #16977, .F. ) ;
#16684=CIRCLE ( 'NONE', #16990, 1.499999999999999556 ) ;
#16686=ORIENTED_EDGE ( 'NONE', *, *, #2341, .T. ) ;
#16689=EDGE_LOOP ( 'NONE', ( #4366, #2024 ) ) ;
#16690=CIRCLE ( 'NONE', #947, 1.499999999999999556 ) ;
#16692=CARTESIAN_POINT ( 'NONE',  ( -4.526176995241833367, -78.67318889687062722, -17.32050807568878525 ) ) ;
#16693=CIRCLE ( 'NONE', #10895, 1.500000000000001332 ) ;
#16695=VERTEX_POINT ( 'NONE', #11759 ) ;
#16696=CYLINDRICAL_SURFACE ( 'NONE', #6394, 1.500000000000000666 ) ;
#16697=CARTESIAN_POINT ( 'NONE',  ( -68.55887868246516348, -26.06197535224279349, -17.32050807568878170 ) ) ;
#16698=DIRECTION ( 'NONE',  ( 0.000000000000000000, 0.000000000000000000, 1.000000000000000000 ) ) ;
#16702=DIRECTION ( 'NONE',  ( -0.1566598588826321192, 0.9876526153536342445, 7.798540720466731404E-17 ) ) ;
#16704=ORIENTED_EDGE ( 'NONE', *, *, #8786, .F. ) ;
#16705=ADVANCED_FACE ( 'NONE', ( #10649 ), #13197, .F. ) ;
#16708=AXIS2_PLACEMENT_3D ( 'NONE', #3004, #13499, #1606 ) ;
#16709=DIRECTION ( 'NONE',  ( 2.887450008416415878E-16, 0.000000000000000000, 1.000000000000000000 ) ) ;
#16712=ORIENTED_EDGE ( 'NONE', *, *, #15232, .T. ) ;
#16714=AXIS2_PLACEMENT_3D ( 'NONE', #2259, #15161, #6268 ) ;
#16715=FACE_BOUND ( 'NONE', #7427, .T. ) ;
#16716=AXIS2_PLACEMENT_3D ( 'NONE', #4364, #3029, #8821 ) ;
#16722=CYLINDRICAL_SURFACE ( 'NONE', #9128, 1.500000000000001554 ) ;
#16723=ORIENTED_EDGE ( 'NONE', *, *, #17292, .T. ) ;
#16724=EDGE_CURVE ( 'NONE', #1063, #16044, #16243, .T. ) ;
#16725=CIRCLE ( 'NONE', #2795, 1.500000000000000888 ) ;
#16726=DIRECTION ( 'NONE',  ( -0.1566598588826321192, 0.9876526153536342445, 7.798540720466730171E-17 ) ) ;
#16727=CARTESIAN_POINT ( 'NONE',  ( -7.528769851480577202, -21.44398703717040888, 4.330127018922214077 ) ) ;
#16728=EDGE_CURVE ( 'NONE', #11102, #442, #14721, .T. ) ;
#16729=CARTESIAN_POINT ( 'NONE',  ( 0.5768043922889515285, -15.09578523045857601, 17.32050807568881368 ) ) ;
#16730=VECTOR ( 'NONE', #15334, 1000.000000000000000 ) ;
#16731=EDGE_CURVE ( 'NONE', #7806, #1829, #328, .T. ) ;
#16732=CARTESIAN_POINT ( 'NONE',  ( -29.05277406831996245, -19.79558099693753803, 8.660254037844417496 ) ) ;
#16733=ORIENTED_EDGE ( 'NONE', *, *, #13827, .T. ) ;
#16734=VERTEX_POINT ( 'NONE', #6682 ) ;
#16735=LINE ( 'NONE', #9711, #18766 ) ;
#16738=EDGE_LOOP ( 'NONE', ( #2069, #300 ) ) ;
#16739=VERTEX_POINT ( 'NONE', #18275 ) ;
#16740=DIRECTION ( 'NONE',  ( -0.1566598588826321747, 0.9876526153536343555, 0.000000000000000000 ) ) ;
#16741=CARTESIAN_POINT ( 'NONE',  ( -2.590506774712417748, -20.66068774275724707, -12.99038105676658361 ) ) ;
#16742=VERTEX_POINT ( 'NONE', #17014 ) ;
#16743=CARTESIAN_POINT ( 'NONE',  ( 2.000000000000000000, 2.449293598294706414E-16, 30.00000000000000000 ) ) ;
#16745=CYLINDRICAL_SURFACE ( 'NONE', #4850, 1.500000000000001554 ) ;
#16746=CARTESIAN_POINT ( 'NONE',  ( -44.85521591397802155, -22.30213873905965372, 21.65063509461101887 ) ) ;
#16747=DIRECTION ( 'NONE',  ( -0.1566598588826321747, 0.9876526153536343555, 0.000000000000000000 ) ) ;
#16750=CYLINDRICAL_SURFACE ( 'NONE', #6280, 1.500000000000001554 ) ;
#16751=ADVANCED_FACE ( 'NONE', ( #15373 ), #14042, .F. ) ;
#16752=CYLINDRICAL_SURFACE ( 'NONE', #6951, 1.500000000000001554 ) ;
#16753=DIRECTION ( 'NONE',  ( -0.9876526153536336894, -0.1566598588826350336, 0.000000000000000000 ) ) ;
#16754=CYLINDRICAL_SURFACE ( 'NONE', #12909, 1.500000000000001554 ) ;
#16756=ADVANCED_FACE ( 'NONE', ( #5246 ), #2293, .F. ) ;
#16757=ORIENTED_EDGE ( 'NONE', *, *, #16353, .F. ) ;
#16758=CIRCLE ( 'NONE', #100, 1.500000000000001332 ) ;
#16760=DIRECTION ( 'NONE',  ( -0.1566598588826321192, 0.9876526153536342445, 7.798540720466730171E-17 ) ) ;
#16762=EDGE_LOOP ( 'NONE', ( #13846, #3343, #7074, #3634 ) ) ;
#16763=ORIENTED_EDGE ( 'NONE', *, *, #467, .T. ) ;
#16764=ORIENTED_EDGE ( 'NONE', *, *, #134, .F. ) ;
#16766=CARTESIAN_POINT ( 'NONE',  ( -67.57122606711153878, -25.90531549336017036, 4.330127018922218518 ) ) ;
#16767=ORIENTED_EDGE ( 'NONE', *, *, #7031, .F. ) ;
#16768=ORIENTED_EDGE ( 'NONE', *, *, #10643, .F. ) ;
#16769=DIRECTION ( 'NONE',  ( -0.1566598588826321192, 0.9876526153536342445, 7.798540720466730171E-17 ) ) ;
#16770=DIRECTION ( 'NONE',  ( -0.9876526153536336894, -0.1566598588826349503, 0.000000000000000000 ) ) ;
#16771=DIRECTION ( 'NONE',  ( -0.1566598588826321192, 0.9876526153536342445, 7.798540720466730171E-17 ) ) ;
#16772=CYLINDRICAL_SURFACE ( 'NONE', #14215, 1.500000000000001554 ) ;
#16773=ORIENTED_EDGE ( 'NONE', *, *, #2973, .T. ) ;
#16774=DIRECTION ( 'NONE',  ( -0.9876526153536344665, -0.1566598588826304539, 0.000000000000000000 ) ) ;
#16775=AXIS2_PLACEMENT_3D ( 'NONE', #18711, #5788, #15901 ) ;
#16777=ORIENTED_EDGE ( 'NONE', *, *, #6776, .T. ) ;
#16781=FACE_OUTER_BOUND ( 'NONE', #10121, .T. ) ;
#16782=EDGE_LOOP ( 'NONE', ( #5285, #17579, #18623, #16854 ) ) ;
#16783=FACE_OUTER_BOUND ( 'NONE', #6148, .T. ) ;
#16784=FACE_OUTER_BOUND ( 'NONE', #7709, .T. ) ;
#16785=EDGE_LOOP ( 'NONE', ( #12307, #12847 ) ) ;
#16786=DIRECTION ( 'NONE',  ( -0.1566598588826321747, 0.9876526153536343555, 0.000000000000000000 ) ) ;
#16787=VECTOR ( 'NONE', #2155, 1000.000000000000000 ) ;
#16788=ORIENTED_EDGE ( 'NONE', *, *, #9567, .T. ) ;
#16789=EDGE_CURVE ( 'NONE', #5230, #16279, #8127, .T. ) ;
#16790=VERTEX_POINT ( 'NONE', #1091 ) ;
#16791=DIRECTION ( 'NONE',  ( -0.1566598588826321192, 0.9876526153536342445, 7.798540720466730171E-17 ) ) ;
#16792=EDGE_CURVE ( 'NONE', #8719, #8399, #16735, .T. ) ;
#16793=ORIENTED_EDGE ( 'NONE', *, *, #11038, .T. ) ;
#16794=DIRECTION ( 'NONE',  ( 0.000000000000000000, 0.000000000000000000, 1.000000000000000000 ) ) ;
#16795=DIRECTION ( 'NONE',  ( 0.000000000000000000, 0.000000000000000000, 1.000000000000000000 ) ) ;
#16796=EDGE_CURVE ( 'NONE', #17807, #7902, #9929, .T. ) ;
#16797=CARTESIAN_POINT ( 'NONE',  ( -51.43967622453926936, -86.11453219379562540, -21.65063509461098690 ) ) ;
#16798=ORIENTED_EDGE ( 'NONE', *, *, #357, .T. ) ;
#16800=DIRECTION ( 'NONE',  ( -0.1566598588826321192, 0.9876526153536342445, 7.798540720466730171E-17 ) ) ;
#16801=PLANE ( 'NONE',  #18151 ) ;
#16802=LINE ( 'NONE', #10880, #8361 ) ;
#16803=EDGE_LOOP ( 'NONE', ( #4765, #9753, #7265, #4625, #5877, #10959, #6926 ) ) ;
#16804=DIRECTION ( 'NONE',  ( -0.1566598588826321192, 0.9876526153536342445, 7.798540720466730171E-17 ) ) ;
#16805=CARTESIAN_POINT ( 'NONE',  ( -32.50955822205765600, -20.34389050302674917, 1.926565525561697761E-14 ) ) ;
#16806=EDGE_CURVE ( 'NONE', #2279, #16410, #16823, .T. ) ;
#16808=ORIENTED_EDGE ( 'NONE', *, *, #11997, .T. ) ;
#16812=FACE_BOUND ( 'NONE', #17287, .T. ) ;
#16813=ADVANCED_FACE ( 'NONE', ( #2499 ), #12608, .F. ) ;
#16815=EDGE_LOOP ( 'NONE', ( #3224, #16029, #1187, #15218 ) ) ;
#16816=CARTESIAN_POINT ( 'NONE',  ( -36.46016868347218320, -20.97052993855726655, -12.99038105676658006 ) ) ;
#16817=CARTESIAN_POINT ( 'NONE',  ( -22.63303206852135929, -18.77729191420043620, 17.32050807568881723 ) ) ;
#16820=DIRECTION ( 'NONE',  ( 0.000000000000000000, 0.000000000000000000, 1.000000000000000000 ) ) ;
#16822=EDGE_LOOP ( 'NONE', ( #16022, #3351, #16009, #18545 ) ) ;
#16823=LINE ( 'NONE', #796, #10534 ) ;
#16824=CIRCLE ( 'NONE', #4679, 1.500000000000001332 ) ;
#16825=DIRECTION ( 'NONE',  ( -0.1566598588826321192, 0.9876526153536342445, 7.798540720466730171E-17 ) ) ;
#16826=EDGE_CURVE ( 'NONE', #11894, #1825, #13665, .T. ) ;
#16827=CARTESIAN_POINT ( 'NONE',  ( -11.93357161039406300, -79.84813783849037350, 21.65063509461100821 ) ) ;
#16828=EDGE_LOOP ( 'NONE', ( #456, #17962 ) ) ;
#16830=CARTESIAN_POINT ( 'NONE',  ( -13.45468554360235203, -22.38394619046619383, -8.660254037844380193 ) ) ;
#16832=EDGE_CURVE ( 'NONE', #15217, #14719, #9664, .T. ) ;
#16834=DIRECTION ( 'NONE',  ( -0.000000000000000000, -0.000000000000000000, -1.000000000000000000 ) ) ;
#16835=DIRECTION ( 'NONE',  ( -0.1566598588826321747, 0.9876526153536343555, 0.000000000000000000 ) ) ;
#16836=ORIENTED_EDGE ( 'NONE', *, *, #11658, .F. ) ;
#16838=FACE_BOUND ( 'NONE', #3383, .T. ) ;
#16840=VECTOR ( 'NONE', #3910, 1000.000000000000000 ) ;
#16843=DIRECTION ( 'NONE',  ( -0.9876526153536336894, -0.1566598588826349503, 0.000000000000000000 ) ) ;
#16844=CARTESIAN_POINT ( 'NONE',  ( -33.99103714508810725, -20.57888029135068564, -17.32050807568878170 ) ) ;
#16845=CARTESIAN_POINT ( 'NONE',  ( -7.818242838216901802, -16.42739403096095074, 8.660254037844413944 ) ) ;
#16847=ORIENTED_EDGE ( 'NONE', *, *, #7662, .F. ) ;
#16850=CARTESIAN_POINT ( 'NONE',  ( -41.39843176024034221, -21.75382923297042481, -12.99038105676658006 ) ) ;
#16852=ORIENTED_EDGE ( 'NONE', *, *, #7189, .F. ) ;
#16853=AXIS2_PLACEMENT_3D ( 'NONE', #4257, #10311, #2749 ) ;
#16854=ORIENTED_EDGE ( 'NONE', *, *, #6802, .T. ) ;
#16855=CARTESIAN_POINT ( 'NONE',  ( -56.37793930130741415, -86.89783148820880854, 12.99038105676661203 ) ) ;
#16856=CARTESIAN_POINT ( 'NONE',  ( 0.3724510713484854851, -20.19070816610934926, 21.65063509461101177 ) ) ;
#16857=DIRECTION ( 'NONE',  ( 0.000000000000000000, 0.000000000000000000, 1.000000000000000000 ) ) ;
#16858=ADVANCED_FACE ( 'NONE', ( #16626 ), #16921, .F. ) ;
#16859=ORIENTED_EDGE ( 'NONE', *, *, #16069, .F. ) ;
#16860=CARTESIAN_POINT ( 'NONE',  ( -46.33669483700847280, -22.53712852738359018, 4.330127018922218518 ) ) ;
#16861=EDGE_CURVE ( 'NONE', #5480, #16555, #1496, .T. ) ;
#16862=VECTOR ( 'NONE', #5708, 1000.000000000000000 ) ;
#16864=FACE_OUTER_BOUND ( 'NONE', #12150, .T. ) ;
#16865=SURFACE_STYLE_USAGE ( .BOTH. , #18315 ) ;
#16866=DIRECTION ( 'NONE',  ( -0.9876526153536341335, -0.1566598588826327021, 0.000000000000000000 ) ) ;
#16867=AXIS2_PLACEMENT_3D ( 'NONE', #13341, #16569, #4621 ) ;
#16869=CARTESIAN_POINT ( 'NONE',  ( -26.78799585087635649, -24.49885428538171794, -17.32050807568878170 ) ) ;
#16870=DIRECTION ( 'NONE',  ( -0.1566598588826321192, 0.9876526153536342445, 7.798540720466730171E-17 ) ) ;
#16871=ORIENTED_EDGE ( 'NONE', *, *, #14755, .T. ) ;
#16872=CARTESIAN_POINT ( 'NONE',  ( -21.64537945316773460, -18.62063205531779886, 12.99038105676661736 ) ) ;
#16873=ORIENTED_EDGE ( 'NONE', *, *, #16826, .T. ) ;
#16874=VERTEX_POINT ( 'NONE', #3608 ) ;
#16875=CARTESIAN_POINT ( 'NONE',  ( -1.892327146095121204, -15.48743487766515337, 4.330127018922213189 ) ) ;
#16876=ORIENTED_EDGE ( 'NONE', *, *, #15330, .F. ) ;
#16877=AXIS2_PLACEMENT_3D ( 'NONE', #9862, #7324, #104 ) ;
#16878=CARTESIAN_POINT ( 'NONE',  ( 3.231158466157551423, 19.73726462726227737, 30.00000000000000000 ) ) ;
#16879=FACE_OUTER_BOUND ( 'NONE', #2120, .T. ) ;
#16881=VERTEX_POINT ( 'NONE', #2207 ) ;
#16884=AXIS2_PLACEMENT_3D ( 'NONE', #15967, #11496, #11669 ) ;
#16885=LINE ( 'NONE', #6542, #12175 ) ;
#16886=CIRCLE ( 'NONE', #5369, 1.500000000000001332 ) ;
#16887=CARTESIAN_POINT ( 'NONE',  ( 0.5768043922889515285, -15.09578523045857601, 8.660254037844412167 ) ) ;
#16889=VECTOR ( 'NONE', #9651, 1000.000000000000000 ) ;
#16890=EDGE_CURVE ( 'NONE', #11171, #10712, #4504, .T. ) ;
#16891=DIRECTION ( 'NONE',  ( -0.9876526153536341335, -0.1566598588826327021, 0.000000000000000000 ) ) ;
#16892=CARTESIAN_POINT ( 'NONE',  ( -66.08974714408108753, -25.67032570503622679, 12.99038105676661736 ) ) ;
#16893=DIRECTION ( 'NONE',  ( 0.000000000000000000, 0.000000000000000000, 1.000000000000000000 ) ) ;
#16894=DIRECTION ( 'NONE',  ( -0.1566598588826321192, 0.9876526153536342445, 7.798540720466731404E-17 ) ) ;
#16895=VECTOR ( 'NONE', #9988, 1000.000000000000000 ) ;
#16897=FACE_OUTER_BOUND ( 'NONE', #17024, .T. ) ;
#16899=ORIENTED_EDGE ( 'NONE', *, *, #12042, .F. ) ;
#16900=DIRECTION ( 'NONE',  ( 0.000000000000000000, 0.000000000000000000, 1.000000000000000000 ) ) ;
#16901=EDGE_LOOP ( 'NONE', ( #11698, #16712 ) ) ;
#16903=CARTESIAN_POINT ( 'NONE',  ( 2.841582609732560272, -19.79905851890276836, 8.660254037844412167 ) ) ;
#16904=VECTOR ( 'NONE', #6841, 1000.000000000000000 ) ;
#16905=FACE_BOUND ( 'NONE', #689, .T. ) ;
#16907=AXIS2_PLACEMENT_3D ( 'NONE', #15446, #18437, #6547 ) ;
#16908=ADVANCED_FACE ( 'NONE', ( #7341 ), #1552, .F. ) ;
#16909=DIRECTION ( 'NONE',  ( -0.1566598588826321747, 0.9876526153536343555, 0.000000000000000000 ) ) ;
#16910=FACE_BOUND ( 'NONE', #692, .T. ) ;
#16911=ORIENTED_EDGE ( 'NONE', *, *, #15415, .T. ) ;
#16912=CARTESIAN_POINT ( 'NONE',  ( -16.70711637639958269, -17.83733276090463704, 12.99038105676661381 ) ) ;
#16913=VECTOR ( 'NONE', #15909, 1000.000000000000000 ) ;
#16914=DIRECTION ( 'NONE',  ( -0.1566598588826321192, 0.9876526153536342445, 7.798540720466731404E-17 ) ) ;
#16915=CARTESIAN_POINT ( 'NONE',  ( 6.338001773648100468, -76.94993044916168401, -4.330127018922189208 ) ) ;
#16916=EDGE_CURVE ( 'NONE', #5805, #11320, #18492, .T. ) ;
#16917=CYLINDRICAL_SURFACE ( 'NONE', #3171, 1.500000000000001554 ) ;
#16918=AXIS2_PLACEMENT_3D ( 'NONE', #13815, #10878, #4994 ) ;
#16920=CIRCLE ( 'NONE', #606, 1.500000000000001332 ) ;
#16921=CYLINDRICAL_SURFACE ( 'NONE', #14790, 1.500000000000001554 ) ;
#16922=AXIS2_PLACEMENT_3D ( 'NONE', #6242, #652, #3458 ) ;
#16924=ORIENTED_EDGE ( 'NONE', *, *, #3926, .F. ) ;
#16925=EDGE_LOOP ( 'NONE', ( #14486, #14098, #17019, #13221 ) ) ;
#16927=ORIENTED_EDGE ( 'NONE', *, *, #8063, .T. ) ;
#16928=ORIENTED_EDGE ( 'NONE', *, *, #4087, .F. ) ;
#16930=CARTESIAN_POINT ( 'NONE',  ( -56.41757431148526081, -29.19865005186066753, 1.887572821959364500E-14 ) ) ;
#16931=AXIS2_PLACEMENT_3D ( 'NONE', #1841, #7530, #4940 ) ;
#16932=AXIS2_PLACEMENT_3D ( 'NONE', #11533, #13235, #1 ) ;
#16937=CARTESIAN_POINT ( 'NONE',  ( -3.538524379888211335, -78.51652903798800764, -12.99038105676658539 ) ) ;
#16938=LINE ( 'NONE', #18482, #520 ) ;
#16939=ADVANCED_FACE ( 'NONE', ( #1283 ), #11376, .F. ) ;
#16940=DIRECTION ( 'NONE',  ( -0.9876526153536341335, -0.1566598588826327021, 0.000000000000000000 ) ) ;
#16941=VERTEX_POINT ( 'NONE', #14340 ) ;
#16943=FACE_BOUND ( 'NONE', #15708, .T. ) ;
#16944=CYLINDRICAL_SURFACE ( 'NONE', #5808, 1.500000000000000888 ) ;
#16945=ORIENTED_EDGE ( 'NONE', *, *, #4912, .T. ) ;
#16946=EDGE_CURVE ( 'NONE', #14599, #1993, #4794, .T. ) ;
#16947=AXIS2_PLACEMENT_3D ( 'NONE', #10146, #11468, #4286 ) ;
#16948=VERTEX_POINT ( 'NONE', #12993 ) ;
#16951=VECTOR ( 'NONE', #12648, 1000.000000000000000 ) ;
#16952=FACE_OUTER_BOUND ( 'NONE', #7559, .T. ) ;
#16955=CARTESIAN_POINT ( 'NONE',  ( -5.513829610595458064, -78.82984875575326100, 12.99038105676660848 ) ) ;
#16956=CARTESIAN_POINT ( 'NONE',  ( -3.578159390066044665, -20.81734760163988440, 1.522258424776792809E-14 ) ) ;
#16957=ORIENTED_EDGE ( 'NONE', *, *, #5812, .F. ) ;
#16960=CARTESIAN_POINT ( 'NONE',  ( -6.047290928450125946, -21.20899724884646531, -12.99038105676658006 ) ) ;
#16961=LINE ( 'NONE', #15223, #15854 ) ;
#16962=DIRECTION ( 'NONE',  ( -0.1566598588826321192, 0.9876526153536342445, 7.798540720466730171E-17 ) ) ;
#16964=CIRCLE ( 'NONE', #11765, 1.499999999999999556 ) ;
#16965=EDGE_CURVE ( 'NONE', #4998, #5711, #15081, .T. ) ;
#16967=DIRECTION ( 'NONE',  ( -0.1566598588826321192, 0.9876526153536342445, 7.798540720466730171E-17 ) ) ;
#16968=AXIS2_PLACEMENT_3D ( 'NONE', #15702, #11516, #17350 ) ;
#16969=ORIENTED_EDGE ( 'NONE', *, *, #4862, .T. ) ;
#16972=DIRECTION ( 'NONE',  ( -0.1566598588826321192, 0.9876526153536342445, 7.798540720466730171E-17 ) ) ;
#16976=ADVANCED_FACE ( 'NONE', ( #2944 ), #18654, .F. ) ;
#16977=EDGE_CURVE ( 'NONE', #11803, #227, #10256, .T. ) ;
#16978=AXIS2_PLACEMENT_3D ( 'NONE', #15448, #9672, #3957 ) ;
#16980=AXIS2_PLACEMENT_3D ( 'NONE', #7713, #17781, #16237 ) ;
#16981=AXIS2_PLACEMENT_3D ( 'NONE', #5106, #16702, #14971 ) ;
#16982=CARTESIAN_POINT ( 'NONE',  ( -25.80034323552273534, -24.34219442649909126, 21.65063509461101887 ) ) ;
#16984=CARTESIAN_POINT ( 'NONE',  ( -1.892327146095121204, -15.48743487766515337, 21.65063509461101532 ) ) ;
#16986=AXIS2_PLACEMENT_3D ( 'NONE', #9921, #15707, #2734 ) ;
#16987=DIRECTION ( 'NONE',  ( -0.1566598588826321192, 0.9876526153536342445, 7.798540720466731404E-17 ) ) ;
#16989=DIRECTION ( 'NONE',  ( -0.1566598588826321192, 0.9876526153536342445, 7.798540720466731404E-17 ) ) ;
#16990=AXIS2_PLACEMENT_3D ( 'NONE', #17102, #7144, #13090 ) ;
#16991=DIRECTION ( 'NONE',  ( -0.9876526153536336894, -0.1566598588826349503, 0.000000000000000000 ) ) ;
#16992=AXIS2_PLACEMENT_3D ( 'NONE', #675, #18036, #10769 ) ;
#16994=DIRECTION ( 'NONE',  ( -0.1566598588826321747, 0.9876526153536343555, 0.000000000000000000 ) ) ;
#16995=ADVANCED_FACE ( 'NONE', ( #12893 ), #9873, .F. ) ;
#16997=VERTEX_POINT ( 'NONE', #5721 ) ;
#16998=VECTOR ( 'NONE', #1664, 1000.000000000000000 ) ;
#16999=VERTEX_POINT ( 'NONE', #5532 ) ;
#17000=CARTESIAN_POINT ( 'NONE',  ( -26.58364252993588650, -19.40393134973096068, 12.99038105676661736 ) ) ;
#17001=EDGE_CURVE ( 'NONE', #3359, #8246, #11286, .T. ) ;
#17002=VECTOR ( 'NONE', #17430, 1000.000000000000000 ) ;
#17003=FACE_BOUND ( 'NONE', #13096, .T. ) ;
#17004=AXIS2_PLACEMENT_3D ( 'NONE', #9535, #8499, #14284 ) ;
#17005=DIRECTION ( 'NONE',  ( -0.1566598588826321192, 0.9876526153536342445, 7.798540720466731404E-17 ) ) ;
#17006=DIRECTION ( 'NONE',  ( -0.9876526153536341335, -0.1566598588826327021, 0.000000000000000000 ) ) ;
#17007=ORIENTED_EDGE ( 'NONE', *, *, #14405, .F. ) ;
#17010=DIRECTION ( 'NONE',  ( -0.1566598588826321192, 0.9876526153536342445, 7.798540720466730171E-17 ) ) ;
#17011=FACE_OUTER_BOUND ( 'NONE', #6036, .T. ) ;
#17012=CARTESIAN_POINT ( 'NONE',  ( -63.82496892663746735, -30.37359899348040315, -12.99038105676658006 ) ) ;
#17013=DIRECTION ( 'NONE',  ( -0.1566598588826321747, 0.9876526153536343555, 0.000000000000000000 ) ) ;
#17014=CARTESIAN_POINT ( 'NONE',  ( -44.85521591397803576, -22.30213873905964306, -4.330127018922180326 ) ) ;
#17018=ORIENTED_EDGE ( 'NONE', *, *, #14640, .F. ) ;
#17019=ORIENTED_EDGE ( 'NONE', *, *, #1372, .T. ) ;
#17020=CYLINDRICAL_SURFACE ( 'NONE', #1567, 1.500000000000001554 ) ;
#17021=EDGE_CURVE ( 'NONE', #6176, #10934, #16314, .T. ) ;
#17023=ORIENTED_EDGE ( 'NONE', *, *, #10838, .F. ) ;
#17024=EDGE_LOOP ( 'NONE', ( #16235, #6495, #7593, #11899 ) ) ;
#17025=DIRECTION ( 'NONE',  ( -0.9876526153536344665, -0.1566598588826304539, 0.000000000000000000 ) ) ;
#17026=CIRCLE ( 'NONE', #6105, 1.500000000000000888 ) ;
#17027=CIRCLE ( 'NONE', #1886, 1.500000000000001332 ) ;
#17028=CARTESIAN_POINT ( 'NONE',  ( -22.63303206852135929, -18.77729191420042909, -8.660254037844380193 ) ) ;
#17029=ORIENTED_EDGE ( 'NONE', *, *, #7503, .F. ) ;
#17030=EDGE_CURVE ( 'NONE', #10706, #8349, #8446, .T. ) ;
#17031=VECTOR ( 'NONE', #7214, 1000.000000000000000 ) ;
#17033=FACE_OUTER_BOUND ( 'NONE', #10104, .T. ) ;
#17034=CARTESIAN_POINT ( 'NONE',  ( -15.92381708198643153, -22.77559583767277473, -4.330127018922181215 ) ) ;
#17036=DIRECTION ( 'NONE',  ( -0.9876526153536336894, -0.1566598588826349503, 0.000000000000000000 ) ) ;
#17037=DIRECTION ( 'NONE',  ( -0.1566598588826321747, 0.9876526153536343555, 0.000000000000000000 ) ) ;
#17038=AXIS2_PLACEMENT_3D ( 'NONE', #3582, #3683, #874 ) ;
#17039=CARTESIAN_POINT ( 'NONE',  ( 2.058283315319403783, -14.86079544213463066, 8.660254037844412167 ) ) ;
#17040=ORIENTED_EDGE ( 'NONE', *, *, #5567, .F. ) ;
#17041=EDGE_LOOP ( 'NONE', ( #14631, #2242 ) ) ;
#17043=CARTESIAN_POINT ( 'NONE',  ( -30.73860631229088369, -25.12549372091224598, -21.65063509461098334 ) ) ;
#17044=CARTESIAN_POINT ( 'NONE',  ( -10.45209268736360997, -79.61314805016641571, 4.330127018922213189 ) ) ;
#17045=ORIENTED_EDGE ( 'NONE', *, *, #18409, .F. ) ;
#17046=AXIS2_PLACEMENT_3D ( 'NONE', #261, #5687, #15999 ) ;
#17048=EDGE_LOOP ( 'NONE', ( #14326, #7049, #15754, #10602 ) ) ;
#17050=EDGE_CURVE ( 'NONE', #13155, #3602, #11731, .T. ) ;
#17052=DIRECTION ( 'NONE',  ( -0.9876526153536336894, -0.1566598588826349503, 0.000000000000000000 ) ) ;
#17053=EDGE_CURVE ( 'NONE', #8527, #7443, #6016, .T. ) ;
#17055=CARTESIAN_POINT ( 'NONE',  ( -72.50948914387967648, -26.68861478777331797, -21.65063509461098334 ) ) ;
#17059=EDGE_LOOP ( 'NONE', ( #17623, #5494, #4653, #277 ) ) ;
#17061=DIRECTION ( 'NONE',  ( -0.1566598588826321192, 0.9876526153536342445, 7.798540720466730171E-17 ) ) ;
#17063=VERTEX_POINT ( 'NONE', #14619 ) ;
#17065=CARTESIAN_POINT ( 'NONE',  ( -63.62061560569701157, -25.27867605782964233, 1.908195823574487804E-14 ) ) ;
#17068=ORIENTED_EDGE ( 'NONE', *, *, #16457, .T. ) ;
#17069=ORIENTED_EDGE ( 'NONE', *, *, #5449, .F. ) ;
#17070=ADVANCED_FACE ( 'NONE', ( #400 ), #4462, .F. ) ;
#17071=EDGE_CURVE ( 'NONE', #370, #12897, #588, .T. ) ;
#17072=CIRCLE ( 'NONE', #8875, 1.500000000000000888 ) ;
#17073=ORIENTED_EDGE ( 'NONE', *, *, #7737, .T. ) ;
#17074=LINE ( 'NONE', #14202, #8829 ) ;
#17075=ORIENTED_EDGE ( 'NONE', *, *, #8638, .T. ) ;
#17076=DIRECTION ( 'NONE',  ( -0.1566598588826321192, 0.9876526153536342445, 7.798540720466730171E-17 ) ) ;
#17078=CYLINDRICAL_SURFACE ( 'NONE', #15795, 1.500000000000001554 ) ;
#17079=LINE ( 'NONE', #1066, #11112 ) ;
#17080=FACE_OUTER_BOUND ( 'NONE', #4674, .T. ) ;
#17082=DIRECTION ( 'NONE',  ( -0.9876526153536336894, -0.1566598588826349503, 0.000000000000000000 ) ) ;
#17084=ORIENTED_EDGE ( 'NONE', *, *, #15772, .F. ) ;
#17085=ORIENTED_EDGE ( 'NONE', *, *, #10702, .F. ) ;
#17086=FACE_OUTER_BOUND ( 'NONE', #15654, .T. ) ;
#17087=ORIENTED_EDGE ( 'NONE', *, *, #3453, .T. ) ;
#17090=ORIENTED_EDGE ( 'NONE', *, *, #219, .F. ) ;
#17091=CARTESIAN_POINT ( 'NONE',  ( -2.057045456857760524, -78.28153924966404986, -21.65063509461098690 ) ) ;
#17092=ORIENTED_EDGE ( 'NONE', *, *, #13337, .T. ) ;
#17093=DIRECTION ( 'NONE',  ( 0.000000000000000000, 0.000000000000000000, 1.000000000000000000 ) ) ;
#17095=EDGE_CURVE ( 'NONE', #18001, #7282, #2984, .T. ) ;
#17096=EDGE_CURVE ( 'NONE', #959, #6534, #5986, .T. ) ;
#17097=DIRECTION ( 'NONE',  ( -0.1566598588826321192, 0.9876526153536342445, 7.798540720466730171E-17 ) ) ;
#17098=ORIENTED_EDGE ( 'NONE', *, *, #12697, .T. ) ;
#17099=EDGE_LOOP ( 'NONE', ( #7755, #16265 ) ) ;
#17100=ORIENTED_EDGE ( 'NONE', *, *, #7149, .T. ) ;
#17101=EDGE_CURVE ( 'NONE', #4996, #15703, #16219, .T. ) ;
#17102=CARTESIAN_POINT ( 'NONE',  ( -48.80582637539254875, -22.92877817459017109, 8.660254037844417496 ) ) ;
#17103=CYLINDRICAL_SURFACE ( 'NONE', #14545, 1.500000000000001554 ) ;
#17104=CARTESIAN_POINT ( 'NONE',  ( -52.42732883989288695, -86.27119205267825919, 1.443110928631665584E-14 ) ) ;
#17105=CARTESIAN_POINT ( 'NONE',  ( -3.538524379888211335, -78.51652903798800764, -4.330127018922185655 ) ) ;
#17106=ORIENTED_EDGE ( 'NONE', *, *, #4726, .T. ) ;
#17107=ORIENTED_EDGE ( 'NONE', *, *, #572, .T. ) ;
#17108=ORIENTED_EDGE ( 'NONE', *, *, #8231, .T. ) ;
#17109=ORIENTED_EDGE ( 'NONE', *, *, #10416, .F. ) ;
#17111=EDGE_LOOP ( 'NONE', ( #5830, #14868 ) ) ;
#17112=AXIS2_PLACEMENT_3D ( 'NONE', #4230, #17249, #18045 ) ;
#17113=CARTESIAN_POINT ( 'NONE',  ( -6.995308533625909320, -79.06483854407721878, 21.65063509461100821 ) ) ;
#17115=CYLINDRICAL_SURFACE ( 'NONE', #5401, 1.500000000000001554 ) ;
#17117=ORIENTED_EDGE ( 'NONE', *, *, #11422, .T. ) ;
#17118=EDGE_CURVE ( 'NONE', #8008, #2990, #15694, .T. ) ;
#17119=LINE ( 'NONE', #6886, #8763 ) ;
#17120=VECTOR ( 'NONE', #159, 1000.000000000000000 ) ;
#17121=DIRECTION ( 'NONE',  ( -0.9876526153536336894, -0.1566598588826349503, 0.000000000000000000 ) ) ;
#17122=ORIENTED_EDGE ( 'NONE', *, *, #3822, .F. ) ;
#17123=DIRECTION ( 'NONE',  ( -0.1566598588826321192, 0.9876526153536342445, 7.798540720466730171E-17 ) ) ;
#17124=CARTESIAN_POINT ( 'NONE',  ( -2.057045456857756971, -78.28153924966404986, 4.330127018922209636 ) ) ;
#17125=VERTEX_POINT ( 'NONE', #8836 ) ;
#17126=EDGE_LOOP ( 'NONE', ( #12873, #2066, #413, #3447 ) ) ;
#17127=FACE_BOUND ( 'NONE', #7169, .T. ) ;
#17128=DIRECTION ( 'NONE',  ( -0.1566598588826321747, 0.9876526153536343555, 0.000000000000000000 ) ) ;
#17129=EDGE_CURVE ( 'NONE', #17592, #6604, #9112, .T. ) ;
#17130=CARTESIAN_POINT ( 'NONE',  ( -15.88418207180859021, -80.47477727402089442, 8.660254037844412167 ) ) ;
#17132=CARTESIAN_POINT ( 'NONE',  ( -9.464440072009985272, -79.45648819128378193, -17.32050807568878525 ) ) ;
#17133=ORIENTED_EDGE ( 'NONE', *, *, #4493, .F. ) ;
#17135=DIRECTION ( 'NONE',  ( -0.1566598588826321192, 0.9876526153536342445, 7.798540720466730171E-17 ) ) ;
#17136=VERTEX_POINT ( 'NONE', #590 ) ;
#17137=LINE ( 'NONE', #18773, #15157 ) ;
#17138=DIRECTION ( 'NONE',  ( -0.9876526153536336894, -0.1566598588826349503, 0.000000000000000000 ) ) ;
#17139=CARTESIAN_POINT ( 'NONE',  ( -81.73462711737164454, 33.01666666666666572, -24.99999999999999289 ) ) ;
#17140=ORIENTED_EDGE ( 'NONE', *, *, #8606, .T. ) ;
#17143=EDGE_CURVE ( 'NONE', #17712, #11092, #1775, .T. ) ;
#17145=CARTESIAN_POINT ( 'NONE',  ( -32.22008523532134205, -25.36048350923618955, -12.99038105676658006 ) ) ;
#17146=DIRECTION ( 'NONE',  ( -0.1566598588826321192, 0.9876526153536342445, 7.798540720466731404E-17 ) ) ;
#17148=ORIENTED_EDGE ( 'NONE', *, *, #13198, .T. ) ;
#17151=CARTESIAN_POINT ( 'NONE',  ( -10.98555400521827963, -21.99229654325962002, -12.99038105676658006 ) ) ;
#17152=ORIENTED_EDGE ( 'NONE', *, *, #7688, .F. ) ;
#17153=EDGE_CURVE ( 'NONE', #16032, #15072, #11446, .T. ) ;
#17156=EDGE_LOOP ( 'NONE', ( #14550, #7586, #15734, #13382 ) ) ;
#17157=DIRECTION ( 'NONE',  ( -0.9876526153536344665, -0.1566598588826304539, 0.000000000000000000 ) ) ;
#17158=EDGE_LOOP ( 'NONE', ( #17018, #2166 ) ) ;
#17160=DIRECTION ( 'NONE',  ( -0.1566598588826321192, 0.9876526153536342445, 7.798540720466731404E-17 ) ) ;
#17161=VECTOR ( 'NONE', #1497, 1000.000000000000000 ) ;
#17162=DIRECTION ( 'NONE',  ( -0.1566598588826321192, 0.9876526153536342445, 7.798540720466730171E-17 ) ) ;
#17163=CYLINDRICAL_SURFACE ( 'NONE', #2962, 1.500000000000001554 ) ;
#17164=DIRECTION ( 'NONE',  ( -0.1566598588826321192, 0.9876526153536342445, 7.798540720466730171E-17 ) ) ;
#17165=ORIENTED_EDGE ( 'NONE', *, *, #9393, .F. ) ;
#17167=ADVANCED_FACE ( 'NONE', ( #10425 ), #17577, .F. ) ;
#17168=EDGE_CURVE ( 'NONE', #9341, #14582, #3402, .T. ) ;
#17170=EDGE_CURVE ( 'NONE', #11831, #18705, #6186, .T. ) ;
#17171=AXIS2_PLACEMENT_3D ( 'NONE', #2565, #12799, #11449 ) ;
#17173=CARTESIAN_POINT ( 'NONE',  ( 4.362696542940843081, -77.26325016692693737, 12.99038105676660493 ) ) ;
#17174=ORIENTED_EDGE ( 'NONE', *, *, #3578, .F. ) ;
#17175=EDGE_CURVE ( 'NONE', #3440, #13905, #4517, .T. ) ;
#17176=VERTEX_POINT ( 'NONE', #8919 ) ;
#17177=CARTESIAN_POINT ( 'NONE',  ( -38.10636591726526490, -83.99962409888010484, -4.330127018922185655 ) ) ;
#17178=ORIENTED_EDGE ( 'NONE', *, *, #2080, .T. ) ;
#17179=AXIS2_PLACEMENT_3D ( 'NONE', #17651, #7673, #13613 ) ;
#17180=ORIENTED_EDGE ( 'NONE', *, *, #18125, .T. ) ;
#17181=ORIENTED_EDGE ( 'NONE', *, *, #8245, .T. ) ;
#17182=EDGE_LOOP ( 'NONE', ( #13113, #2860 ) ) ;
#17183=CYLINDRICAL_SURFACE ( 'NONE', #16877, 1.500000000000001554 ) ;
#17185=DIRECTION ( 'NONE',  ( -0.9876526153536341335, -0.1566598588826327021, 0.000000000000000000 ) ) ;
#17186=AXIS2_PLACEMENT_3D ( 'NONE', #10225, #3028, #7406 ) ;
#17187=DIRECTION ( 'NONE',  ( 0.000000000000000000, 0.000000000000000000, 1.000000000000000000 ) ) ;
#17188=CIRCLE ( 'NONE', #7188, 1.500000000000000000 ) ;
#17190=DIRECTION ( 'NONE',  ( -0.1566598588826321192, 0.9876526153536342445, 7.798540720466731404E-17 ) ) ;
#17191=VERTEX_POINT ( 'NONE', #17855 ) ;
#17193=EDGE_LOOP ( 'NONE', ( #11788, #13597 ) ) ;
#17194=EDGE_CURVE ( 'NONE', #4463, #2115, #11917, .T. ) ;
#17195=EDGE_LOOP ( 'NONE', ( #8785, #11117, #3712, #3598 ) ) ;
#17196=CARTESIAN_POINT ( 'NONE',  ( -33.20773785067495254, -25.51714336811882688, -17.32050807568878170 ) ) ;
#17197=CARTESIAN_POINT ( 'NONE',  ( -37.94164760650263446, -21.20551972688122433, 12.99038105676661736 ) ) ;
#17198=CARTESIAN_POINT ( 'NONE',  ( -49.01017969633301163, -28.02370111024092481, 12.99038105676661736 ) ) ;
#17199=DIRECTION ( 'NONE',  ( -0.1566598588826321192, 0.9876526153536342445, 7.798540720466730171E-17 ) ) ;
#17200=DIRECTION ( 'NONE',  ( -0.9876526153536341335, -0.1566598588826327021, 0.000000000000000000 ) ) ;
#17201=ORIENTED_EDGE ( 'NONE', *, *, #12497, .T. ) ;
#17202=EDGE_CURVE ( 'NONE', #10018, #4398, #14515, .T. ) ;
#17203=ORIENTED_EDGE ( 'NONE', *, *, #7428, .T. ) ;
#17204=ORIENTED_EDGE ( 'NONE', *, *, #11491, .T. ) ;
#17206=DIRECTION ( 'NONE',  ( -0.1566598588826321192, 0.9876526153536342445, 7.798540720466730171E-17 ) ) ;
#17207=EDGE_CURVE ( 'NONE', #7553, #15083, #13586, .T. ) ;
#17208=ORIENTED_EDGE ( 'NONE', *, *, #81, .F. ) ;
#17209=FACE_BOUND ( 'NONE', #4747, .T. ) ;
#17210=VECTOR ( 'NONE', #8285, 1000.000000000000000 ) ;
#17211=FACE_OUTER_BOUND ( 'NONE', #7972, .T. ) ;
#17213=CARTESIAN_POINT ( 'NONE',  ( -22.63303206852135929, -18.77729191420043620, 8.660254037844417496 ) ) ;
#17214=CARTESIAN_POINT ( 'NONE',  ( -50.45202360918563045, -85.95787233491300583, 8.660254037844412167 ) ) ;
#17215=DIRECTION ( 'NONE',  ( -0.1566598588826321192, 0.9876526153536342445, 7.798540720466730171E-17 ) ) ;
#17217=AXIS2_PLACEMENT_3D ( 'NONE', #17424, #1316, #1492 ) ;
#17218=DIRECTION ( 'NONE',  ( 0.000000000000000000, 0.000000000000000000, 1.000000000000000000 ) ) ;
#17222=DIRECTION ( 'NONE',  ( -0.9876526153536336894, -0.1566598588826349503, 0.000000000000000000 ) ) ;
#17224=VERTEX_POINT ( 'NONE', #12302 ) ;
#17225=ORIENTED_EDGE ( 'NONE', *, *, #11457, .T. ) ;
#17226=FACE_BOUND ( 'NONE', #17743, .T. ) ;
#17227=DIRECTION ( 'NONE',  ( -0.1566598588826321192, 0.9876526153536342445, 7.798540720466731404E-17 ) ) ;
#17228=ORIENTED_EDGE ( 'NONE', *, *, #3564, .F. ) ;
#17229=EDGE_CURVE ( 'NONE', #17593, #4102, #9289, .T. ) ;
#17230=DIRECTION ( 'NONE',  ( -0.1566598588826321192, 0.9876526153536342445, 7.798540720466730171E-17 ) ) ;
#17231=CARTESIAN_POINT ( 'NONE',  ( -27.28182215855319015, -24.57718421482303484, 21.65063509461101887 ) ) ;
#17232=VECTOR ( 'NONE', #1390, 1000.000000000000000 ) ;
#17233=EDGE_LOOP ( 'NONE', ( #6166, #13118 ) ) ;
#17234=DIRECTION ( 'NONE',  ( -0.9876526153536336894, -0.1566598588826349503, 0.000000000000000000 ) ) ;
#17237=AXIS2_PLACEMENT_3D ( 'NONE', #1926, #16516, #3508 ) ;
#17238=DIRECTION ( 'NONE',  ( -0.9876526153536336894, -0.1566598588826350336, 0.000000000000000000 ) ) ;
#17239=LINE ( 'NONE', #4217, #12718 ) ;
#17240=VECTOR ( 'NONE', #10752, 1000.000000000000000 ) ;
#17241=DIRECTION ( 'NONE',  ( -0.1566598588826321192, 0.9876526153536342445, 7.798540720466731404E-17 ) ) ;
#17242=DIRECTION ( 'NONE',  ( -0.1566598588826321747, 0.9876526153536343555, 0.000000000000000000 ) ) ;
#17243=CARTESIAN_POINT ( 'NONE',  ( -11.93357161039406300, -79.84813783849037350, 12.99038105676661203 ) ) ;
#17245=VERTEX_POINT ( 'NONE', #8265 ) ;
#17246=CARTESIAN_POINT ( 'NONE',  ( -12.92122422574768592, -80.00479769737299307, 17.32050807568881368 ) ) ;
#17247=ORIENTED_EDGE ( 'NONE', *, *, #14245, .T. ) ;
#17248=CARTESIAN_POINT ( 'NONE',  ( -13.41505053342451426, -80.08312762681433128, 12.99038105676661203 ) ) ;
#17249=DIRECTION ( 'NONE',  ( -0.1566598588826321747, 0.9876526153536343555, 0.000000000000000000 ) ) ;
#17250=AXIS2_PLACEMENT_3D ( 'NONE', #9673, #16987, #1069 ) ;
#17251=CARTESIAN_POINT ( 'NONE',  ( -31.68662391746665463, -82.98133501614300656, 12.99038105676661203 ) ) ;
#17253=DIRECTION ( 'NONE',  ( -0.9876526153536336894, -0.1566598588826349503, 0.000000000000000000 ) ) ;
#17254=AXIS2_PLACEMENT_3D ( 'NONE', #7315, #14499, #13067 ) ;
#17255=ORIENTED_EDGE ( 'NONE', *, *, #15024, .F. ) ;
#17256=DIRECTION ( 'NONE',  ( -0.1566598588826321747, 0.9876526153536343555, 0.000000000000000000 ) ) ;
#17257=DIRECTION ( 'NONE',  ( -0.9876526153536336894, -0.1566598588826349503, 0.000000000000000000 ) ) ;
#17259=DIRECTION ( 'NONE',  ( -0.9876526153536341335, -0.1566598588826327021, 0.000000000000000000 ) ) ;
#17260=ORIENTED_EDGE ( 'NONE', *, *, #13694, .T. ) ;
#17261=ORIENTED_EDGE ( 'NONE', *, *, #4578, .F. ) ;
#17262=EDGE_LOOP ( 'NONE', ( #18571, #9394 ) ) ;
#17263=AXIS2_PLACEMENT_3D ( 'NONE', #6171, #9187, #852 ) ;
#17264=ADVANCED_FACE ( 'NONE', ( #12117 ), #14028, .F. ) ;
#17265=CIRCLE ( 'NONE', #11746, 1.500000000000001332 ) ;
#17266=CARTESIAN_POINT ( 'NONE',  ( -36.62488699423479943, -83.76463431055617548, 12.99038105676661203 ) ) ;
#17267=CARTESIAN_POINT ( 'NONE',  ( -42.09661138885763165, -26.92708209806250608, 21.65063509461101887 ) ) ;
#17268=CIRCLE ( 'NONE', #15716, 1.499999999999999556 ) ;
#17270=AXIS2_PLACEMENT_3D ( 'NONE', #8158, #3583, #8051 ) ;
#17271=VECTOR ( 'NONE', #12514, 1000.000000000000000 ) ;
#17272=FACE_OUTER_BOUND ( 'NONE', #14801, .T. ) ;
#17273=CARTESIAN_POINT ( 'NONE',  ( -27.57129514528951120, -19.56059120861359801, 17.32050807568881723 ) ) ;
#17275=CARTESIAN_POINT ( 'NONE',  ( -79.91688375903190433, -27.86356372939305714, -17.32050807568878170 ) ) ;
#17278=CIRCLE ( 'NONE', #17581, 1.500000000000000000 ) ;
#17280=ORIENTED_EDGE ( 'NONE', *, *, #3058, .F. ) ;
#17281=VECTOR ( 'NONE', #12318, 1000.000000000000000 ) ;
#17282=VERTEX_POINT ( 'NONE', #15069 ) ;
#17283=AXIS2_PLACEMENT_3D ( 'NONE', #14161, #18481, #6594 ) ;
#17284=ORIENTED_EDGE ( 'NONE', *, *, #13193, .T. ) ;
#17285=CARTESIAN_POINT ( 'NONE',  ( -61.31620237807555895, -87.68113078262193483, -21.65063509461098690 ) ) ;
#17286=VERTEX_POINT ( 'NONE', #10888 ) ;
#17287=EDGE_LOOP ( 'NONE', ( #2173, #14573 ) ) ;
#17288=FACE_OUTER_BOUND ( 'NONE', #17933, .T. ) ;
#17289=FACE_BOUND ( 'NONE', #5389, .T. ) ;
#17290=CIRCLE ( 'NONE', #18, 1.500000000000000444 ) ;
#17291=EDGE_CURVE ( 'NONE', #9121, #10521, #17959, .T. ) ;
#17292=EDGE_CURVE ( 'NONE', #12642, #2898, #2092, .T. ) ;
#17293=AXIS2_PLACEMENT_3D ( 'NONE', #16872, #18615, #14093 ) ;
#17294=ORIENTED_EDGE ( 'NONE', *, *, #12961, .F. ) ;
#17296=ADVANCED_FACE ( 'NONE', ( #15171, #5006 ), #16501, .F. ) ;
#17297=VECTOR ( 'NONE', #13286, 1000.000000000000000 ) ;
#17298=VECTOR ( 'NONE', #18131, 1000.000000000000000 ) ;
#17300=DIRECTION ( 'NONE',  ( -0.1566598588826321747, 0.9876526153536343555, 0.000000000000000000 ) ) ;
#17302=AXIS2_PLACEMENT_3D ( 'NONE', #16076, #4595, #11675 ) ;
#17304=VECTOR ( 'NONE', #12938, 1000.000000000000000 ) ;
#17305=ORIENTED_EDGE ( 'NONE', *, *, #10238, .T. ) ;
#17306=ORIENTED_EDGE ( 'NONE', *, *, #5862, .F. ) ;
#17308=EDGE_LOOP ( 'NONE', ( #17582, #15305 ) ) ;
#17309=CARTESIAN_POINT ( 'NONE',  ( -78.43540483600145308, -27.62857394106912068, 8.660254037844417496 ) ) ;
#17311=CIRCLE ( 'NONE', #9102, 1.499999999999999556 ) ;
#17312=FACE_BOUND ( 'NONE', #15505, .T. ) ;
#17313=CIRCLE ( 'NONE', #17004, 1.500000000000001332 ) ;
#17314=DIRECTION ( 'NONE',  ( -0.1566598588826321747, 0.9876526153536343555, 0.000000000000000000 ) ) ;
#17315=ADVANCED_FACE ( 'NONE', ( #3587 ), #9576, .F. ) ;
#17316=ORIENTED_EDGE ( 'NONE', *, *, #18576, .F. ) ;
#17317=CIRCLE ( 'NONE', #12115, 1.500000000000000888 ) ;
#17318=DIRECTION ( 'NONE',  ( -0.1566598588826321747, 0.9876526153536343555, 0.000000000000000000 ) ) ;
#17319=CARTESIAN_POINT ( 'NONE',  ( -71.02801022084922522, -26.45362499944937085, -21.65063509461097979 ) ) ;
#17320=ADVANCED_FACE ( 'NONE', ( #2272 ), #8054, .F. ) ;
#17322=CARTESIAN_POINT ( 'NONE',  ( -43.08426400421126345, -27.08374195694514341, -17.32050807568878170 ) ) ;
#17323=LINE ( 'NONE', #1384, #16895 ) ;
#17324=AXIS2_PLACEMENT_3D ( 'NONE', #6785, #6873, #11201 ) ;
#17326=ORIENTED_EDGE ( 'NONE', *, *, #5478, .T. ) ;
#17327=ORIENTED_EDGE ( 'NONE', *, *, #7361, .F. ) ;
#17329=CIRCLE ( 'NONE', #17626, 1.500000000000000888 ) ;
#17331=CIRCLE ( 'NONE', #979, 1.500000000000000888 ) ;
#17332=CARTESIAN_POINT ( 'NONE',  ( -28.06512145296634486, -19.63892113805489714, -12.99038105676658006 ) ) ;
#17334=CYLINDRICAL_SURFACE ( 'NONE', #1259, 1.500000000000001554 ) ;
#17335=VECTOR ( 'NONE', #969, 1000.000000000000000 ) ;
#17336=CARTESIAN_POINT ( 'NONE',  ( -74.48479437458692587, -27.00193450553859620, 4.330127018922218518 ) ) ;
#17337=CARTESIAN_POINT ( 'NONE',  ( -48.02252708097942246, -27.86704125135829813, -17.32050807568878170 ) ) ;
#17339=FACE_OUTER_BOUND ( 'NONE', #8544, .T. ) ;
#17341=EDGE_CURVE ( 'NONE', #17772, #9210, #17265, .T. ) ;
#17342=CARTESIAN_POINT ( 'NONE',  ( -39.62747985047356281, -26.53543245085591806, 8.660254037844417496 ) ) ;
#17343=VERTEX_POINT ( 'NONE', #3491 ) ;
#17344=DIRECTION ( 'NONE',  ( 0.000000000000000000, 0.000000000000000000, 1.000000000000000000 ) ) ;
#17345=DIRECTION ( 'NONE',  ( -0.9876526153536341335, -0.1566598588826327021, 0.000000000000000000 ) ) ;
#17346=DIRECTION ( 'NONE',  ( -0.1566598588826321192, 0.9876526153536342445, 7.798540720466731404E-17 ) ) ;
#17348=DIRECTION ( 'NONE',  ( -0.1566598588826321747, 0.9876526153536343555, 0.000000000000000000 ) ) ;
#17349=EDGE_CURVE ( 'NONE', #3641, #2692, #5748, .T. ) ;
#17350=DIRECTION ( 'NONE',  ( -0.9876526153536336894, -0.1566598588826349503, 0.000000000000000000 ) ) ;
#17351=ORIENTED_EDGE ( 'NONE', *, *, #11353, .F. ) ;
#17352=CARTESIAN_POINT ( 'NONE',  ( -20.32861884089991023, -81.17974663899272514, -12.99038105676658539 ) ) ;
#17353=VERTEX_POINT ( 'NONE', #10703 ) ;
#17354=AXIS2_PLACEMENT_3D ( 'NONE', #2648, #18634, #11350 ) ;
#17355=ORIENTED_EDGE ( 'NONE', *, *, #13765, .F. ) ;
#17356=LINE ( 'NONE', #7028, #2773 ) ;
#17357=DIRECTION ( 'NONE',  ( -0.9876526153536341335, -0.1566598588826327021, 0.000000000000000000 ) ) ;
#17358=VECTOR ( 'NONE', #14415, 1000.000000000000000 ) ;
#17360=ORIENTED_EDGE ( 'NONE', *, *, #15152, .F. ) ;
#17361=LINE ( 'NONE', #8798, #13356 ) ;
#17362=CARTESIAN_POINT ( 'NONE',  ( -48.97054468615519340, -85.72288254658904805, -8.660254037844385522 ) ) ;
#17363=CARTESIAN_POINT ( 'NONE',  ( -22.79775037928398618, -81.57139628619930249, 1.443110928631665584E-14 ) ) ;
#17364=DIRECTION ( 'NONE',  ( -0.1566598588826321192, 0.9876526153536342445, 7.798540720466730171E-17 ) ) ;
#17365=FACE_BOUND ( 'NONE', #8851, .T. ) ;
#17367=CARTESIAN_POINT ( 'NONE',  ( -67.77557938805200877, -31.00023842901093118, 1.869203119972154228E-14 ) ) ;
#17368=EDGE_LOOP ( 'NONE', ( #5730, #12668 ) ) ;
#17369=EDGE_CURVE ( 'NONE', #12390, #13736, #15114, .T. ) ;
#17371=ORIENTED_EDGE ( 'NONE', *, *, #17369, .T. ) ;
#17373=AXIS2_PLACEMENT_3D ( 'NONE', #16692, #12397, #15158 ) ;
#17375=ORIENTED_EDGE ( 'NONE', *, *, #18277, .F. ) ;
#17376=ADVANCED_FACE ( 'NONE', ( #4923 ), #11, .F. ) ;
#17377=DIRECTION ( 'NONE',  ( -0.1566598588826321192, 0.9876526153536342445, 7.798540720466730171E-17 ) ) ;
#17378=VERTEX_POINT ( 'NONE', #4158 ) ;
#17380=FACE_BOUND ( 'NONE', #10092, .T. ) ;
#17381=CARTESIAN_POINT ( 'NONE',  ( -56.21322099054476240, -24.10372711620991382, 21.65063509461102242 ) ) ;
#17382=DIRECTION ( 'NONE',  ( -0.9876526153536336894, -0.1566598588826349503, 0.000000000000000000 ) ) ;
#17383=ORIENTED_EDGE ( 'NONE', *, *, #16497, .T. ) ;
#17384=FACE_BOUND ( 'NONE', #5347, .T. ) ;
#17385=ORIENTED_EDGE ( 'NONE', *, *, #3694, .T. ) ;
#17386=DIRECTION ( 'NONE',  ( -0.1566598588826321192, 0.9876526153536342445, 7.798540720466731404E-17 ) ) ;
#17387=EDGE_CURVE ( 'NONE', #11671, #5804, #2395, .T. ) ;
#17388=CARTESIAN_POINT ( 'NONE',  ( -50.49165861936346289, -28.25869089856487903, 12.99038105676661736 ) ) ;
#17389=LINE ( 'NONE', #7238, #9081 ) ;
#17390=FACE_BOUND ( 'NONE', #6627, .T. ) ;
#17392=ADVANCED_FACE ( 'NONE', ( #1351 ), #15737, .F. ) ;
#17393=ORIENTED_EDGE ( 'NONE', *, *, #11070, .F. ) ;
#17394=EDGE_LOOP ( 'NONE', ( #5342, #4000, #18500, #6681 ) ) ;
#17395=ADVANCED_FACE ( 'NONE', ( #7130 ), #2921, .F. ) ;
#17397=ORIENTED_EDGE ( 'NONE', *, *, #14368, .F. ) ;
#17399=ORIENTED_EDGE ( 'NONE', *, *, #12615, .F. ) ;
#17401=DIRECTION ( 'NONE',  ( -0.1566598588826321192, 0.9876526153536342445, 7.798540720466730171E-17 ) ) ;
#17403=DIRECTION ( 'NONE',  ( -0.1566598588826321192, 0.9876526153536342445, 7.798540720466731404E-17 ) ) ;
#17405=DIRECTION ( 'NONE',  ( -0.9876526153536341335, -0.1566598588826327021, 0.000000000000000000 ) ) ;
#17406=DIRECTION ( 'NONE',  ( -0.1566598588826321192, 0.9876526153536342445, 7.798540720466731404E-17 ) ) ;
#17407=ADVANCED_FACE ( 'NONE', ( #15545 ), #8549, .F. ) ;
#17408=DIRECTION ( 'NONE',  ( -0.1566598588826321192, 0.9876526153536342445, 7.798540720466731404E-17 ) ) ;
#17410=ORIENTED_EDGE ( 'NONE', *, *, #18468, .T. ) ;
#17412=DIRECTION ( 'NONE',  ( -0.1566598588826321192, 0.9876526153536342445, 7.798540720466730171E-17 ) ) ;
#17413=ADVANCED_FACE ( 'NONE', ( #4265 ), #5701, .F. ) ;
#17414=LINE ( 'NONE', #16161, #4757 ) ;
#17416=ORIENTED_EDGE ( 'NONE', *, *, #4137, .T. ) ;
#17417=EDGE_CURVE ( 'NONE', #3263, #14051, #10846, .T. ) ;
#17418=ORIENTED_EDGE ( 'NONE', *, *, #14706, .T. ) ;
#17419=VERTEX_POINT ( 'NONE', #18639 ) ;
#17420=DIRECTION ( 'NONE',  ( -0.1566598588826321192, 0.9876526153536342445, 7.798540720466730171E-17 ) ) ;
#17421=DIRECTION ( 'NONE',  ( -0.9876526153536341335, -0.1566598588826330907, 0.000000000000000000 ) ) ;
#17422=AXIS2_PLACEMENT_3D ( 'NONE', #875, #7967, #11324 ) ;
#17424=CARTESIAN_POINT ( 'NONE',  ( 0.000000000000000000, 0.000000000000000000, 30.00000000000000000 ) ) ;
#17425=CARTESIAN_POINT ( 'NONE',  ( -29.25712738926042888, -24.89050393258829175, -21.65063509461098334 ) ) ;
#17426=CARTESIAN_POINT ( 'NONE',  ( -14.93616446663280328, -22.61893597879013740, -8.660254037844380193 ) ) ;
#17427=CYLINDRICAL_SURFACE ( 'NONE', #9537, 1.500000000000001554 ) ;
#17428=DIRECTION ( 'NONE',  ( 0.000000000000000000, 0.000000000000000000, 1.000000000000000000 ) ) ;
#17430=DIRECTION ( 'NONE',  ( -0.1566598588826321192, 0.9876526153536342445, 7.798540720466730171E-17 ) ) ;
#17431=DIRECTION ( 'NONE',  ( -0.1566598588826321747, 0.9876526153536343555, 0.000000000000000000 ) ) ;
#17432=ORIENTED_EDGE ( 'NONE', *, *, #6987, .F. ) ;
#17433=AXIS2_PLACEMENT_3D ( 'NONE', #2229, #16544, #3534 ) ;
#17434=CYLINDRICAL_SURFACE ( 'NONE', #8787, 1.500000000000001554 ) ;
#17435=EDGE_LOOP ( 'NONE', ( #5267, #5063, #9488, #17832 ) ) ;
#17436=EDGE_CURVE ( 'NONE', #9991, #3282, #8718, .T. ) ;
#17437=EDGE_CURVE ( 'NONE', #795, #11890, #11356, .T. ) ;
#17438=DIRECTION ( 'NONE',  ( -0.9876526153536336894, -0.1566598588826349503, 0.000000000000000000 ) ) ;
#17440=LINE ( 'NONE', #4425, #2528 ) ;
#17441=ORIENTED_EDGE ( 'NONE', *, *, #16728, .T. ) ;
#17442=DIRECTION ( 'NONE',  ( 0.000000000000000000, 0.000000000000000000, 1.000000000000000000 ) ) ;
#17444=DIRECTION ( 'NONE',  ( -0.1566598588826321192, 0.9876526153536342445, 7.798540720466731404E-17 ) ) ;
#17445=AXIS2_PLACEMENT_3D ( 'NONE', #14165, #11114, #11304 ) ;
#17446=LINE ( 'NONE', #4431, #4107 ) ;
#17447=FACE_BOUND ( 'NONE', #2925, .T. ) ;
#17448=DIRECTION ( 'NONE',  ( -0.1566598588826321747, 0.9876526153536343555, 0.000000000000000000 ) ) ;
#17450=ORIENTED_EDGE ( 'NONE', *, *, #16806, .F. ) ;
#17453=VERTEX_POINT ( 'NONE', #14503 ) ;
#17455=ORIENTED_EDGE ( 'NONE', *, *, #4749, .T. ) ;
#17456=VERTEX_POINT ( 'NONE', #1435 ) ;
#17457=DIRECTION ( 'NONE',  ( -0.9876526153536341335, -0.1566598588826327021, 0.000000000000000000 ) ) ;
#17459=FACE_BOUND ( 'NONE', #4497, .T. ) ;
#17460=EDGE_CURVE ( 'NONE', #1264, #14170, #7225, .T. ) ;
#17461=CARTESIAN_POINT ( 'NONE',  ( -36.46016868347218320, -20.97052993855727010, -4.330127018922180326 ) ) ;
#17462=AXIS2_PLACEMENT_3D ( 'NONE', #7420, #7790, #10431 ) ;
#17463=DIRECTION ( 'NONE',  ( -0.1566598588826321192, 0.9876526153536342445, 7.798540720466730171E-17 ) ) ;
#17464=ORIENTED_EDGE ( 'NONE', *, *, #15184, .F. ) ;
#17465=EDGE_CURVE ( 'NONE', #3229, #9249, #6360, .T. ) ;
#17466=FACE_BOUND ( 'NONE', #17193, .T. ) ;
#17467=ORIENTED_EDGE ( 'NONE', *, *, #10214, .T. ) ;
#17468=DIRECTION ( 'NONE',  ( 0.000000000000000000, 0.000000000000000000, 1.000000000000000000 ) ) ;
#17469=CARTESIAN_POINT ( 'NONE',  ( -63.62061560569699736, -25.27867605782964944, 17.32050807568882078 ) ) ;
#17470=CIRCLE ( 'NONE', #8677, 1.499999999999999556 ) ;
#17471=DIRECTION ( 'NONE',  ( -0.1566598588826321192, 0.9876526153536342445, 7.798540720466731404E-17 ) ) ;
#17472=CARTESIAN_POINT ( 'NONE',  ( -52.26261052913024230, -23.47708768067938934, 17.32050807568881723 ) ) ;
#17473=DIRECTION ( 'NONE',  ( -0.1566598588826321747, 0.9876526153536343555, 0.000000000000000000 ) ) ;
#17474=ORIENTED_EDGE ( 'NONE', *, *, #12840, .T. ) ;
#17476=ORIENTED_EDGE ( 'NONE', *, *, #15510, .T. ) ;
#17477=ORIENTED_EDGE ( 'NONE', *, *, #315, .T. ) ;
#17478=FACE_OUTER_BOUND ( 'NONE', #2988, .T. ) ;
#17479=CIRCLE ( 'NONE', #18729, 1.500000000000000888 ) ;
#17480=ORIENTED_EDGE ( 'NONE', *, *, #10634, .F. ) ;
#17481=FACE_BOUND ( 'NONE', #4378, .T. ) ;
#17483=ORIENTED_EDGE ( 'NONE', *, *, #15389, .F. ) ;
#17484=EDGE_CURVE ( 'NONE', #1263, #755, #2703, .T. ) ;
#17485=AXIS2_PLACEMENT_3D ( 'NONE', #4601, #1757, #17997 ) ;
#17486=ORIENTED_EDGE ( 'NONE', *, *, #242, .T. ) ;
#17487=AXIS2_PLACEMENT_3D ( 'NONE', #3565, #16484, #8030 ) ;
#17488=ORIENTED_EDGE ( 'NONE', *, *, #8928, .F. ) ;
#17489=CARTESIAN_POINT ( 'NONE',  ( -40.41077914488671041, -21.59716937408780524, 17.32050807568881723 ) ) ;
#17491=FACE_BOUND ( 'NONE', #6636, .T. ) ;
#17492=AXIS2_PLACEMENT_3D ( 'NONE', #11512, #17346, #17428 ) ;
#17493=DIRECTION ( 'NONE',  ( 0.000000000000000000, 0.000000000000000000, 1.000000000000000000 ) ) ;
#17497=CARTESIAN_POINT ( 'NONE',  ( -9.464440072009985272, -79.45648819128378193, 1.424741226644455312E-14 ) ) ;
#17498=DIRECTION ( 'NONE',  ( -0.1566598588826321192, 0.9876526153536342445, 7.798540720466730171E-17 ) ) ;
#17499=EDGE_LOOP ( 'NONE', ( #3215, #8238, #4903, #5652 ) ) ;
#17500=EDGE_LOOP ( 'NONE', ( #7706, #2253 ) ) ;
#17503=DIRECTION ( 'NONE',  ( -0.9876526153536336894, -0.1566598588826349503, 0.000000000000000000 ) ) ;
#17505=EDGE_CURVE ( 'NONE', #4978, #1802, #6653, .T. ) ;
#17508=CIRCLE ( 'NONE', #9303, 1.500000000000000888 ) ;
#17509=FACE_BOUND ( 'NONE', #1382, .T. ) ;
#17510=ADVANCED_FACE ( 'NONE', ( #17086 ), #4059, .F. ) ;
#17511=EDGE_CURVE ( 'NONE', #4072, #3070, #14803, .T. ) ;
#17514=DIRECTION ( 'NONE',  ( 0.000000000000000000, 0.000000000000000000, 1.000000000000000000 ) ) ;
#17515=DIRECTION ( 'NONE',  ( -0.1566598588826321192, 0.9876526153536342445, 7.798540720466731404E-17 ) ) ;
#17516=AXIS2_PLACEMENT_3D ( 'NONE', #9000, #4731, #13533 ) ;
#17517=EDGE_CURVE ( 'NONE', #18393, #4379, #4443, .T. ) ;
#17518=LINE ( 'NONE', #10285, #8160 ) ;
#17519=ADVANCED_FACE ( 'NONE', ( #10600 ), #16120, .F. ) ;
#17521=VERTEX_POINT ( 'NONE', #13350 ) ;
#17522=FACE_OUTER_BOUND ( 'NONE', #7792, .T. ) ;
#17524=ORIENTED_EDGE ( 'NONE', *, *, #2088, .T. ) ;
#17525=LINE ( 'NONE', #11607, #2748 ) ;
#17526=CIRCLE ( 'NONE', #15984, 1.500000000000000888 ) ;
#17527=VECTOR ( 'NONE', #7807, 1000.000000000000000 ) ;
#17528=DIRECTION ( 'NONE',  ( -0.1566598588826321747, 0.9876526153536343555, 0.000000000000000000 ) ) ;
#17530=AXIS2_PLACEMENT_3D ( 'NONE', #2262, #10613, #10972 ) ;
#17531=CIRCLE ( 'NONE', #14177, 1.500000000000000888 ) ;
#17532=DIRECTION ( 'NONE',  ( -0.1566598588826321192, 0.9876526153536342445, 7.798540720466730171E-17 ) ) ;
#17533=DIRECTION ( 'NONE',  ( -0.9876526153536336894, -0.1566598588826349503, 0.000000000000000000 ) ) ;
#17534=EDGE_LOOP ( 'NONE', ( #15502, #5539 ) ) ;
#17535=MECHANICAL_DESIGN_GEOMETRIC_PRESENTATION_REPRESENTATION('',(#2067),#14179);
#17537=EDGE_CURVE ( 'NONE', #18596, #8348, #214, .T. ) ;
#17538=DIRECTION ( 'NONE',  ( 3.208277787129350839E-17, 0.000000000000000000, -1.000000000000000000 ) ) ;
#17539=CARTESIAN_POINT ( 'NONE',  ( -2.590506774712417748, -20.66068774275724707, 12.99038105676661026 ) ) ;
#17540=AXIS2_PLACEMENT_3D ( 'NONE', #2673, #8466, #7067 ) ;
#17541=CARTESIAN_POINT ( 'NONE',  ( -14.40270314877813895, -80.23978748569695085, 8.660254037844412167 ) ) ;
#17542=DIRECTION ( 'NONE',  ( -0.9876526153536336894, -0.1566598588826350336, 0.000000000000000000 ) ) ;
#17543=FACE_OUTER_BOUND ( 'NONE', #493, .T. ) ;
#17544=ORIENTED_EDGE ( 'NONE', *, *, #1958, .T. ) ;
#17548=AXIS2_PLACEMENT_3D ( 'NONE', #16729, #15560, #8363 ) ;
#17549=CYLINDRICAL_SURFACE ( 'NONE', #16853, 1.500000000000001554 ) ;
#17551=ADVANCED_FACE ( 'NONE', ( #11813 ), #8983, .F. ) ;
#17554=DIRECTION ( 'NONE',  ( -0.1566598588826321747, 0.9876526153536343555, 0.000000000000000000 ) ) ;
#17555=ORIENTED_EDGE ( 'NONE', *, *, #16890, .T. ) ;
#17559=VECTOR ( 'NONE', #14409, 1000.000000000000000 ) ;
#17560=ORIENTED_EDGE ( 'NONE', *, *, #15257, .T. ) ;
#17561=ORIENTED_EDGE ( 'NONE', *, *, #5520, .F. ) ;
#17562=CARTESIAN_POINT ( 'NONE',  ( -24.81269062016911064, -24.18553456761645393, 17.32050807568881723 ) ) ;
#17564=CARTESIAN_POINT ( 'NONE',  ( -12.92122422574768592, -80.00479769737299307, 8.660254037844412167 ) ) ;
#17566=LINE ( 'NONE', #15636, #17358 ) ;
#17567=AXIS2_PLACEMENT_3D ( 'NONE', #8850, #11744, #14710 ) ;
#17568=AXIS2_PLACEMENT_3D ( 'NONE', #15917, #5410, #14222 ) ;
#17569=VERTEX_POINT ( 'NONE', #17741 ) ;
#17570=EDGE_CURVE ( 'NONE', #12897, #11672, #4440, .T. ) ;
#17571=CIRCLE ( 'NONE', #16048, 1.500000000000001332 ) ;
#17572=CARTESIAN_POINT ( 'NONE',  ( -60.16383145195930382, -24.73036655174043474, 8.660254037844417496 ) ) ;
#17573=ORIENTED_EDGE ( 'NONE', *, *, #5589, .T. ) ;
#17575=CIRCLE ( 'NONE', #3600, 1.500000000000001332 ) ;
#17576=DIRECTION ( 'NONE',  ( -0.1566598588826321747, 0.9876526153536343555, 0.000000000000000000 ) ) ;
#17577=CYLINDRICAL_SURFACE ( 'NONE', #16327, 1.500000000000001554 ) ;
#17578=EDGE_CURVE ( 'NONE', #15920, #4102, #14438, .T. ) ;
#17579=ORIENTED_EDGE ( 'NONE', *, *, #3353, .F. ) ;
#17581=AXIS2_PLACEMENT_3D ( 'NONE', #15722, #16276, #14401 ) ;
#17582=ORIENTED_EDGE ( 'NONE', *, *, #10008, .F. ) ;
#17583=DIRECTION ( 'NONE',  ( 0.000000000000000000, 0.000000000000000000, 1.000000000000000000 ) ) ;
#17585=VECTOR ( 'NONE', #12519, 1000.000000000000000 ) ;
#17586=FACE_BOUND ( 'NONE', #4844, .T. ) ;
#17588=CIRCLE ( 'NONE', #2738, 1.500000000000000000 ) ;
#17589=ORIENTED_EDGE ( 'NONE', *, *, #17684, .F. ) ;
#17590=CARTESIAN_POINT ( 'NONE',  ( -12.92122422574768592, -80.00479769737297886, -17.32050807568878525 ) ) ;
#17592=VERTEX_POINT ( 'NONE', #3190 ) ;
#17593=VERTEX_POINT ( 'NONE', #5883 ) ;
#17594=CARTESIAN_POINT ( 'NONE',  ( -37.61253960958843834, -83.92129416943878084, -8.660254037844385522 ) ) ;
#17595=AXIS2_PLACEMENT_3D ( 'NONE', #9812, #2603, #8105 ) ;
#17596=CARTESIAN_POINT ( 'NONE',  ( -43.86756329862440396, -22.14547888017700927, 1.908195823574487804E-14 ) ) ;
#17597=CIRCLE ( 'NONE', #10298, 1.500000000000000444 ) ;
#17598=DIRECTION ( 'NONE',  ( -0.1566598588826321747, 0.9876526153536343555, 0.000000000000000000 ) ) ;
#17599=DIRECTION ( 'NONE',  ( 1.000000000000000000, 0.000000000000000000, 0.000000000000000000 ) ) ;
#17600=LINE ( 'NONE', #15870, #13761 ) ;
#17601=CIRCLE ( 'NONE', #7007, 1.500000000000000888 ) ;
#17602=CARTESIAN_POINT ( 'NONE',  ( -36.66452200441264608, -26.06545287420802737, -8.660254037844380193 ) ) ;
#17604=VERTEX_POINT ( 'NONE', #6169 ) ;
#17605=DIRECTION ( 'NONE',  ( -0.9876526153536341335, -0.1566598588826327021, 0.000000000000000000 ) ) ;
#17606=ORIENTED_EDGE ( 'NONE', *, *, #12486, .F. ) ;
#17607=EDGE_CURVE ( 'NONE', #4488, #11609, #3522, .T. ) ;
#17608=AXIS2_PLACEMENT_3D ( 'NONE', #11999, #6267, #14874 ) ;
#17609=CIRCLE ( 'NONE', #13327, 1.500000000000000000 ) ;
#17610=LINE ( 'NONE', #7269, #13223 ) ;
#17611=CARTESIAN_POINT ( 'NONE',  ( -28.22983976372896109, -82.43302551005379541, -12.99038105676658539 ) ) ;
#17612=AXIS2_PLACEMENT_3D ( 'NONE', #8598, #16166, #11673 ) ;
#17613=ORIENTED_EDGE ( 'NONE', *, *, #14426, .F. ) ;
#17618=AXIS2_PLACEMENT_3D ( 'NONE', #3168, #538, #13319 ) ;
#17619=CARTESIAN_POINT ( 'NONE',  ( -44.56574292724172182, -27.31873174526908699, -17.32050807568878170 ) ) ;
#17620=DIRECTION ( 'NONE',  ( -0.1566598588826321747, 0.9876526153536343555, 0.000000000000000000 ) ) ;
#17622=CIRCLE ( 'NONE', #5508, 1.500000000000000444 ) ;
#17623=ORIENTED_EDGE ( 'NONE', *, *, #8231, .F. ) ;
#17624=CYLINDRICAL_SURFACE ( 'NONE', #6033, 1.500000000000001554 ) ;
#17625=DIRECTION ( 'NONE',  ( 0.000000000000000000, 0.000000000000000000, 1.000000000000000000 ) ) ;
#17626=AXIS2_PLACEMENT_3D ( 'NONE', #8141, #5210, #15053 ) ;
#17627=CIRCLE ( 'NONE', #13353, 1.499999999999999556 ) ;
#17628=DIRECTION ( 'NONE',  ( 0.000000000000000000, 0.000000000000000000, 1.000000000000000000 ) ) ;
#17629=FACE_OUTER_BOUND ( 'NONE', #6287, .T. ) ;
#17630=ORIENTED_EDGE ( 'NONE', *, *, #7378, .T. ) ;
#17631=EDGE_LOOP ( 'NONE', ( #2070, #4309, #3752, #6035 ) ) ;
#17632=CARTESIAN_POINT ( 'NONE',  ( -22.34355908178503469, -23.79388492040988012, 4.330127018922217630 ) ) ;
#17634=ORIENTED_EDGE ( 'NONE', *, *, #353, .T. ) ;
#17635=EDGE_CURVE ( 'NONE', #12573, #2063, #1148, .T. ) ;
#17636=AXIS2_PLACEMENT_3D ( 'NONE', #9197, #14875, #478 ) ;
#17637=EDGE_CURVE ( 'NONE', #9762, #16064, #8988, .T. ) ;
#17639=ORIENTED_EDGE ( 'NONE', *, *, #1970, .T. ) ;
#17641=AXIS2_PLACEMENT_3D ( 'NONE', #12690, #18728, #14511 ) ;
#17642=DIRECTION ( 'NONE',  ( -0.1566598588826321192, 0.9876526153536342445, 7.798540720466730171E-17 ) ) ;
#17643=CARTESIAN_POINT ( 'NONE',  ( -72.71384246482016067, -31.78353772342409300, 17.32050807568881723 ) ) ;
#17644=AXIS2_PLACEMENT_3D ( 'NONE', #4198, #7162, #15778 ) ;
#17645=DIRECTION ( 'NONE',  ( -0.9876526153536341335, -0.1566598588826327021, 0.000000000000000000 ) ) ;
#17646=CARTESIAN_POINT ( 'NONE',  ( -44.03228160938704860, -84.93958325217589334, -8.660254037844385522 ) ) ;
#17647=CARTESIAN_POINT ( 'NONE',  ( -35.47251606811855851, -20.81387007967464697, 17.32050807568881723 ) ) ;
#17649=AXIS2_PLACEMENT_3D ( 'NONE', #1517, #5873, #7305 ) ;
#17651=CARTESIAN_POINT ( 'NONE',  ( 2.881217619910392269, -77.49823995525089515, 4.330127018922209636 ) ) ;
#17654=CARTESIAN_POINT ( 'NONE',  ( -30.73860631229088369, -25.12549372091224598, -21.65063509461098334 ) ) ;
#17655=ORIENTED_EDGE ( 'NONE', *, *, #2037, .F. ) ;
#17657=DIRECTION ( 'NONE',  ( -0.1566598588826321192, 0.9876526153536342445, 7.798540720466730171E-17 ) ) ;
#17658=ORIENTED_EDGE ( 'NONE', *, *, #1166, .F. ) ;
#17660=EDGE_CURVE ( 'NONE', #13224, #8567, #2636, .T. ) ;
#17661=ORIENTED_EDGE ( 'NONE', *, *, #5061, .T. ) ;
#17662=DIRECTION ( 'NONE',  ( -0.1566598588826321192, 0.9876526153536342445, 7.798540720466730171E-17 ) ) ;
#17663=ORIENTED_EDGE ( 'NONE', *, *, #17831, .F. ) ;
#17664=ORIENTED_EDGE ( 'NONE', *, *, #7408, .T. ) ;
#17665=LINE ( 'NONE', #4719, #14127 ) ;
#17667=EDGE_LOOP ( 'NONE', ( #3567, #4244, #18640, #4120 ) ) ;
#17670=FACE_OUTER_BOUND ( 'NONE', #6722, .T. ) ;
#17671=CYLINDRICAL_SURFACE ( 'NONE', #15129, 1.500000000000001554 ) ;
#17672=DIRECTION ( 'NONE',  ( -0.9876526153536336894, -0.1566598588826349503, 0.000000000000000000 ) ) ;
#17673=CARTESIAN_POINT ( 'NONE',  ( 4.362696542940843081, -77.26325016692693737, -12.99038105676658539 ) ) ;
#17674=VERTEX_POINT ( 'NONE', #15235 ) ;
#17675=ORIENTED_EDGE ( 'NONE', *, *, #1576, .T. ) ;
#17676=AXIS2_PLACEMENT_3D ( 'NONE', #10328, #10508, #6265 ) ;
#17677=CARTESIAN_POINT ( 'NONE',  ( -4.526176995241833367, -78.67318889687062722, -8.660254037844385522 ) ) ;
#17678=DIRECTION ( 'NONE',  ( -0.9876526153536341335, -0.1566598588826327021, 0.000000000000000000 ) ) ;
#17679=ORIENTED_EDGE ( 'NONE', *, *, #683, .F. ) ;
#17681=ORIENTED_EDGE ( 'NONE', *, *, #1446, .T. ) ;
#17682=DIRECTION ( 'NONE',  ( 0.000000000000000000, 0.000000000000000000, 1.000000000000000000 ) ) ;
#17683=FACE_BOUND ( 'NONE', #4414, .T. ) ;
#17684=EDGE_CURVE ( 'NONE', #15676, #6194, #6895, .T. ) ;
#17686=EDGE_CURVE ( 'NONE', #13070, #1457, #18734, .T. ) ;
#17687=ORIENTED_EDGE ( 'NONE', *, *, #4241, .T. ) ;
#17688=CIRCLE ( 'NONE', #14927, 1.500000000000000000 ) ;
#17689=CARTESIAN_POINT ( 'NONE',  ( -73.49714175923330117, -26.84527464665595176, -17.32050807568878170 ) ) ;
#17690=ORIENTED_EDGE ( 'NONE', *, *, #1850, .T. ) ;
#17691=ADVANCED_FACE ( 'NONE', ( #2250 ), #10961, .F. ) ;
#17692=ORIENTED_EDGE ( 'NONE', *, *, #1647, .F. ) ;
#17693=ORIENTED_EDGE ( 'NONE', *, *, #3902, .T. ) ;
#17694=CARTESIAN_POINT ( 'NONE',  ( -66.78792677269838407, -30.84357857012830095, 12.99038105676661736 ) ) ;
#17695=DIRECTION ( 'NONE',  ( -0.9876526153536336894, -0.1566598588826350336, 0.000000000000000000 ) ) ;
#17696=DIRECTION ( 'NONE',  ( -0.1566598588826321747, 0.9876526153536343555, 0.000000000000000000 ) ) ;
#17698=CARTESIAN_POINT ( 'NONE',  ( -25.80034323552273534, -24.34219442649909126, 12.99038105676661736 ) ) ;
#17699=VERTEX_POINT ( 'NONE', #18118 ) ;
#17701=AXIS2_PLACEMENT_3D ( 'NONE', #9373, #18238, #11157 ) ;
#17703=DIRECTION ( 'NONE',  ( 0.000000000000000000, 0.000000000000000000, 1.000000000000000000 ) ) ;
#17704=DIRECTION ( 'NONE',  ( -0.9876526153536336894, -0.1566598588826350336, 0.000000000000000000 ) ) ;
#17706=LINE ( 'NONE', #7536, #52 ) ;
#17707=EDGE_CURVE ( 'NONE', #3093, #1326, #13907, .T. ) ;
#17709=EDGE_CURVE ( 'NONE', #1903, #14341, #16567, .T. ) ;
#17712=VERTEX_POINT ( 'NONE', #7757 ) ;
#17713=DIRECTION ( 'NONE',  ( -0.9876526153536341335, -0.1566598588826327021, 0.000000000000000000 ) ) ;
#17714=FACE_OUTER_BOUND ( 'NONE', #9974, .T. ) ;
#17716=CYLINDRICAL_SURFACE ( 'NONE', #16198, 1.500000000000001554 ) ;
#17717=ORIENTED_EDGE ( 'NONE', *, *, #7059, .F. ) ;
#17718=ORIENTED_EDGE ( 'NONE', *, *, #12663, .F. ) ;
#17719=CYLINDRICAL_SURFACE ( 'NONE', #2450, 1.500000000000000666 ) ;
#17720=ORIENTED_EDGE ( 'NONE', *, *, #17746, .F. ) ;
#17721=ORIENTED_EDGE ( 'NONE', *, *, #14075, .T. ) ;
#17722=CIRCLE ( 'NONE', #16185, 1.500000000000000888 ) ;
#17724=EDGE_CURVE ( 'NONE', #14381, #7806, #18107, .T. ) ;
#17725=CARTESIAN_POINT ( 'NONE',  ( -38.92930022185626626, -21.36217958576384390, -17.32050807568878170 ) ) ;
#17726=ORIENTED_EDGE ( 'NONE', *, *, #13156, .F. ) ;
#17728=CARTESIAN_POINT ( 'NONE',  ( -40.61513246582718750, -26.69209230973856251, -21.65063509461098334 ) ) ;
#17729=EDGE_LOOP ( 'NONE', ( #9578, #383 ) ) ;
#17730=DIRECTION ( 'NONE',  ( -0.9876526153536341335, -0.1566598588826327021, 0.000000000000000000 ) ) ;
#17731=EDGE_CURVE ( 'NONE', #6405, #6362, #5367, .T. ) ;
#17732=DIRECTION ( 'NONE',  ( -0.1566598588826321192, 0.9876526153536342445, 7.798540720466730171E-17 ) ) ;
#17733=LINE ( 'NONE', #11982, #486 ) ;
#17734=CIRCLE ( 'NONE', #10137, 1.500000000000000000 ) ;
#17736=DIRECTION ( 'NONE',  ( 0.000000000000000000, 0.000000000000000000, 1.000000000000000000 ) ) ;
#17737=CARTESIAN_POINT ( 'NONE',  ( -11.93357161039406300, -79.84813783849035929, -12.99038105676658539 ) ) ;
#17738=ORIENTED_EDGE ( 'NONE', *, *, #16789, .T. ) ;
#17739=ORIENTED_EDGE ( 'NONE', *, *, #13175, .F. ) ;
#17740=EDGE_LOOP ( 'NONE', ( #16620, #2234, #5713, #710 ) ) ;
#17741=CARTESIAN_POINT ( 'NONE',  ( -10.28737437660098131, -16.81904367816753165, -12.99038105676658006 ) ) ;
#17742=VERTEX_POINT ( 'NONE', #12279 ) ;
#17743=EDGE_LOOP ( 'NONE', ( #12191, #12801 ) ) ;
#17744=DIRECTION ( 'NONE',  ( 0.000000000000000000, 0.000000000000000000, 1.000000000000000000 ) ) ;
#17745=FACE_OUTER_BOUND ( 'NONE', #14788, .T. ) ;
#17746=EDGE_CURVE ( 'NONE', #11470, #17593, #9899, .T. ) ;
#17747=DIRECTION ( 'NONE',  ( -0.9876526153536341335, -0.1566598588826327021, 0.000000000000000000 ) ) ;
#17748=CIRCLE ( 'NONE', #781, 1.500000000000000888 ) ;
#17749=VERTEX_POINT ( 'NONE', #15150 ) ;
#17750=PLANE ( 'NONE',  #8838 ) ;
#17751=ADVANCED_FACE ( 'NONE', ( #6358 ), #9555, .F. ) ;
#17755=DIRECTION ( 'NONE',  ( -0.1566598588826321747, 0.9876526153536343555, 0.000000000000000000 ) ) ;
#17757=ORIENTED_EDGE ( 'NONE', *, *, #12239, .T. ) ;
#17758=FACE_BOUND ( 'NONE', #16582, .T. ) ;
#17759=ADVANCED_FACE ( 'NONE', ( #2342 ), #17939, .F. ) ;
#17761=ORIENTED_EDGE ( 'NONE', *, *, #6987, .T. ) ;
#17762=DIRECTION ( 'NONE',  ( -0.1566598588826321747, 0.9876526153536343555, 0.000000000000000000 ) ) ;
#17763=DIRECTION ( 'NONE',  ( -0.1566598588826321747, 0.9876526153536343555, 0.000000000000000000 ) ) ;
#17765=ORIENTED_EDGE ( 'NONE', *, *, #4609, .F. ) ;
#17767=ORIENTED_EDGE ( 'NONE', *, *, #13285, .F. ) ;
#17768=DIRECTION ( 'NONE',  ( -0.1566598588826321192, 0.9876526153536342445, 7.798540720466730171E-17 ) ) ;
#17769=ORIENTED_EDGE ( 'NONE', *, *, #17709, .F. ) ;
#17770=ORIENTED_EDGE ( 'NONE', *, *, #10438, .F. ) ;
#17771=FACE_BOUND ( 'NONE', #4268, .T. ) ;
#17772=VERTEX_POINT ( 'NONE', #851 ) ;
#17773=DIRECTION ( 'NONE',  ( -0.9876526153536341335, -0.1566598588826327021, 0.000000000000000000 ) ) ;
#17776=EDGE_LOOP ( 'NONE', ( #12209, #13663 ) ) ;
#17777=DIRECTION ( 'NONE',  ( -0.9876526153536344665, -0.1566598588826304539, 0.000000000000000000 ) ) ;
#17778=FACE_BOUND ( 'NONE', #15955, .T. ) ;
#17779=CYLINDRICAL_SURFACE ( 'NONE', #1590, 1.500000000000000888 ) ;
#17781=DIRECTION ( 'NONE',  ( -0.1566598588826321747, 0.9876526153536343555, 0.000000000000000000 ) ) ;
#17785=ORIENTED_EDGE ( 'NONE', *, *, #8676, .T. ) ;
#17787=DIRECTION ( 'NONE',  ( -0.1566598588826321192, 0.9876526153536342445, 7.798540720466730171E-17 ) ) ;
#17789=DIRECTION ( 'NONE',  ( 0.000000000000000000, 0.000000000000000000, 1.000000000000000000 ) ) ;
#17790=CIRCLE ( 'NONE', #14738, 1.500000000000000888 ) ;
#17791=EDGE_LOOP ( 'NONE', ( #10604, #2657 ) ) ;
#17792=CARTESIAN_POINT ( 'NONE',  ( 6.831828081324923474, -76.87160051972034580, -17.32050807568878525 ) ) ;
#17793=AXIS2_PLACEMENT_3D ( 'NONE', #6733, #9364, #13516 ) ;
#17794=FACE_BOUND ( 'NONE', #10456, .T. ) ;
#17795=VECTOR ( 'NONE', #16471, 1000.000000000000000 ) ;
#17796=VECTOR ( 'NONE', #2820, 1000.000000000000000 ) ;
#17798=DIRECTION ( 'NONE',  ( 0.000000000000000000, 0.000000000000000000, 1.000000000000000000 ) ) ;
#17799=CYLINDRICAL_SURFACE ( 'NONE', #12372, 1.500000000000001554 ) ;
#17800=DIRECTION ( 'NONE',  ( -0.1566598588826321192, 0.9876526153536342445, 7.798540720466730171E-17 ) ) ;
#17801=AXIS2_PLACEMENT_3D ( 'NONE', #15665, #4392, #50 ) ;
#17802=DIRECTION ( 'NONE',  ( -0.1566598588826321192, 0.9876526153536342445, 7.798540720466731404E-17 ) ) ;
#17806=ORIENTED_EDGE ( 'NONE', *, *, #15829, .F. ) ;
#17807=VERTEX_POINT ( 'NONE', #16070 ) ;
#17808=CARTESIAN_POINT ( 'NONE',  ( -26.74836084069852404, -82.19803572172983763, -21.65063509461098690 ) ) ;
#17809=EDGE_CURVE ( 'NONE', #4926, #3971, #5682, .T. ) ;
#17810=EDGE_LOOP ( 'NONE', ( #6189, #1743, #7222, #14512 ) ) ;
#17811=AXIS2_PLACEMENT_3D ( 'NONE', #8600, #1396, #7181 ) ;
#17812=EDGE_CURVE ( 'NONE', #2898, #11338, #14008, .T. ) ;
#17813=ORIENTED_EDGE ( 'NONE', *, *, #8908, .T. ) ;
#17814=CARTESIAN_POINT ( 'NONE',  ( -48.02252708097940825, -27.86704125135829813, -8.660254037844380193 ) ) ;
#17816=VERTEX_POINT ( 'NONE', #14366 ) ;
#17817=DIRECTION ( 'NONE',  ( -0.9876526153536341335, -0.1566598588826327021, 0.000000000000000000 ) ) ;
#17818=DIRECTION ( 'NONE',  ( -0.1566598588826321192, 0.9876526153536342445, 7.798540720466731404E-17 ) ) ;
#17819=EDGE_LOOP ( 'NONE', ( #1392, #4555 ) ) ;
#17821=AXIS2_PLACEMENT_3D ( 'NONE', #18020, #4977, #16571 ) ;
#17822=CARTESIAN_POINT ( 'NONE',  ( -58.68235252892886678, -24.49537676341647696, -17.32050807568878170 ) ) ;
#17823=CARTESIAN_POINT ( 'NONE',  ( -41.56315007100297265, -84.54793360496931598, -21.65063509461098690 ) ) ;
#17824=FACE_BOUND ( 'NONE', #1292, .T. ) ;
#17825=DIRECTION ( 'NONE',  ( -0.1566598588826321192, 0.9876526153536342445, 7.798540720466730171E-17 ) ) ;
#17826=CARTESIAN_POINT ( 'NONE',  ( -67.24211807019732134, -88.62108993591773753, -17.32050807568878525 ) ) ;
#17827=DIRECTION ( 'NONE',  ( -0.1566598588826321192, 0.9876526153536342445, 7.798540720466730171E-17 ) ) ;
#17828=EDGE_LOOP ( 'NONE', ( #11454, #6890 ) ) ;
#17829=AXIS2_PLACEMENT_3D ( 'NONE', #12577, #10969, #14017 ) ;
#17830=DIRECTION ( 'NONE',  ( -0.1566598588826321192, 0.9876526153536342445, 7.798540720466731404E-17 ) ) ;
#17831=EDGE_CURVE ( 'NONE', #8230, #9109, #1437, .T. ) ;
#17832=ORIENTED_EDGE ( 'NONE', *, *, #1471, .T. ) ;
#17833=ORIENTED_EDGE ( 'NONE', *, *, #13522, .T. ) ;
#17834=DIRECTION ( 'NONE',  ( -0.1566598588826321192, 0.9876526153536342445, 7.798540720466730171E-17 ) ) ;
#17836=DIRECTION ( 'NONE',  ( -0.9876526153536336894, -0.1566598588826350336, 0.000000000000000000 ) ) ;
#17838=CIRCLE ( 'NONE', #15082, 1.500000000000000888 ) ;
#17839=ORIENTED_EDGE ( 'NONE', *, *, #13276, .F. ) ;
#17841=VECTOR ( 'NONE', #5242, 1000.000000000000000 ) ;
#17842=CARTESIAN_POINT ( 'NONE',  ( -31.72625892764450484, -25.28215357979487266, -8.660254037844380193 ) ) ;
#17843=CARTESIAN_POINT ( 'NONE',  ( -10.98555400521827963, -21.99229654325962002, -4.330127018922181215 ) ) ;
#17845=DIRECTION ( 'NONE',  ( -0.1566598588826321192, 0.9876526153536342445, 7.798540720466731404E-17 ) ) ;
#17846=CARTESIAN_POINT ( 'NONE',  ( -62.79768130110601021, -87.91612057094592103, 12.99038105676661203 ) ) ;
#17848=ORIENTED_EDGE ( 'NONE', *, *, #10351, .F. ) ;
#17849=CIRCLE ( 'NONE', #3873, 1.500000000000000888 ) ;
#17850=CARTESIAN_POINT ( 'NONE',  ( -5.842937607509656850, -16.11407431319567962, -17.32050807568878170 ) ) ;
#17851=ORIENTED_EDGE ( 'NONE', *, *, #4273, .T. ) ;
#17852=CARTESIAN_POINT ( 'NONE',  ( -34.97868976044173195, -20.73554015023333363, 12.99038105676661736 ) ) ;
#17854=AXIS2_PLACEMENT_3D ( 'NONE', #971, #2467, #11161 ) ;
#17855=CARTESIAN_POINT ( 'NONE',  ( -55.22556837519117323, -23.94706725732726937, -8.660254037844380193 ) ) ;
#17858=EDGE_LOOP ( 'NONE', ( #13555, #9558, #17201, #6996 ) ) ;
#17859=ORIENTED_EDGE ( 'NONE', *, *, #3540, .F. ) ;
#17860=CYLINDRICAL_SURFACE ( 'NONE', #6555, 1.500000000000001554 ) ;
#17861=EDGE_CURVE ( 'NONE', #8059, #4101, #3817, .T. ) ;
#17862=EDGE_CURVE ( 'NONE', #6801, #442, #8687, .T. ) ;
#17863=ORIENTED_EDGE ( 'NONE', *, *, #3619, .T. ) ;
#17864=FACE_BOUND ( 'NONE', #9062, .T. ) ;
#17866=AXIS2_PLACEMENT_3D ( 'NONE', #5543, #14435, #11576 ) ;
#17867=CARTESIAN_POINT ( 'NONE',  ( -13.41505053342451426, -80.08312762681431707, -21.65063509461098690 ) ) ;
#17868=AXIS2_PLACEMENT_3D ( 'NONE', #2363, #3685, #15255 ) ;
#17869=ORIENTED_EDGE ( 'NONE', *, *, #8296, .F. ) ;
#17870=CIRCLE ( 'NONE', #9682, 1.500000000000000444 ) ;
#17871=VECTOR ( 'NONE', #15691, 1000.000000000000000 ) ;
#17872=AXIS2_PLACEMENT_3D ( 'NONE', #9524, #9892, #920 ) ;
#17873=CIRCLE ( 'NONE', #9689, 1.500000000000000888 ) ;
#17874=EDGE_LOOP ( 'NONE', ( #2445, #13543 ) ) ;
#17875=CARTESIAN_POINT ( 'NONE',  ( -52.42732883989287274, -86.27119205267827340, 17.32050807568881368 ) ) ;
#17878=VERTEX_POINT ( 'NONE', #1391 ) ;
#17879=DIRECTION ( 'NONE',  ( -0.9876526153536336894, -0.1566598588826349503, 0.000000000000000000 ) ) ;
#17880=ORIENTED_EDGE ( 'NONE', *, *, #10577, .T. ) ;
#17881=DIRECTION ( 'NONE',  ( 0.000000000000000000, 0.000000000000000000, 1.000000000000000000 ) ) ;
#17882=DIRECTION ( 'NONE',  ( -0.1566598588826321747, 0.9876526153536343555, 0.000000000000000000 ) ) ;
#17883=AXIS2_PLACEMENT_3D ( 'NONE', #5403, #2644, #18341 ) ;
#17884=FACE_OUTER_BOUND ( 'NONE', #16815, .T. ) ;
#17885=DIRECTION ( 'NONE',  ( -0.000000000000000000, -0.000000000000000000, -1.000000000000000000 ) ) ;
#17886=ORIENTED_EDGE ( 'NONE', *, *, #8806, .F. ) ;
#17887=ORIENTED_EDGE ( 'NONE', *, *, #3274, .T. ) ;
#17889=ADVANCED_FACE ( 'NONE', ( #8762 ), #1661, .F. ) ;
#17891=AXIS2_PLACEMENT_3D ( 'NONE', #13561, #8857, #13384 ) ;
#17892=DIRECTION ( 'NONE',  ( -0.1566598588826321192, 0.9876526153536342445, 7.798540720466730171E-17 ) ) ;
#17894=CIRCLE ( 'NONE', #13005, 1.499999999999999556 ) ;
#17895=ADVANCED_FACE ( 'NONE', ( #7440 ), #13114, .F. ) ;
#17896=ORIENTED_EDGE ( 'NONE', *, *, #4609, .T. ) ;
#17899=ORIENTED_EDGE ( 'NONE', *, *, #7312, .F. ) ;
#17900=CIRCLE ( 'NONE', #9709, 1.500000000000001332 ) ;
#17903=LINE ( 'NONE', #6222, #16639 ) ;
#17904=CIRCLE ( 'NONE', #13312, 1.500000000000000888 ) ;
#17905=DIRECTION ( 'NONE',  ( -0.1566598588826321192, 0.9876526153536342445, 7.798540720466730171E-17 ) ) ;
#17906=VECTOR ( 'NONE', #12258, 1000.000000000000000 ) ;
#17908=LINE ( 'NONE', #17999, #12858 ) ;
#17909=DIRECTION ( 'NONE',  ( 0.000000000000000000, 0.000000000000000000, 1.000000000000000000 ) ) ;
#17910=ORIENTED_EDGE ( 'NONE', *, *, #7361, .T. ) ;
#17911=ORIENTED_EDGE ( 'NONE', *, *, #3676, .T. ) ;
#17912=CARTESIAN_POINT ( 'NONE',  ( -41.39843176024034221, -21.75382923297042481, -21.65063509461097979 ) ) ;
#17914=EDGE_LOOP ( 'NONE', ( #5627, #2040, #11490, #13643 ) ) ;
#17915=ORIENTED_EDGE ( 'NONE', *, *, #872, .F. ) ;
#17916=AXIS2_PLACEMENT_3D ( 'NONE', #2615, #8682, #4112 ) ;
#17919=FACE_OUTER_BOUND ( 'NONE', #16160, .T. ) ;
#17920=ADVANCED_FACE ( 'NONE', ( #12920 ), #6014, .F. ) ;
#17921=AXIS2_PLACEMENT_3D ( 'NONE', #15509, #2428, #8215 ) ;
#17922=EDGE_LOOP ( 'NONE', ( #17663, #5438 ) ) ;
#17923=DIRECTION ( 'NONE',  ( -0.1566598588826321192, 0.9876526153536342445, 7.798540720466730171E-17 ) ) ;
#17924=EDGE_CURVE ( 'NONE', #5396, #8469, #9302, .T. ) ;
#17925=FACE_OUTER_BOUND ( 'NONE', #15361, .T. ) ;
#17926=CYLINDRICAL_SURFACE ( 'NONE', #2187, 1.500000000000001554 ) ;
#17927=CARTESIAN_POINT ( 'NONE',  ( -70.24471092643608472, -31.39188807621751209, -21.65063509461098334 ) ) ;
#17928=AXIS2_PLACEMENT_3D ( 'NONE', #15996, #17076, #5787 ) ;
#17929=EDGE_CURVE ( 'NONE', #8901, #6017, #6909, .T. ) ;
#17930=DIRECTION ( 'NONE',  ( -0.1566598588826321192, 0.9876526153536342445, 7.798540720466731404E-17 ) ) ;
#17931=CARTESIAN_POINT ( 'NONE',  ( -64.60826822105063627, -25.43533591671227967, 4.330127018922218518 ) ) ;
#17932=DIRECTION ( 'NONE',  ( -0.1566598588826321192, 0.9876526153536342445, 7.798540720466731404E-17 ) ) ;
#17933=EDGE_LOOP ( 'NONE', ( #13620, #10788, #1060, #2141 ) ) ;
#17936=CARTESIAN_POINT ( 'NONE',  ( -4.526176995241833367, -78.67318889687062722, 17.32050807568880657 ) ) ;
#17937=DIRECTION ( 'NONE',  ( -0.9876526153536336894, -0.1566598588826349503, 0.000000000000000000 ) ) ;
#17938=ORIENTED_EDGE ( 'NONE', *, *, #9265, .F. ) ;
#17939=CYLINDRICAL_SURFACE ( 'NONE', #3228, 1.500000000000000888 ) ;
#17940=ORIENTED_EDGE ( 'NONE', *, *, #5040, .T. ) ;
#17941=VERTEX_POINT ( 'NONE', #11764 ) ;
#17942=AXIS2_PLACEMENT_3D ( 'NONE', #5506, #8150, #11346 ) ;
#17943=DIRECTION ( 'NONE',  ( -0.1566598588826321747, 0.9876526153536343555, 0.000000000000000000 ) ) ;
#17944=VERTEX_POINT ( 'NONE', #2808 ) ;
#17945=AXIS2_PLACEMENT_3D ( 'NONE', #15342, #18243, #2354 ) ;
#17946=CARTESIAN_POINT ( 'NONE',  ( -45.55339554259532520, -27.47539160415171722, 21.65063509461101887 ) ) ;
#17949=EDGE_CURVE ( 'NONE', #1506, #12466, #231, .T. ) ;
#17951=CARTESIAN_POINT ( 'NONE',  ( -3.578159390066044665, -20.81734760163988440, 1.522258424776792809E-14 ) ) ;
#17953=ORIENTED_EDGE ( 'NONE', *, *, #6239, .T. ) ;
#17956=ORIENTED_EDGE ( 'NONE', *, *, #807, .T. ) ;
#17959=LINE ( 'NONE', #774, #5436 ) ;
#17961=VERTEX_POINT ( 'NONE', #5750 ) ;
#17962=ORIENTED_EDGE ( 'NONE', *, *, #4777, .T. ) ;
#17963=CARTESIAN_POINT ( 'NONE',  ( -29.21749237908258223, -82.58968536893642920, 8.660254037844412167 ) ) ;
#17964=FACE_BOUND ( 'NONE', #7815, .T. ) ;
#17965=CARTESIAN_POINT ( 'NONE',  ( -79.13358446461874962, -32.80182680616118773, -17.32050807568878170 ) ) ;
#17969=FACE_BOUND ( 'NONE', #3075, .T. ) ;
#17970=ORIENTED_EDGE ( 'NONE', *, *, #9153, .T. ) ;
#17972=LINE ( 'NONE', #12031, #15752 ) ;
#17974=CARTESIAN_POINT ( 'NONE',  ( -57.20087360589841552, -24.26038697509253339, -17.32050807568878170 ) ) ;
#17975=ADVANCED_FACE ( 'NONE', ( #15876 ), #2877, .F. ) ;
#17977=CARTESIAN_POINT ( 'NONE',  ( -11.76885329963143434, -17.05403346649147878, -4.330127018922180326 ) ) ;
#17978=EDGE_LOOP ( 'NONE', ( #3405, #16629, #17675, #16421 ) ) ;
#17979=EDGE_LOOP ( 'NONE', ( #687, #17863, #15567, #11664 ) ) ;
#17981=LINE ( 'NONE', #10547, #843 ) ;
#17982=CYLINDRICAL_SURFACE ( 'NONE', #14455, 1.500000000000001554 ) ;
#17983=ORIENTED_EDGE ( 'NONE', *, *, #3998, .F. ) ;
#17984=VECTOR ( 'NONE', #6077, 1000.000000000000000 ) ;
#17986=DIRECTION ( 'NONE',  ( -0.1566598588826321192, 0.9876526153536342445, 7.798540720466730171E-17 ) ) ;
#17988=FACE_OUTER_BOUND ( 'NONE', #17195, .T. ) ;
#17989=CARTESIAN_POINT ( 'NONE',  ( -29.21749237908259644, -82.58968536893641499, -17.32050807568878525 ) ) ;
#17992=VERTEX_POINT ( 'NONE', #10723 ) ;
#17994=VECTOR ( 'NONE', #7957, 1000.000000000000000 ) ;
#17995=EDGE_CURVE ( 'NONE', #5108, #11461, #3532, .T. ) ;
#17996=CARTESIAN_POINT ( 'NONE',  ( -72.50948914387967648, -26.68861478777332863, 4.330127018922218518 ) ) ;
#17997=DIRECTION ( 'NONE',  ( 0.000000000000000000, 0.000000000000000000, 1.000000000000000000 ) ) ;
#17998=DIRECTION ( 'NONE',  ( -0.9876526153536336894, -0.1566598588826349503, 0.000000000000000000 ) ) ;
#17999=CARTESIAN_POINT ( 'NONE',  ( 1.399738696879940791, -77.73322974357483872, 4.330127018922209636 ) ) ;
#18001=VERTEX_POINT ( 'NONE', #16447 ) ;
#18002=DIRECTION ( 'NONE',  ( -0.1566598588826321192, 0.9876526153536342445, 7.798540720466730171E-17 ) ) ;
#18003=VERTEX_POINT ( 'NONE', #11939 ) ;
#18004=VERTEX_POINT ( 'NONE', #7721 ) ;
#18005=CARTESIAN_POINT ( 'NONE',  ( -55.42992169613162190, -29.04199019297804085, 12.99038105676661736 ) ) ;
#18006=VERTEX_POINT ( 'NONE', #6494 ) ;
#18008=DIRECTION ( 'NONE',  ( -0.1566598588826321747, 0.9876526153536343555, 0.000000000000000000 ) ) ;
#18009=VERTEX_POINT ( 'NONE', #713 ) ;
#18010=CARTESIAN_POINT ( 'NONE',  ( -81.73462711737164454, 33.01666666666666572, 35.00000000000000000 ) ) ;
#18011=CARTESIAN_POINT ( 'NONE',  ( -30.69897130211304770, -82.82467515726037277, -17.32050807568878525 ) ) ;
#18012=EDGE_LOOP ( 'NONE', ( #18087, #4661 ) ) ;
#18013=FACE_OUTER_BOUND ( 'NONE', #8653, .T. ) ;
#18015=ORIENTED_EDGE ( 'NONE', *, *, #17101, .T. ) ;
#18016=CARTESIAN_POINT ( 'NONE',  ( -67.07739975943471222, -25.82698556391884992, -17.32050807568878170 ) ) ;
#18017=FACE_OUTER_BOUND ( 'NONE', #8031, .T. ) ;
#18018=CYLINDRICAL_SURFACE ( 'NONE', #3784, 1.500000000000001554 ) ;
#18019=FACE_BOUND ( 'NONE', #6096, .T. ) ;
#18020=CARTESIAN_POINT ( 'NONE',  ( -6.830590222863280658, -16.27073417207831696, 12.99038105676661026 ) ) ;
#18021=CYLINDRICAL_SURFACE ( 'NONE', #1822, 1.500000000000001554 ) ;
#18022=CARTESIAN_POINT ( 'NONE',  ( -53.94844277310118486, -28.80700040465408662, -4.330127018922181215 ) ) ;
#18024=ORIENTED_EDGE ( 'NONE', *, *, #13156, .T. ) ;
#18025=EDGE_CURVE ( 'NONE', #16064, #4400, #3515, .T. ) ;
#18026=ADVANCED_FACE ( 'NONE', ( #12231 ), #6214, .F. ) ;
#18028=DIRECTION ( 'NONE',  ( -0.1566598588826321192, 0.9876526153536342445, 7.798540720466730171E-17 ) ) ;
#18029=CIRCLE ( 'NONE', #13440, 1.500000000000000444 ) ;
#18030=ORIENTED_EDGE ( 'NONE', *, *, #8697, .F. ) ;
#18031=ORIENTED_EDGE ( 'NONE', *, *, #8467, .T. ) ;
#18032=LINE ( 'NONE', #15241, #16403 ) ;
#18033=ORIENTED_EDGE ( 'NONE', *, *, #8262, .F. ) ;
#18034=DIRECTION ( 'NONE',  ( -0.1566598588826321192, 0.9876526153536342445, 7.798540720466730171E-17 ) ) ;
#18035=DIRECTION ( 'NONE',  ( -0.9876526153536336894, -0.1566598588826349503, 0.000000000000000000 ) ) ;
#18036=DIRECTION ( 'NONE',  ( -0.1566598588826321747, 0.9876526153536343555, 0.000000000000000000 ) ) ;
#18039=DIRECTION ( 'NONE',  ( -0.9876526153536341335, -0.1566598588826327021, 0.000000000000000000 ) ) ;
#18041=ORIENTED_EDGE ( 'NONE', *, *, #14992, .F. ) ;
#18042=FACE_OUTER_BOUND ( 'NONE', #15872, .T. ) ;
#18043=ORIENTED_EDGE ( 'NONE', *, *, #17929, .F. ) ;
#18044=DIRECTION ( 'NONE',  ( -0.1566598588826321747, 0.9876526153536343555, 0.000000000000000000 ) ) ;
#18045=DIRECTION ( 'NONE',  ( -0.9876526153536341335, -0.1566598588826327021, 0.000000000000000000 ) ) ;
#18046=CARTESIAN_POINT ( 'NONE',  ( -63.62061560569701157, -25.27867605782964588, 8.660254037844417496 ) ) ;
#18047=EDGE_CURVE ( 'NONE', #3060, #4754, #7796, .T. ) ;
#18051=FACE_OUTER_BOUND ( 'NONE', #18117, .T. ) ;
#18052=EDGE_CURVE ( 'NONE', #8214, #5148, #8405, .T. ) ;
#18054=FACE_BOUND ( 'NONE', #11842, .T. ) ;
#18055=DIRECTION ( 'NONE',  ( -0.1566598588826321192, 0.9876526153536342445, 7.798540720466730171E-17 ) ) ;
#18057=CARTESIAN_POINT ( 'NONE',  ( -7.034943543803747090, -21.36565710772908488, 8.660254037844413944 ) ) ;
#18058=ORIENTED_EDGE ( 'NONE', *, *, #2766, .T. ) ;
#18059=FACE_OUTER_BOUND ( 'NONE', #9234, .T. ) ;
#18060=VECTOR ( 'NONE', #18295, 1000.000000000000000 ) ;
#18061=LINE ( 'NONE', #5023, #17281 ) ;
#18063=DIRECTION ( 'NONE',  ( -0.9876526153536341335, 0.1566598588826326743, -0.000000000000000000 ) ) ;
#18065=ORIENTED_EDGE ( 'NONE', *, *, #5243, .T. ) ;
#18067=CARTESIAN_POINT ( 'NONE',  ( -71.23236354178970942, -31.54854793510013877, 17.32050807568881723 ) ) ;
#18068=LINE ( 'NONE', #16627, #5697 ) ;
#18069=ORIENTED_EDGE ( 'NONE', *, *, #7358, .F. ) ;
#18070=CARTESIAN_POINT ( 'NONE',  ( -78.43540483600145308, -27.62857394106911713, 1.908195823574487804E-14 ) ) ;
#18071=VECTOR ( 'NONE', #16057, 1000.000000000000000 ) ;
#18072=ADVANCED_FACE ( 'NONE', ( #13472 ), #6117, .F. ) ;
#18073=DIRECTION ( 'NONE',  ( -0.1566598588826321192, 0.9876526153536342445, 7.798540720466730171E-17 ) ) ;
#18075=VERTEX_POINT ( 'NONE', #10650 ) ;
#18076=CIRCLE ( 'NONE', #9870, 1.500000000000001332 ) ;
#18077=EDGE_CURVE ( 'NONE', #968, #8399, #1448, .T. ) ;
#18080=LINE ( 'NONE', #16645, #12957 ) ;
#18082=DIRECTION ( 'NONE',  ( -0.9876526153536336894, -0.1566598588826349503, 0.000000000000000000 ) ) ;
#18083=CARTESIAN_POINT ( 'NONE',  ( -25.26688191766805858, -81.96304593340589406, -12.99038105676658539 ) ) ;
#18085=DIRECTION ( 'NONE',  ( -0.1566598588826321192, 0.9876526153536342445, 7.798540720466730171E-17 ) ) ;
#18086=DIRECTION ( 'NONE',  ( -0.9876526153536336894, -0.1566598588826350336, 0.000000000000000000 ) ) ;
#18087=ORIENTED_EDGE ( 'NONE', *, *, #4064, .F. ) ;
#18088=ORIENTED_EDGE ( 'NONE', *, *, #6482, .F. ) ;
#18090=AXIS2_PLACEMENT_3D ( 'NONE', #5078, #11045, #15229 ) ;
#18091=FACE_OUTER_BOUND ( 'NONE', #12972, .T. ) ;
#18092=VERTEX_POINT ( 'NONE', #15095 ) ;
#18094=ORIENTED_EDGE ( 'NONE', *, *, #17129, .F. ) ;
#18095=AXIS2_PLACEMENT_3D ( 'NONE', #17251, #12936, #10378 ) ;
#18096=EDGE_CURVE ( 'NONE', #7506, #8207, #10799, .T. ) ;
#18097=ADVANCED_FACE ( 'NONE', ( #3155 ), #17982, .F. ) ;
#18099=DIRECTION ( 'NONE',  ( 0.000000000000000000, 0.000000000000000000, 1.000000000000000000 ) ) ;
#18100=EDGE_CURVE ( 'NONE', #1829, #16999, #12619, .T. ) ;
#18101=DIRECTION ( 'NONE',  ( 0.000000000000000000, 0.000000000000000000, 1.000000000000000000 ) ) ;
#18102=EDGE_CURVE ( 'NONE', #16138, #14196, #9002, .T. ) ;
#18103=DIRECTION ( 'NONE',  ( -0.1566598588826321747, 0.9876526153536343555, 0.000000000000000000 ) ) ;
#18105=DIRECTION ( 'NONE',  ( -0.1566598588826321192, 0.9876526153536342445, 7.798540720466730171E-17 ) ) ;
#18107=CIRCLE ( 'NONE', #17793, 1.500000000000000888 ) ;
#18108=ORIENTED_EDGE ( 'NONE', *, *, #15843, .F. ) ;
#18109=DIRECTION ( 'NONE',  ( -0.1566598588826321747, 0.9876526153536343555, 0.000000000000000000 ) ) ;
#18110=VERTEX_POINT ( 'NONE', #9040 ) ;
#18111=DIRECTION ( 'NONE',  ( 0.000000000000000000, 0.000000000000000000, 1.000000000000000000 ) ) ;
#18112=FACE_BOUND ( 'NONE', #12358, .T. ) ;
#18113=CIRCLE ( 'NONE', #9902, 1.500000000000001332 ) ;
#18114=CYLINDRICAL_SURFACE ( 'NONE', #16600, 1.500000000000001554 ) ;
#18115=CARTESIAN_POINT ( 'NONE',  ( -64.60826822105062206, -25.43533591671228677, 21.65063509461101887 ) ) ;
#18116=CARTESIAN_POINT ( 'NONE',  ( -75.18297400320422241, -32.17518737063066681, 4.330127018922217630 ) ) ;
#18117=EDGE_LOOP ( 'NONE', ( #7717, #11751, #9596, #4789 ) ) ;
#18118=CARTESIAN_POINT ( 'NONE',  ( -12.46703292824873088, -22.22728633158356359, -12.99038105676658006 ) ) ;
#18120=AXIS2_PLACEMENT_3D ( 'NONE', #11865, #13572, #517 ) ;
#18121=EDGE_CURVE ( 'NONE', #8348, #5828, #1843, .T. ) ;
#18124=DIRECTION ( 'NONE',  ( -0.9876526153536341335, -0.1566598588826327021, 0.000000000000000000 ) ) ;
#18125=EDGE_CURVE ( 'NONE', #3927, #3563, #11991, .T. ) ;
#18128=CARTESIAN_POINT ( 'NONE',  ( 0.000000000000000000, 0.000000000000000000, 30.00000000000000000 ) ) ;
#18131=DIRECTION ( 'NONE',  ( -0.1566598588826321192, 0.9876526153536342445, 7.798540720466730171E-17 ) ) ;
#18132=CARTESIAN_POINT ( 'NONE',  ( -73.70149508017377116, -31.94019758230671258, 12.99038105676661736 ) ) ;
#18134=EDGE_CURVE ( 'NONE', #17191, #8885, #10515, .T. ) ;
#18137=DIRECTION ( 'NONE',  ( 0.000000000000000000, 0.000000000000000000, 1.000000000000000000 ) ) ;
#18138=ORIENTED_EDGE ( 'NONE', *, *, #16117, .F. ) ;
#18139=CIRCLE ( 'NONE', #11713, 1.500000000000001332 ) ;
#18140=CARTESIAN_POINT ( 'NONE',  ( -7.528769851480577202, -21.44398703717040888, 12.99038105676661026 ) ) ;
#18141=DIRECTION ( 'NONE',  ( -0.9876526153536341335, -0.1566598588826327021, 0.000000000000000000 ) ) ;
#18142=DIRECTION ( 'NONE',  ( -0.9876526153536341335, -0.1566598588826327021, 0.000000000000000000 ) ) ;
#18143=EDGE_LOOP ( 'NONE', ( #4899, #14030, #2000, #15349 ) ) ;
#18145=AXIS2_PLACEMENT_3D ( 'NONE', #15091, #2117, #2387 ) ;
#18146=EDGE_LOOP ( 'NONE', ( #14002, #17455 ) ) ;
#18147=ORIENTED_EDGE ( 'NONE', *, *, #3692, .F. ) ;
#18149=ORIENTED_EDGE ( 'NONE', *, *, #11014, .T. ) ;
#18151=AXIS2_PLACEMENT_3D ( 'NONE', #15248, #3761, #9281 ) ;
#18152=AXIS2_PLACEMENT_3D ( 'NONE', #8281, #6862, #18167 ) ;
#18154=FACE_BOUND ( 'NONE', #13347, .T. ) ;
#18156=CARTESIAN_POINT ( 'NONE',  ( -77.65210554158829837, -32.56683701783724416, 1.869203119972154228E-14 ) ) ;
#18158=CIRCLE ( 'NONE', #13258, 1.500000000000000444 ) ;
#18159=ADVANCED_FACE ( 'NONE', ( #5248 ), #15197, .F. ) ;
#18160=ORIENTED_EDGE ( 'NONE', *, *, #6948, .F. ) ;
#18161=VECTOR ( 'NONE', #13143, 1000.000000000000000 ) ;
#18162=EDGE_CURVE ( 'NONE', #16065, #15050, #6685, .T. ) ;
#18163=DIRECTION ( 'NONE',  ( -0.1566598588826321192, 0.9876526153536342445, 7.798540720466730171E-17 ) ) ;
#18165=EDGE_LOOP ( 'NONE', ( #10492, #8074 ) ) ;
#18166=DIRECTION ( 'NONE',  ( -0.1566598588826321192, 0.9876526153536342445, 7.798540720466730171E-17 ) ) ;
#18167=DIRECTION ( 'NONE',  ( -0.9876526153536336894, -0.1566598588826349503, 0.000000000000000000 ) ) ;
#18168=CARTESIAN_POINT ( 'NONE',  ( -67.77557938805200877, -31.00023842901093118, -8.660254037844380193 ) ) ;
#18169=ORIENTED_EDGE ( 'NONE', *, *, #13307, .F. ) ;
#18170=EDGE_LOOP ( 'NONE', ( #4495, #10764, #9610, #1310 ) ) ;
#18172=CARTESIAN_POINT ( 'NONE',  ( -68.55887868246516348, -26.06197535224280060, 1.908195823574487804E-14 ) ) ;
#18173=EDGE_LOOP ( 'NONE', ( #18638, #9498 ) ) ;
#18175=ORIENTED_EDGE ( 'NONE', *, *, #12985, .F. ) ;
#18176=DIRECTION ( 'NONE',  ( -0.9876526153536336894, -0.1566598588826349503, 0.000000000000000000 ) ) ;
#18177=ORIENTED_EDGE ( 'NONE', *, *, #18655, .F. ) ;
#18178=AXIS2_PLACEMENT_3D ( 'NONE', #5226, #15352, #877 ) ;
#18179=EDGE_LOOP ( 'NONE', ( #7786, #5921, #3920, #8395 ) ) ;
#18181=CIRCLE ( 'NONE', #9958, 1.500000000000000888 ) ;
#18182=ORIENTED_EDGE ( 'NONE', *, *, #23, .F. ) ;
#18183=VECTOR ( 'NONE', #1202, 1000.000000000000000 ) ;
#18184=VECTOR ( 'NONE', #16115, 1000.000000000000000 ) ;
#18185=CIRCLE ( 'NONE', #9963, 1.500000000000000444 ) ;
#18186=FACE_BOUND ( 'NONE', #12121, .T. ) ;
#18187=FACE_OUTER_BOUND ( 'NONE', #5647, .T. ) ;
#18188=LINE ( 'NONE', #6787, #9026 ) ;
#18190=CIRCLE ( 'NONE', #615, 1.500000000000000888 ) ;
#18191=AXIS2_PLACEMENT_3D ( 'NONE', #936, #18307, #8218 ) ;
#18193=LINE ( 'NONE', #16937, #605 ) ;
#18194=AXIS2_PLACEMENT_3D ( 'NONE', #3507, #3882, #9707 ) ;
#18195=DIRECTION ( 'NONE',  ( -0.1566598588826321192, 0.9876526153536342445, 7.798540720466730171E-17 ) ) ;
#18196=ORIENTED_EDGE ( 'NONE', *, *, #12149, .T. ) ;
#18197=LINE ( 'NONE', #5170, #12989 ) ;
#18198=CARTESIAN_POINT ( 'NONE',  ( -37.61253960958845255, -83.92129416943878084, -17.32050807568878525 ) ) ;
#18200=VERTEX_POINT ( 'NONE', #18278 ) ;
#18201=EDGE_LOOP ( 'NONE', ( #9163, #12896, #1955, #13019 ) ) ;
#18203=DIRECTION ( 'NONE',  ( -0.9876526153536344665, -0.1566598588826304539, 0.000000000000000000 ) ) ;
#18205=AXIS2_PLACEMENT_3D ( 'NONE', #4698, #4424, #10304 ) ;
#18206=ORIENTED_EDGE ( 'NONE', *, *, #10634, .T. ) ;
#18207=EDGE_CURVE ( 'NONE', #3520, #98, #2652, .T. ) ;
#18208=ORIENTED_EDGE ( 'NONE', *, *, #8341, .T. ) ;
#18209=DIRECTION ( 'NONE',  ( -0.9876526153536336894, -0.1566598588826349503, 0.000000000000000000 ) ) ;
#18210=DIRECTION ( 'NONE',  ( -0.9876526153536341335, -0.1566598588826327021, 0.000000000000000000 ) ) ;
#18211=EDGE_LOOP ( 'NONE', ( #11812, #10237 ) ) ;
#18212=VECTOR ( 'NONE', #15231, 1000.000000000000000 ) ;
#18213=CARTESIAN_POINT ( 'NONE',  ( -7.034943543803747090, -21.36565710772908488, -17.32050807568878170 ) ) ;
#18214=ORIENTED_EDGE ( 'NONE', *, *, #3792, .F. ) ;
#18215=AXIS2_PLACEMENT_3D ( 'NONE', #9789, #16726, #5330 ) ;
#18216=DIRECTION ( 'NONE',  ( -0.1566598588826321192, 0.9876526153536342445, 7.798540720466731404E-17 ) ) ;
#18218=AXIS2_PLACEMENT_3D ( 'NONE', #6545, #4992, #1897 ) ;
#18219=DIRECTION ( 'NONE',  ( -0.1566598588826321192, 0.9876526153536342445, 7.798540720466731404E-17 ) ) ;
#18220=EDGE_LOOP ( 'NONE', ( #15367, #3013, #16503, #7760 ) ) ;
#18221=CARTESIAN_POINT ( 'NONE',  ( -40.61513246582718040, -26.69209230973856251, 12.99038105676661736 ) ) ;
#18222=VERTEX_POINT ( 'NONE', #12611 ) ;
#18223=CYLINDRICAL_SURFACE ( 'NONE', #3503, 1.500000000000001554 ) ;
#18224=DIRECTION ( 'NONE',  ( -0.9876526153536336894, -0.1566598588826349503, 0.000000000000000000 ) ) ;
#18225=PLANE ( 'NONE',  #16075 ) ;
#18226=EDGE_CURVE ( 'NONE', #9762, #8333, #9713, .T. ) ;
#18229=VERTEX_POINT ( 'NONE', #5033 ) ;
#18230=ADVANCED_FACE ( 'NONE', ( #13751 ), #3709, .F. ) ;
#18232=AXIS2_PLACEMENT_3D ( 'NONE', #367, #8891, #7471 ) ;
#18233=CYLINDRICAL_SURFACE ( 'NONE', #941, 1.500000000000001554 ) ;
#18234=ORIENTED_EDGE ( 'NONE', *, *, #4912, .F. ) ;
#18235=EDGE_LOOP ( 'NONE', ( #9338, #6210 ) ) ;
#18238=DIRECTION ( 'NONE',  ( -0.1566598588826321192, 0.9876526153536342445, 7.798540720466730171E-17 ) ) ;
#18239=AXIS2_PLACEMENT_3D ( 'NONE', #9737, #2519, #12630 ) ;
#18241=ORIENTED_EDGE ( 'NONE', *, *, #2967, .T. ) ;
#18242=CARTESIAN_POINT ( 'NONE',  ( -10.45209268736360997, -79.61314805016641571, -4.330127018922185655 ) ) ;
#18243=DIRECTION ( 'NONE',  ( -0.1566598588826321192, 0.9876526153536342445, 7.798540720466731404E-17 ) ) ;
#18245=CIRCLE ( 'NONE', #5183, 1.500000000000000888 ) ;
#18247=CARTESIAN_POINT ( 'NONE',  ( -71.72618984946653597, -31.62687786454144856, -4.330127018922181215 ) ) ;
#18250=EDGE_CURVE ( 'NONE', #3501, #2218, #18068, .T. ) ;
#18251=ORIENTED_EDGE ( 'NONE', *, *, #2059, .T. ) ;
#18252=VECTOR ( 'NONE', #15010, 1000.000000000000000 ) ;
#18253=EDGE_CURVE ( 'NONE', #8678, #9632, #11105, .T. ) ;
#18254=DIRECTION ( 'NONE',  ( -0.1566598588826321192, 0.9876526153536342445, 7.798540720466730171E-17 ) ) ;
#18255=CARTESIAN_POINT ( 'NONE',  ( -12.46703292824872733, -22.22728633158356359, 21.65063509461101177 ) ) ;
#18256=VECTOR ( 'NONE', #16271, 1000.000000000000000 ) ;
#18260=ORIENTED_EDGE ( 'NONE', *, *, #1223, .T. ) ;
#18261=DIRECTION ( 'NONE',  ( -0.1566598588826321192, 0.9876526153536342445, 7.798540720466730171E-17 ) ) ;
#18262=FACE_BOUND ( 'NONE', #18211, .T. ) ;
#18263=VECTOR ( 'NONE', #11652, 1000.000000000000000 ) ;
#18264=DIRECTION ( 'NONE',  ( -0.1566598588826321192, 0.9876526153536342445, 7.798540720466730171E-17 ) ) ;
#18265=VECTOR ( 'NONE', #8582, 1000.000000000000000 ) ;
#18266=DIRECTION ( 'NONE',  ( 0.000000000000000000, 0.000000000000000000, 1.000000000000000000 ) ) ;
#18267=DIRECTION ( 'NONE',  ( -0.1566598588826321192, 0.9876526153536342445, 7.798540720466730171E-17 ) ) ;
#18268=ORIENTED_EDGE ( 'NONE', *, *, #6465, .T. ) ;
#18269=VECTOR ( 'NONE', #15035, 1000.000000000000000 ) ;
#18270=DIRECTION ( 'NONE',  ( 0.000000000000000000, 0.000000000000000000, 1.000000000000000000 ) ) ;
#18272=CARTESIAN_POINT ( 'NONE',  ( -32.50955822205765600, -20.34389050302675628, 17.32050807568881723 ) ) ;
#18274=ORIENTED_EDGE ( 'NONE', *, *, #14993, .T. ) ;
#18275=CARTESIAN_POINT ( 'NONE',  ( -64.60826822105063627, -25.43533591671227256, -12.99038105676658006 ) ) ;
#18276=FACE_OUTER_BOUND ( 'NONE', #778, .T. ) ;
#18277=EDGE_CURVE ( 'NONE', #7282, #18001, #12931, .T. ) ;
#18278=CARTESIAN_POINT ( 'NONE',  ( -7.818242838216901802, -16.42739403096095074, -17.32050807568878170 ) ) ;
#18279=CIRCLE ( 'NONE', #14595, 1.500000000000000888 ) ;
#18280=ORIENTED_EDGE ( 'NONE', *, *, #5464, .T. ) ;
#18281=EDGE_LOOP ( 'NONE', ( #2516, #6537, #12712, #10410 ) ) ;
#18282=CYLINDRICAL_SURFACE ( 'NONE', #16394, 1.500000000000001554 ) ;
#18283=EDGE_CURVE ( 'NONE', #14582, #356, #10200, .T. ) ;
#18284=DIRECTION ( 'NONE',  ( -0.1566598588826321192, 0.9876526153536342445, 7.798540720466731404E-17 ) ) ;
#18287=AXIS2_PLACEMENT_3D ( 'NONE', #15593, #2617, #9907 ) ;
#18288=CARTESIAN_POINT ( 'NONE',  ( -42.09661138885763876, -26.92708209806250608, -21.65063509461098334 ) ) ;
#18289=DIRECTION ( 'NONE',  ( 0.000000000000000000, 0.000000000000000000, 1.000000000000000000 ) ) ;
#18292=LINE ( 'NONE', #9807, #16654 ) ;
#18293=CARTESIAN_POINT ( 'NONE',  ( -3.578159390066044665, -20.81734760163988440, -8.660254037844383745 ) ) ;
#18294=DIRECTION ( 'NONE',  ( -0.9876526153536336894, -0.1566598588826350336, 0.000000000000000000 ) ) ;
#18295=DIRECTION ( 'NONE',  ( -0.1566598588826321192, 0.9876526153536342445, 7.798540720466730171E-17 ) ) ;
#18297=ORIENTED_EDGE ( 'NONE', *, *, #14004, .T. ) ;
#18298=AXIS2_PLACEMENT_3D ( 'NONE', #9563, #10872, #762 ) ;
#18299=FACE_BOUND ( 'NONE', #7413, .T. ) ;
#18300=LINE ( 'NONE', #2318, #12103 ) ;
#18301=VERTEX_POINT ( 'NONE', #5107 ) ;
#18303=CARTESIAN_POINT ( 'NONE',  ( -10.78120068427780964, -16.89737360760884144, -8.660254037844380193 ) ) ;
#18304=CARTESIAN_POINT ( 'NONE',  ( -21.64537945316773460, -18.62063205531779886, 21.65063509461101532 ) ) ;
#18305=EDGE_CURVE ( 'NONE', #16372, #8304, #13848, .T. ) ;
#18306=CARTESIAN_POINT ( 'NONE',  ( -41.56315007100294423, -84.54793360496933019, 21.65063509461101532 ) ) ;
#18307=DIRECTION ( 'NONE',  ( -0.1566598588826321192, 0.9876526153536342445, 7.798540720466730171E-17 ) ) ;
#18308=ORIENTED_EDGE ( 'NONE', *, *, #12332, .T. ) ;
#18309=CYLINDRICAL_SURFACE ( 'NONE', #13321, 1.500000000000001554 ) ;
#18310=CIRCLE ( 'NONE', #12190, 1.499999999999999556 ) ;
#18311=DIRECTION ( 'NONE',  ( -0.000000000000000000, -0.000000000000000000, -1.000000000000000000 ) ) ;
#18313=ORIENTED_EDGE ( 'NONE', *, *, #12052, .F. ) ;
#18314=CARTESIAN_POINT ( 'NONE',  ( -75.96627329761737712, -27.23692429386254332, 12.99038105676661736 ) ) ;
#18315=SURFACE_SIDE_STYLE ('',( #15516 ) ) ;
#18316=EDGE_CURVE ( 'NONE', #15072, #16032, #15668, .T. ) ;
#18317=CARTESIAN_POINT ( 'NONE',  ( -70.04035760549561473, -26.29696514056675483, 17.32050807568881723 ) ) ;
#18318=ORIENTED_EDGE ( 'NONE', *, *, #10416, .T. ) ;
#18319=CARTESIAN_POINT ( 'NONE',  ( -46.50141314777110324, -85.33123289938248490, 12.99038105676661203 ) ) ;
#18320=VERTEX_POINT ( 'NONE', #16214 ) ;
#18321=DIRECTION ( 'NONE',  ( -0.1566598588826321192, 0.9876526153536342445, 7.798540720466731404E-17 ) ) ;
#18322=CARTESIAN_POINT ( 'NONE',  ( -47.32434745236209750, -22.69378838626623107, 17.32050807568881723 ) ) ;
#18323=DIRECTION ( 'NONE',  ( -0.9876526153536344665, -0.1566598588826304539, 0.000000000000000000 ) ) ;
#18324=EDGE_LOOP ( 'NONE', ( #11539, #10914 ) ) ;
#18325=ORIENTED_EDGE ( 'NONE', *, *, #14558, .T. ) ;
#18326=DIRECTION ( 'NONE',  ( -0.1566598588826321192, 0.9876526153536342445, 7.798540720466731404E-17 ) ) ;
#18327=CIRCLE ( 'NONE', #6179, 1.500000000000000444 ) ;
#18328=ORIENTED_EDGE ( 'NONE', *, *, #15531, .F. ) ;
#18329=EDGE_LOOP ( 'NONE', ( #15470, #4449 ) ) ;
#18330=CARTESIAN_POINT ( 'NONE',  ( -15.92381708198642798, -22.77559583767277473, -12.99038105676658006 ) ) ;
#18331=EDGE_CURVE ( 'NONE', #17378, #5203, #14770, .T. ) ;
#18333=DIRECTION ( 'NONE',  ( -0.1566598588826321192, 0.9876526153536342445, 7.798540720466731404E-17 ) ) ;
#18334=ORIENTED_EDGE ( 'NONE', *, *, #4622, .F. ) ;
#18336=FACE_OUTER_BOUND ( 'NONE', #2993, .T. ) ;
#18338=DIRECTION ( 'NONE',  ( -0.1566598588826321747, 0.9876526153536343555, 0.000000000000000000 ) ) ;
#18339=DIRECTION ( 'NONE',  ( -0.9876526153536341335, -0.1566598588826327021, 0.000000000000000000 ) ) ;
#18341=DIRECTION ( 'NONE',  ( 0.000000000000000000, 0.000000000000000000, 1.000000000000000000 ) ) ;
#18343=FACE_OUTER_BOUND ( 'NONE', #4722, .T. ) ;
#18344=EDGE_CURVE ( 'NONE', #5655, #16506, #16287, .T. ) ;
#18346=CYLINDRICAL_SURFACE ( 'NONE', #3493, 1.500000000000000666 ) ;
#18347=DIRECTION ( 'NONE',  ( -0.1566598588826321192, 0.9876526153536342445, 7.798540720466731404E-17 ) ) ;
#18348=DIRECTION ( 'NONE',  ( -0.1566598588826321192, 0.9876526153536342445, 7.798540720466730171E-17 ) ) ;
#18349=ADVANCED_FACE ( 'NONE', ( #15063 ), #14974, .F. ) ;
#18350=ORIENTED_EDGE ( 'NONE', *, *, #14564, .T. ) ;
#18351=FACE_OUTER_BOUND ( 'NONE', #3111, .T. ) ;
#18352=FACE_BOUND ( 'NONE', #5586, .T. ) ;
#18353=EDGE_CURVE ( 'NONE', #5886, #1028, #9622, .T. ) ;
#18354=ADVANCED_FACE ( 'NONE', ( #6374 ), #13718, .F. ) ;
#18355=DIRECTION ( 'NONE',  ( -0.9876526153536344665, -0.1566598588826304539, 0.000000000000000000 ) ) ;
#18356=CIRCLE ( 'NONE', #8630, 1.500000000000000888 ) ;
#18357=ORIENTED_EDGE ( 'NONE', *, *, #16117, .T. ) ;
#18359=EDGE_CURVE ( 'NONE', #7684, #3359, #1754, .T. ) ;
#18360=FACE_OUTER_BOUND ( 'NONE', #11934, .T. ) ;
#18361=LINE ( 'NONE', #5332, #10865 ) ;
#18362=CARTESIAN_POINT ( 'NONE',  ( -42.55080268635659735, -84.70459346385193555, -8.660254037844385522 ) ) ;
#18363=DIRECTION ( 'NONE',  ( -0.1566598588826321747, 0.9876526153536343555, 0.000000000000000000 ) ) ;
#18364=ORIENTED_EDGE ( 'NONE', *, *, #434, .T. ) ;
#18366=AXIS2_PLACEMENT_3D ( 'NONE', #6794, #12626, #1110 ) ;
#18368=ORIENTED_EDGE ( 'NONE', *, *, #7708, .T. ) ;
#18369=ORIENTED_EDGE ( 'NONE', *, *, #9202, .F. ) ;
#18370=DIRECTION ( 'NONE',  ( -0.1566598588826321192, 0.9876526153536342445, 7.798540720466730171E-17 ) ) ;
#18373=DIRECTION ( 'NONE',  ( -0.1566598588826321192, 0.9876526153536342445, 7.798540720466730171E-17 ) ) ;
#18376=FACE_BOUND ( 'NONE', #6995, .T. ) ;
#18377=CARTESIAN_POINT ( 'NONE',  ( -57.36559191666103175, -87.05449134709142811, 1.443110928631665584E-14 ) ) ;
#18380=ADVANCED_FACE ( 'NONE', ( #18042 ), #4918, .F. ) ;
#18381=ORIENTED_EDGE ( 'NONE', *, *, #11487, .F. ) ;
#18384=DIRECTION ( 'NONE',  ( -0.1566598588826321192, 0.9876526153536342445, 7.798540720466731404E-17 ) ) ;
#18385=VERTEX_POINT ( 'NONE', #3577 ) ;
#18387=LINE ( 'NONE', #5361, #16840 ) ;
#18390=FACE_BOUND ( 'NONE', #2230, .T. ) ;
#18392=VECTOR ( 'NONE', #10522, 1000.000000000000000 ) ;
#18393=VERTEX_POINT ( 'NONE', #6550 ) ;
#18394=ORIENTED_EDGE ( 'NONE', *, *, #10215, .T. ) ;
#18396=VECTOR ( 'NONE', #14404, 1000.000000000000000 ) ;
#18398=FACE_OUTER_BOUND ( 'NONE', #213, .T. ) ;
#18399=CARTESIAN_POINT ( 'NONE',  ( -63.78533391645962780, -88.07278042982854060, 8.660254037844412167 ) ) ;
#18400=ORIENTED_EDGE ( 'NONE', *, *, #14709, .F. ) ;
#18401=CARTESIAN_POINT ( 'NONE',  ( -37.15834831208948685, -26.14378280364935137, 12.99038105676661736 ) ) ;
#18402=AXIS2_PLACEMENT_3D ( 'NONE', #16507, #14624, #1821 ) ;
#18403=DIRECTION ( 'NONE',  ( -0.1566598588826321192, 0.9876526153536342445, 7.798540720466731404E-17 ) ) ;
#18404=DIRECTION ( 'NONE',  ( -0.9876526153536336894, -0.1566598588826349503, 0.000000000000000000 ) ) ;
#18406=ADVANCED_FACE ( 'NONE', ( #10614 ), #16417, .F. ) ;
#18407=ORIENTED_EDGE ( 'NONE', *, *, #13101, .T. ) ;
#18409=EDGE_CURVE ( 'NONE', #4280, #2469, #14163, .T. ) ;
#18410=CYLINDRICAL_SURFACE ( 'NONE', #2091, 1.500000000000000666 ) ;
#18412=ORIENTED_EDGE ( 'NONE', *, *, #11076, .F. ) ;
#18413=DIRECTION ( 'NONE',  ( -0.1566598588826321747, 0.9876526153536343555, 0.000000000000000000 ) ) ;
#18414=ORIENTED_EDGE ( 'NONE', *, *, #7985, .T. ) ;
#18416=VERTEX_POINT ( 'NONE', #12292 ) ;
#18417=ORIENTED_EDGE ( 'NONE', *, *, #11211, .F. ) ;
#18419=ADVANCED_FACE ( 'NONE', ( #9671 ), #8431, .F. ) ;
#18420=DIRECTION ( 'NONE',  ( -0.9876526153536341335, -0.1566598588826327021, 0.000000000000000000 ) ) ;
#18421=CYLINDRICAL_SURFACE ( 'NONE', #4799, 1.500000000000000888 ) ;
#18422=ORIENTED_EDGE ( 'NONE', *, *, #4677, .T. ) ;
#18424=EDGE_LOOP ( 'NONE', ( #14121, #7552 ) ) ;
#18425=AXIS2_PLACEMENT_3D ( 'NONE', #10132, #15839, #14230 ) ;
#18426=CARTESIAN_POINT ( 'NONE',  ( -0.4108482230646762212, -15.25244508934120802, -21.65063509461098334 ) ) ;
#18433=DIRECTION ( 'NONE',  ( -0.1566598588826321192, 0.9876526153536342445, 7.798540720466731404E-17 ) ) ;
#18434=CARTESIAN_POINT ( 'NONE',  ( -49.50400600400985951, -28.10203103968224170, -8.660254037844380193 ) ) ;
#18435=AXIS2_PLACEMENT_3D ( 'NONE', #15132, #16666, #740 ) ;
#18436=DIRECTION ( 'NONE',  ( -0.9876526153536336894, -0.1566598588826350336, 0.000000000000000000 ) ) ;
#18437=DIRECTION ( 'NONE',  ( -0.1566598588826321192, 0.9876526153536342445, 7.798540720466730171E-17 ) ) ;
#18438=CIRCLE ( 'NONE', #5675, 1.499999999999999556 ) ;
#18439=CARTESIAN_POINT ( 'NONE',  ( -3.044698072211382112, -78.43819910854666944, 17.32050807568880657 ) ) ;
#18440=ORIENTED_EDGE ( 'NONE', *, *, #8730, .T. ) ;
#18441=DIRECTION ( 'NONE',  ( -0.1566598588826321192, 0.9876526153536342445, 7.798540720466731404E-17 ) ) ;
#18443=EDGE_CURVE ( 'NONE', #2583, #8675, #18139, .T. ) ;
#18447=EDGE_LOOP ( 'NONE', ( #14319, #185, #18149, #1890 ) ) ;
#18448=EDGE_CURVE ( 'NONE', #7294, #14450, #14464, .T. ) ;
#18449=ORIENTED_EDGE ( 'NONE', *, *, #17291, .F. ) ;
#18450=DIRECTION ( 'NONE',  ( -0.9876526153536336894, -0.1566598588826349503, 0.000000000000000000 ) ) ;
#18451=CIRCLE ( 'NONE', #8397, 1.500000000000000888 ) ;
#18452=FACE_BOUND ( 'NONE', #16072, .T. ) ;
#18455=ORIENTED_EDGE ( 'NONE', *, *, #2607, .F. ) ;
#18456=ORIENTED_EDGE ( 'NONE', *, *, #543, .F. ) ;
#18457=DIRECTION ( 'NONE',  ( -0.1566598588826321192, 0.9876526153536342445, 7.798540720466730171E-17 ) ) ;
#18458=AXIS2_PLACEMENT_3D ( 'NONE', #14858, #7674, #2061 ) ;
#18459=CARTESIAN_POINT ( 'NONE',  ( -73.49714175923330117, -26.84527464665595886, 1.908195823574487804E-14 ) ) ;
#18460=CARTESIAN_POINT ( 'NONE',  ( -37.94164760650263446, -21.20551972688122078, 4.330127018922218518 ) ) ;
#18462=EDGE_CURVE ( 'NONE', #3287, #6534, #15977, .T. ) ;
#18463=CIRCLE ( 'NONE', #16918, 1.500000000000000888 ) ;
#18464=CIRCLE ( 'NONE', #13897, 1.500000000000000444 ) ;
#18466=EDGE_CURVE ( 'NONE', #13075, #11927, #8716, .T. ) ;
#18468=EDGE_CURVE ( 'NONE', #12073, #2, #240, .T. ) ;
#18469=CARTESIAN_POINT ( 'NONE',  ( -35.67686938905902849, -25.90879301532540779, 21.65063509461101887 ) ) ;
#18470=EDGE_LOOP ( 'NONE', ( #18260, #7290 ) ) ;
#18471=ORIENTED_EDGE ( 'NONE', *, *, #9439, .T. ) ;
#18473=ORIENTED_EDGE ( 'NONE', *, *, #12171, .F. ) ;
#18474=ORIENTED_EDGE ( 'NONE', *, *, #13328, .F. ) ;
#18475=CARTESIAN_POINT ( 'NONE',  ( -60.32854976272193426, -87.52447092373932946, -8.660254037844385522 ) ) ;
#18476=VECTOR ( 'NONE', #13295, 1000.000000000000000 ) ;
#18477=CIRCLE ( 'NONE', #16932, 1.500000000000000888 ) ;
#18478=VECTOR ( 'NONE', #3703, 1000.000000000000000 ) ;
#18481=DIRECTION ( 'NONE',  ( -0.1566598588826321747, 0.9876526153536343555, 0.000000000000000000 ) ) ;
#18482=CARTESIAN_POINT ( 'NONE',  ( 1.399738696879940791, -77.73322974357483872, 21.65063509461100821 ) ) ;
#18483=EDGE_LOOP ( 'NONE', ( #12432, #8578 ) ) ;
#18485=CARTESIAN_POINT ( 'NONE',  ( -24.11451099155181055, -19.01228170252437266, -8.660254037844380193 ) ) ;
#18486=DIRECTION ( 'NONE',  ( -0.1566598588826321192, 0.9876526153536342445, 7.798540720466730171E-17 ) ) ;
#18489=EDGE_LOOP ( 'NONE', ( #17023, #7779, #3265, #124 ) ) ;
#18490=DIRECTION ( 'NONE',  ( 0.000000000000000000, 0.000000000000000000, 1.000000000000000000 ) ) ;
#18491=CYLINDRICAL_SURFACE ( 'NONE', #13947, 1.500000000000001554 ) ;
#18492=CIRCLE ( 'NONE', #7842, 1.500000000000000444 ) ;
#18493=EDGE_LOOP ( 'NONE', ( #10677, #16836, #1376, #15863 ) ) ;
#18497=ORIENTED_EDGE ( 'NONE', *, *, #242, .F. ) ;
#18498=ORIENTED_EDGE ( 'NONE', *, *, #708, .F. ) ;
#18499=CARTESIAN_POINT ( 'NONE',  ( -25.80034323552273179, -24.34219442649909126, -21.65063509461098334 ) ) ;
#18500=ORIENTED_EDGE ( 'NONE', *, *, #17349, .T. ) ;
#18501=DIRECTION ( 'NONE',  ( -0.1566598588826321192, 0.9876526153536342445, 7.798540720466730171E-17 ) ) ;
#18502=ORIENTED_EDGE ( 'NONE', *, *, #13085, .F. ) ;
#18503=CIRCLE ( 'NONE', #271, 1.500000000000000888 ) ;
#18504=DIRECTION ( 'NONE',  ( 0.000000000000000000, 0.000000000000000000, 1.000000000000000000 ) ) ;
#18505=DIRECTION ( 'NONE',  ( -0.1566598588826321192, 0.9876526153536342445, 7.798540720466730171E-17 ) ) ;
#18506=AXIS2_PLACEMENT_3D ( 'NONE', #3865, #9684, #15459 ) ;
#18507=CARTESIAN_POINT ( 'NONE',  ( -32.22008523532133495, -25.36048350923618955, -21.65063509461098334 ) ) ;
#18509=AXIS2_PLACEMENT_3D ( 'NONE', #2960, #10078, #17493 ) ;
#18510=CARTESIAN_POINT ( 'NONE',  ( -5.349111299832828514, -16.03574438375436984, -21.65063509461098334 ) ) ;
#18511=AXIS2_PLACEMENT_3D ( 'NONE', #4957, #14591, #8978 ) ;
#18513=DIRECTION ( 'NONE',  ( -0.9876526153536336894, -0.1566598588826349503, 0.000000000000000000 ) ) ;
#18515=VERTEX_POINT ( 'NONE', #5215 ) ;
#18516=DIRECTION ( 'NONE',  ( -0.1566598588826321192, 0.9876526153536342445, 7.798540720466731404E-17 ) ) ;
#18517=DIRECTION ( 'NONE',  ( 0.000000000000000000, 0.000000000000000000, 1.000000000000000000 ) ) ;
#18518=EDGE_LOOP ( 'NONE', ( #549, #17069, #9837, #14681 ) ) ;
#18521=EDGE_LOOP ( 'NONE', ( #1482, #8303 ) ) ;
#18522=EDGE_LOOP ( 'NONE', ( #4318, #146 ) ) ;
#18523=EDGE_CURVE ( 'NONE', #6427, #15929, #17079, .T. ) ;
#18524=CIRCLE ( 'NONE', #11181, 1.499999999999999556 ) ;
#18525=EDGE_CURVE ( 'NONE', #3315, #1682, #9924, .T. ) ;
#18526=CARTESIAN_POINT ( 'NONE',  ( -71.23236354178969520, -31.54854793510013877, 1.887572821959364500E-14 ) ) ;
#18530=CARTESIAN_POINT ( 'NONE',  ( -11.93357161039406300, -79.84813783849035929, -12.99038105676658539 ) ) ;
#18531=CARTESIAN_POINT ( 'NONE',  ( -75.96627329761737712, -27.23692429386253622, -4.330127018922180326 ) ) ;
#18532=AXIS2_PLACEMENT_3D ( 'NONE', #11696, #15896, #14477 ) ;
#18533=CYLINDRICAL_SURFACE ( 'NONE', #17854, 1.500000000000001554 ) ;
#18535=FACE_BOUND ( 'NONE', #9919, .T. ) ;
#18537=CARTESIAN_POINT ( 'NONE',  ( -56.37793930130741415, -86.89783148820879433, -12.99038105676658539 ) ) ;
#18538=CIRCLE ( 'NONE', #12094, 1.500000000000000888 ) ;
#18539=ORIENTED_EDGE ( 'NONE', *, *, #2080, .F. ) ;
#18540=CIRCLE ( 'NONE', #8204, 1.499999999999999556 ) ;
#18541=EDGE_LOOP ( 'NONE', ( #6957, #18313, #11816, #203 ) ) ;
#18542=DIRECTION ( 'NONE',  ( -0.9876526153536341335, -0.1566598588826327021, 0.000000000000000000 ) ) ;
#18544=ORIENTED_EDGE ( 'NONE', *, *, #1119, .F. ) ;
#18545=ORIENTED_EDGE ( 'NONE', *, *, #17436, .T. ) ;
#18546=CIRCLE ( 'NONE', #11801, 1.500000000000000888 ) ;
#18548=CIRCLE ( 'NONE', #10001, 1.500000000000000888 ) ;
#18549=DIRECTION ( 'NONE',  ( -0.1566598588826321192, 0.9876526153536342445, 7.798540720466731404E-17 ) ) ;
#18550=ADVANCED_FACE ( 'NONE', ( #2641 ), #1156, .F. ) ;
#18551=CYLINDRICAL_SURFACE ( 'NONE', #6456, 1.500000000000001554 ) ;
#18552=ORIENTED_EDGE ( 'NONE', *, *, #14304, .T. ) ;
#18553=CIRCLE ( 'NONE', #15773, 1.500000000000000888 ) ;
#18554=LINE ( 'NONE', #14132, #9663 ) ;
#18556=EDGE_LOOP ( 'NONE', ( #11336, #12974, #15043, #3763 ) ) ;
#18557=EDGE_CURVE ( 'NONE', #13791, #6631, #16594, .T. ) ;
#18559=CARTESIAN_POINT ( 'NONE',  ( -51.97313754239392125, -28.49368068688881550, 21.65063509461101887 ) ) ;
#18560=CARTESIAN_POINT ( 'NONE',  ( -39.09401853261890381, -84.15628395776272441, -17.32050807568878525 ) ) ;
#18562=EDGE_LOOP ( 'NONE', ( #5956, #17133, #8418, #3288 ) ) ;
#18563=DIRECTION ( 'NONE',  ( -0.9876526153536336894, -0.1566598588826349503, 0.000000000000000000 ) ) ;
#18564=AXIS2_PLACEMENT_3D ( 'NONE', #2743, #8536, #11343 ) ;
#18565=ORIENTED_EDGE ( 'NONE', *, *, #13149, .F. ) ;
#18566=ORIENTED_EDGE ( 'NONE', *, *, #5486, .F. ) ;
#18567=AXIS2_PLACEMENT_3D ( 'NONE', #15382, #15202, #7996 ) ;
#18568=ORIENTED_EDGE ( 'NONE', *, *, #16916, .F. ) ;
#18569=ORIENTED_EDGE ( 'NONE', *, *, #18707, .T. ) ;
#18571=ORIENTED_EDGE ( 'NONE', *, *, #8209, .T. ) ;
#18572=ORIENTED_EDGE ( 'NONE', *, *, #15950, .F. ) ;
#18576=EDGE_CURVE ( 'NONE', #9820, #17569, #12670, .T. ) ;
#18577=AXIS2_PLACEMENT_3D ( 'NONE', #5214, #14016, #1248 ) ;
#18579=CARTESIAN_POINT ( 'NONE',  ( -75.18297400320422241, -32.17518737063066681, -21.65063509461098334 ) ) ;
#18581=EDGE_CURVE ( 'NONE', #2601, #15004, #4172, .T. ) ;
#18582=AXIS2_PLACEMENT_3D ( 'NONE', #7589, #6263, #11995 ) ;
#18583=ORIENTED_EDGE ( 'NONE', *, *, #14732, .T. ) ;
#18584=CYLINDRICAL_SURFACE ( 'NONE', #15735, 1.500000000000001554 ) ;
#18585=CARTESIAN_POINT ( 'NONE',  ( -21.81009776393036503, -81.41473642731669713, 21.65063509461101532 ) ) ;
#18587=COLOUR_RGB ( '', 0.31764706, 0.68627451, 0.89019608) ;
#18588=CARTESIAN_POINT ( 'NONE',  ( -13.25033222266188560, -17.28902325481542235, 12.99038105676661381 ) ) ;
#18589=ORIENTED_EDGE ( 'NONE', *, *, #10987, .T. ) ;
#18590=VERTEX_POINT ( 'NONE', #9931 ) ;
#18591=CARTESIAN_POINT ( 'NONE',  ( 1.360103686702108128, -20.03404830722672259, 17.32050807568881012 ) ) ;
#18593=CIRCLE ( 'NONE', #686, 1.500000000000000888 ) ;
#18596=VERTEX_POINT ( 'NONE', #173 ) ;
#18597=CARTESIAN_POINT ( 'NONE',  ( -51.43967622453926936, -86.11453219379562540, -12.99038105676658539 ) ) ;
#18600=EDGE_CURVE ( 'NONE', #11742, #9953, #1518, .T. ) ;
#18602=DIRECTION ( 'NONE',  ( -0.1566598588826321192, 0.9876526153536342445, 7.798540720466730171E-17 ) ) ;
#18603=EDGE_CURVE ( 'NONE', #5396, #13454, #4428, .T. ) ;
#18604=CYLINDRICAL_SURFACE ( 'NONE', #10628, 1.500000000000001554 ) ;
#18605=CARTESIAN_POINT ( 'NONE',  ( -42.09661138885763165, -26.92708209806250608, 4.330127018922217630 ) ) ;
#18606=CARTESIAN_POINT ( 'NONE',  ( -27.57129514528951120, -19.56059120861358736, -8.660254037844380193 ) ) ;
#18608=AXIS2_PLACEMENT_3D ( 'NONE', #412, #18055, #12025 ) ;
#18609=CYLINDRICAL_SURFACE ( 'NONE', #3877, 1.500000000000001554 ) ;
#18611=DIRECTION ( 'NONE',  ( -0.1566598588826321747, 0.9876526153536343555, 0.000000000000000000 ) ) ;
#18612=CARTESIAN_POINT ( 'NONE',  ( -41.39843176024032800, -21.75382923297043192, 4.330127018922218518 ) ) ;
#18615=DIRECTION ( 'NONE',  ( -0.1566598588826321192, 0.9876526153536342445, 7.798540720466731404E-17 ) ) ;
#18617=ORIENTED_EDGE ( 'NONE', *, *, #10015, .F. ) ;
#18618=ORIENTED_EDGE ( 'NONE', *, *, #13364, .F. ) ;
#18619=VERTEX_POINT ( 'NONE', #8537 ) ;
#18620=VERTEX_POINT ( 'NONE', #14488 ) ;
#18621=CIRCLE ( 'NONE', #7665, 1.500000000000000888 ) ;
#18623=ORIENTED_EDGE ( 'NONE', *, *, #11715, .T. ) ;
#18624=CARTESIAN_POINT ( 'NONE',  ( -11.76885329963143079, -17.05403346649147878, 12.99038105676661381 ) ) ;
#18625=CARTESIAN_POINT ( 'NONE',  ( -50.28730529842301422, -23.16376796291411111, -8.660254037844380193 ) ) ;
#18626=DIRECTION ( 'NONE',  ( -0.9876526153536336894, -0.1566598588826349503, 0.000000000000000000 ) ) ;
#18627=DIRECTION ( 'NONE',  ( -0.9876526153536336894, -0.1566598588826349503, 0.000000000000000000 ) ) ;
#18628=DIRECTION ( 'NONE',  ( -0.1566598588826321747, 0.9876526153536343555, 0.000000000000000000 ) ) ;
#18629=CYLINDRICAL_SURFACE ( 'NONE', #17942, 1.500000000000001554 ) ;
#18630=CARTESIAN_POINT ( 'NONE',  ( -39.91695283720989096, -21.51883944464648124, -12.99038105676658006 ) ) ;
#18631=FACE_BOUND ( 'NONE', #1167, .T. ) ;
#18634=DIRECTION ( 'NONE',  ( -0.1566598588826321192, 0.9876526153536342445, 7.798540720466730171E-17 ) ) ;
#18636=DIRECTION ( 'NONE',  ( 0.000000000000000000, 0.000000000000000000, 1.000000000000000000 ) ) ;
#18637=ORIENTED_EDGE ( 'NONE', *, *, #13971, .F. ) ;
#18638=ORIENTED_EDGE ( 'NONE', *, *, #8154, .T. ) ;
#18639=CARTESIAN_POINT ( 'NONE',  ( -47.32434745236211171, -22.69378838626622041, -8.660254037844380193 ) ) ;
#18640=ORIENTED_EDGE ( 'NONE', *, *, #4028, .T. ) ;
#18641=ORIENTED_EDGE ( 'NONE', *, *, #16184, .F. ) ;
#18642=CARTESIAN_POINT ( 'NONE',  ( 1.360103686702108128, -20.03404830722672259, -17.32050807568878170 ) ) ;
#18643=EDGE_LOOP ( 'NONE', ( #12492, #4752, #9342, #10402, #7152, #7006, #1713, #1073, #14657, #14707, #11382, #1635 ) ) ;
#18644=CARTESIAN_POINT ( 'NONE',  ( -6.047290928450125946, -21.20899724884646531, 12.99038105676661026 ) ) ;
#18645=DIRECTION ( 'NONE',  ( -0.1566598588826321192, 0.9876526153536342445, 7.798540720466731404E-17 ) ) ;
#18646=EDGE_LOOP ( 'NONE', ( #16757, #16505, #4188, #13872 ) ) ;
#18648=FACE_BOUND ( 'NONE', #9947, .T. ) ;
#18649=ADVANCED_FACE ( 'NONE', ( #14400 ), #17163, .F. ) ;
#18650=LINE ( 'NONE', #11186, #6854 ) ;
#18652=CARTESIAN_POINT ( 'NONE',  ( -63.78533391645962780, -88.07278042982852639, -8.660254037844385522 ) ) ;
#18654=CYLINDRICAL_SURFACE ( 'NONE', #5733, 2.000000000000000000 ) ;
#18655=EDGE_CURVE ( 'NONE', #14342, #5230, #3011, .T. ) ;
#18656=ORIENTED_EDGE ( 'NONE', *, *, #3962, .F. ) ;
#18657=ORIENTED_EDGE ( 'NONE', *, *, #3170, .F. ) ;
#18658=ORIENTED_EDGE ( 'NONE', *, *, #6746, .T. ) ;
#18659=DIRECTION ( 'NONE',  ( 0.000000000000000000, 0.000000000000000000, 1.000000000000000000 ) ) ;
#18660=EDGE_LOOP ( 'NONE', ( #402, #10322, #6122, #10713 ) ) ;
#18661=ORIENTED_EDGE ( 'NONE', *, *, #14159, .T. ) ;
#18662=CIRCLE ( 'NONE', #17112, 1.500000000000000888 ) ;
#18663=FACE_BOUND ( 'NONE', #13908, .T. ) ;
#18665=CARTESIAN_POINT ( 'NONE',  ( -56.21322099054479082, -24.10372711620989961, -12.99038105676658006 ) ) ;
#18666=FACE_OUTER_BOUND ( 'NONE', #8441, .T. ) ;
#18668=EDGE_LOOP ( 'NONE', ( #14251, #12816 ) ) ;
#18669=CARTESIAN_POINT ( 'NONE',  ( -16.70711637639958269, -17.83733276090463349, -21.65063509461097979 ) ) ;
#18670=CARTESIAN_POINT ( 'NONE',  ( -6.830590222863280658, -16.27073417207831696, 4.330127018922214965 ) ) ;
#18671=CARTESIAN_POINT ( 'NONE',  ( -56.91140061916209447, -29.27697998130198442, -4.330127018922181215 ) ) ;
#18672=CARTESIAN_POINT ( 'NONE',  ( -30.20514499443621759, -82.74634522781903456, -21.65063509461098690 ) ) ;
#18673=VERTEX_POINT ( 'NONE', #12956 ) ;
#18674=EDGE_LOOP ( 'NONE', ( #7617, #14931 ) ) ;
#18675=LINE ( 'NONE', #12737, #16664 ) ;
#18676=FACE_OUTER_BOUND ( 'NONE', #5679, .T. ) ;
#18677=ADVANCED_FACE ( 'NONE', ( #11531 ), #8799, .F. ) ;
#18678=DIRECTION ( 'NONE',  ( -0.1566598588826321192, 0.9876526153536342445, 7.798540720466730171E-17 ) ) ;
#18679=ORIENTED_EDGE ( 'NONE', *, *, #7689, .T. ) ;
#18680=DIRECTION ( 'NONE',  ( -0.1566598588826321192, 0.9876526153536342445, 7.798540720466730171E-17 ) ) ;
#18681=EDGE_CURVE ( 'NONE', #6631, #14196, #18714, .T. ) ;
#18682=EDGE_LOOP ( 'NONE', ( #1951, #2396 ) ) ;
#18683=AXIS2_PLACEMENT_3D ( 'NONE', #11586, #17408, #5643 ) ;
#18685=EDGE_LOOP ( 'NONE', ( #18065, #10890 ) ) ;
#18687=DIRECTION ( 'NONE',  ( -0.1566598588826321192, 0.9876526153536342445, 7.798540720466731404E-17 ) ) ;
#18688=CARTESIAN_POINT ( 'NONE',  ( -55.42992169613161479, -29.04199019297804085, 21.65063509461101887 ) ) ;
#18690=EDGE_LOOP ( 'NONE', ( #10195, #9290 ) ) ;
#18691=CIRCLE ( 'NONE', #11943, 1.500000000000000888 ) ;
#18692=FACE_OUTER_BOUND ( 'NONE', #13805, .T. ) ;
#18693=ORIENTED_EDGE ( 'NONE', *, *, #4150, .F. ) ;
#18694=CARTESIAN_POINT ( 'NONE',  ( -52.92115514756972061, -86.34952198211958319, -21.65063509461098690 ) ) ;
#18696=CARTESIAN_POINT ( 'NONE',  ( -57.89905323451570496, -29.43363984018461466, 17.32050807568881723 ) ) ;
#18697=CYLINDRICAL_SURFACE ( 'NONE', #7592, 1.500000000000001554 ) ;
#18698=AXIS2_PLACEMENT_3D ( 'NONE', #16109, #3104, #8896 ) ;
#18699=DIRECTION ( 'NONE',  ( -0.1566598588826321192, 0.9876526153536342445, 7.798540720466730171E-17 ) ) ;
#18700=ORIENTED_EDGE ( 'NONE', *, *, #12138, .F. ) ;
#18701=EDGE_CURVE ( 'NONE', #3501, #4575, #11131, .T. ) ;
#18702=ADVANCED_FACE ( 'NONE', ( #17543 ), #10307, .F. ) ;
#18703=CARTESIAN_POINT ( 'NONE',  ( -84.16561914167408531, 33.59999999999999432, -24.99999999999999289 ) ) ;
#18704=DIRECTION ( 'NONE',  ( -0.1566598588826321192, 0.9876526153536342445, 7.798540720466731404E-17 ) ) ;
#18705=VERTEX_POINT ( 'NONE', #11434 ) ;
#18706=VERTEX_POINT ( 'NONE', #17273 ) ;
#18707=EDGE_CURVE ( 'NONE', #9998, #11894, #12340, .T. ) ;
#18708=AXIS2_PLACEMENT_3D ( 'NONE', #13452, #6289, #303 ) ;
#18709=FACE_OUTER_BOUND ( 'NONE', #16286, .T. ) ;
#18710=ORIENTED_EDGE ( 'NONE', *, *, #16353, .T. ) ;
#18711=CARTESIAN_POINT ( 'NONE',  ( -11.93357161039406300, -79.84813783849037350, 12.99038105676661203 ) ) ;
#18713=CARTESIAN_POINT ( 'NONE',  ( -4.526176995241833367, -78.67318889687062722, 1.424741226644455312E-14 ) ) ;
#18714=LINE ( 'NONE', #8707, #9937 ) ;
#18715=CARTESIAN_POINT ( 'NONE',  ( -0.5755665338273054932, -78.04654946134009208, 21.65063509461100821 ) ) ;
#18717=CARTESIAN_POINT ( 'NONE',  ( -16.87183468716221313, -80.63143713290352821, -21.65063509461098690 ) ) ;
#18718=CARTESIAN_POINT ( 'NONE',  ( -15.22563745336913144, -17.60234297258068992, -12.99038105676658006 ) ) ;
#18719=ORIENTED_EDGE ( 'NONE', *, *, #5083, .T. ) ;
#18720=EDGE_CURVE ( 'NONE', #10673, #6102, #2375, .T. ) ;
#18722=DIRECTION ( 'NONE',  ( -0.1566598588826321192, 0.9876526153536342445, 7.798540720466730171E-17 ) ) ;
#18723=AXIS2_PLACEMENT_3D ( 'NONE', #10375, #17802, #7825 ) ;
#18724=ORIENTED_EDGE ( 'NONE', *, *, #11185, .F. ) ;
#18725=ORIENTED_EDGE ( 'NONE', *, *, #9241, .F. ) ;
#18726=DIRECTION ( 'NONE',  ( -0.9876526153536341335, -0.1566598588826327021, 0.000000000000000000 ) ) ;
#18727=CIRCLE ( 'NONE', #1440, 1.499999999999999556 ) ;
#18728=DIRECTION ( 'NONE',  ( 0.1566598588826321192, -0.9876526153536342445, -7.798540720466731404E-17 ) ) ;
#18729=AXIS2_PLACEMENT_3D ( 'NONE', #1134, #1232, #1052 ) ;
#18730=CIRCLE ( 'NONE', #13814, 1.500000000000000888 ) ;
#18731=ORIENTED_EDGE ( 'NONE', *, *, #16669, .F. ) ;
#18732=AXIS2_PLACEMENT_3D ( 'NONE', #9890, #10079, #5641 ) ;
#18734=CIRCLE ( 'NONE', #13506, 1.500000000000000888 ) ;
#18735=CYLINDRICAL_SURFACE ( 'NONE', #16063, 1.500000000000001554 ) ;
#18736=DIRECTION ( 'NONE',  ( -0.1566598588826321747, 0.9876526153536343555, 0.000000000000000000 ) ) ;
#18737=DIRECTION ( 'NONE',  ( 0.000000000000000000, 0.000000000000000000, 1.000000000000000000 ) ) ;
#18738=CIRCLE ( 'NONE', #10208, 1.500000000000000888 ) ;
#18739=CARTESIAN_POINT ( 'NONE',  ( -63.78533391645962780, -88.07278042982852639, 1.424741226644455312E-14 ) ) ;
#18740=ORIENTED_EDGE ( 'NONE', *, *, #1830, .F. ) ;
#18743=ORIENTED_EDGE ( 'NONE', *, *, #2404, .F. ) ;
#18745=EDGE_LOOP ( 'NONE', ( #8541, #8448, #17738, #18182 ) ) ;
#18749=AXIS2_PLACEMENT_3D ( 'NONE', #144, #18678, #17503 ) ;
#18750=CARTESIAN_POINT ( 'NONE',  ( -33.20773785067495965, -25.51714336811882688, 17.32050807568881723 ) ) ;
#18751=EDGE_CURVE ( 'NONE', #11320, #5805, #13865, .T. ) ;
#18753=AXIS2_PLACEMENT_3D ( 'NONE', #12274, #17932, #4898 ) ;
#18754=DIRECTION ( 'NONE',  ( 0.000000000000000000, 0.000000000000000000, 1.000000000000000000 ) ) ;
#18756=AXIS2_PLACEMENT_3D ( 'NONE', #723, #17620, #630 ) ;
#18757=CARTESIAN_POINT ( 'NONE',  ( -0.4108482230646692823, -15.25244508934120802, 4.330127018922213189 ) ) ;
#18758=CARTESIAN_POINT ( 'NONE',  ( -81.73462711737164454, 33.01666666666666572, 25.00000000000001421 ) ) ;
#18759=DIRECTION ( 'NONE',  ( 0.000000000000000000, 0.000000000000000000, 1.000000000000000000 ) ) ;
#18760=AXIS2_PLACEMENT_3D ( 'NONE', #12495, #6933, #18339 ) ;
#18761=DIRECTION ( 'NONE',  ( -0.9876526153536341335, -0.1566598588826327021, 0.000000000000000000 ) ) ;
#18766=VECTOR ( 'NONE', #8183, 1000.000000000000000 ) ;
#18768=CARTESIAN_POINT ( 'NONE',  ( -28.26947477390680774, -24.73384407370567217, 17.32050807568881723 ) ) ;
#18769=CIRCLE ( 'NONE', #17530, 1.500000000000000444 ) ;
#18770=AXIS2_PLACEMENT_3D ( 'NONE', #792, #9708, #5428 ) ;
#18771=CARTESIAN_POINT ( 'NONE',  ( -33.00338452973448966, -20.42222043246805185, -21.65063509461098334 ) ) ;
#18772=AXIS2_PLACEMENT_3D ( 'NONE', #13611, #7473, #14759 ) ;
#18773=CARTESIAN_POINT ( 'NONE',  ( -25.76070822534488869, -82.04137586284720385, -17.32050807568878525 ) ) ;
#18774=ADVANCED_FACE ( 'NONE', ( #4973 ), #4895, .F. ) ;
#18775=DIRECTION ( 'NONE',  ( -0.1566598588826321192, 0.9876526153536342445, 7.798540720466731404E-17 ) ) ;
#18777=FACE_OUTER_BOUND ( 'NONE', #4476, .T. ) ;
#18778=AXIS2_PLACEMENT_3D ( 'NONE', #10061, #5825, #11565 ) ;
#18779=DIRECTION ( 'NONE',  ( -0.1566598588826321192, 0.9876526153536342445, 7.798540720466731404E-17 ) ) ;
#18782=AXIS2_PLACEMENT_3D ( 'NONE', #372, #11706, #10309 ) ;
#18783=ORIENTED_EDGE ( 'NONE', *, *, #14564, .F. ) ;
#18785=EDGE_CURVE ( 'NONE', #2879, #13088, #7746, .T. ) ;
#18786=EDGE_LOOP ( 'NONE', ( #5644, #409, #4098, #12793 ) ) ;
#18788=ORIENTED_EDGE ( 'NONE', *, *, #6249, .F. ) ;
#18789=ORIENTED_EDGE ( 'NONE', *, *, #4744, .T. ) ;
#18790=VECTOR ( 'NONE', #7320, 1000.000000000000000 ) ;
#18791=VECTOR ( 'NONE', #9207, 1000.000000000000000 ) ;
#18792=CARTESIAN_POINT ( 'NONE',  ( 3.231158466157545206, -19.73726462726228092, 30.00000000000000000 ) ) ;
#18793=ORIENTED_EDGE ( 'NONE', *, *, #2850, .T. ) ;
#18794=EDGE_CURVE ( 'NONE', #5711, #4998, #12641, .T. ) ;
ENDSEC;
END-ISO-10303-21;
